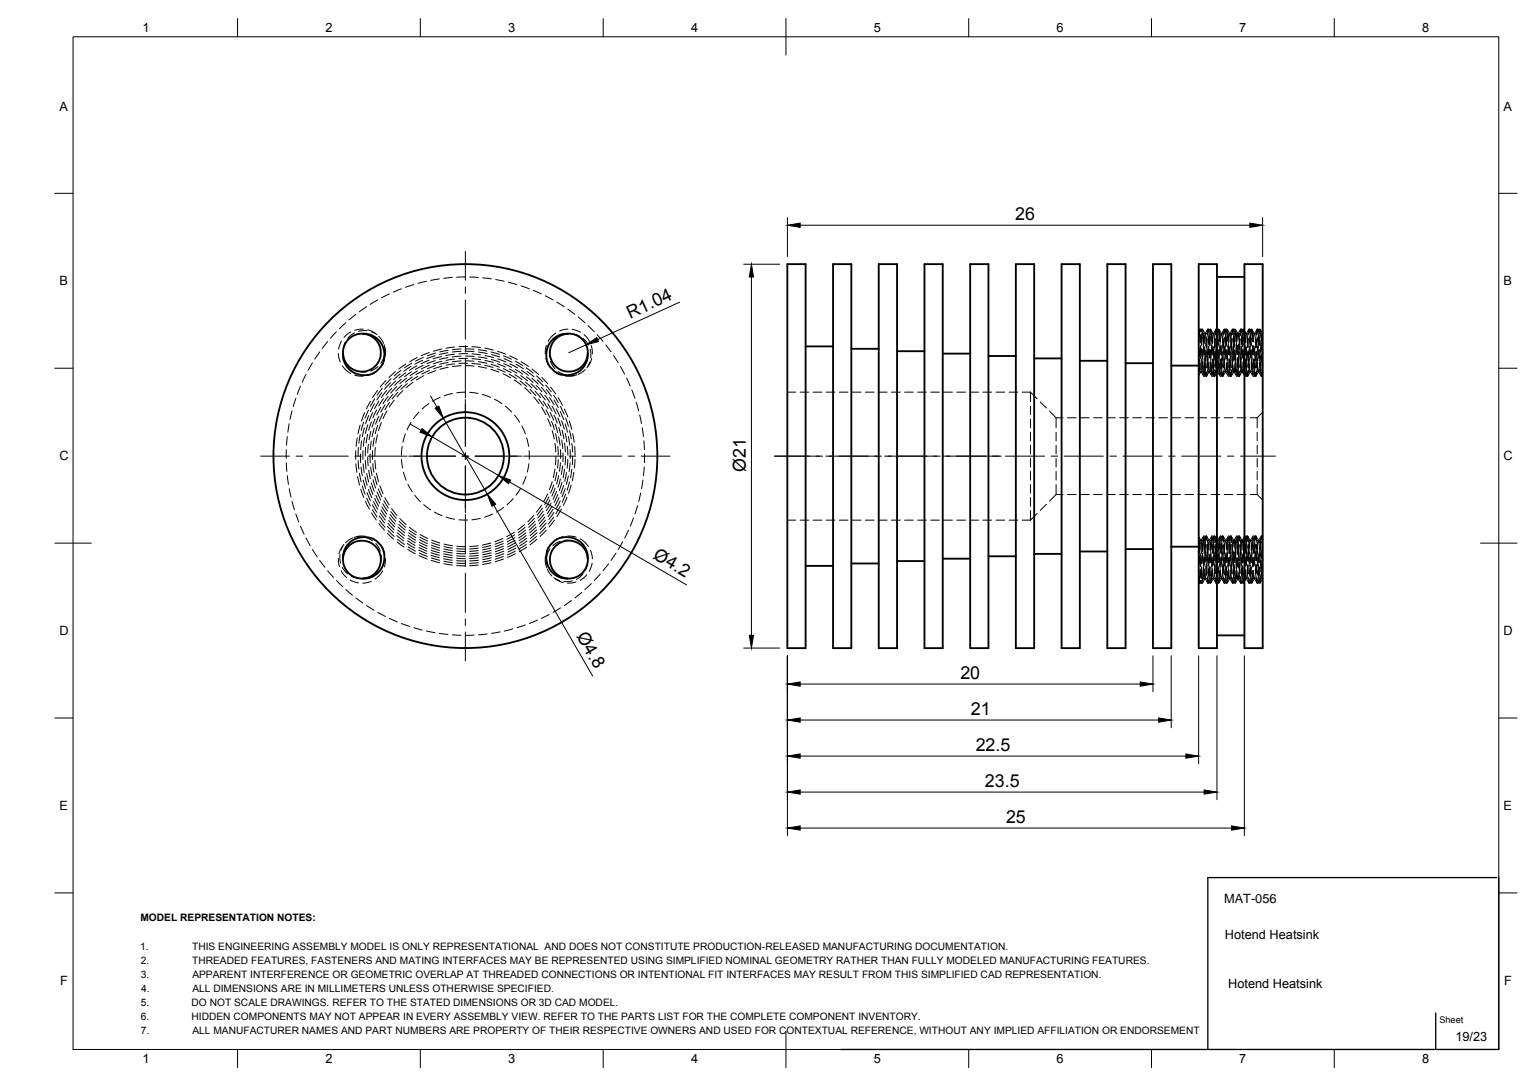
ISO-10303-21;
HEADER;
/* Generated by software containing ST-Developer
 * from STEP Tools, Inc. (www.steptools.com) 
 */

FILE_DESCRIPTION(
/* description */ (''),
/* implementation_level */ '2;1');

FILE_NAME(
/* name */ 'Hotend Heatsink.step',
/* time_stamp */ '2026-10-28T16:47:13+01:00',
/* author */ (''),
/* organization */ (''),
/* preprocessor_version */ 'ST-DEVELOPER v20.2',
/* originating_system */ 'Autodesk Translation Framework v15.17.0.0',
/* authorisation */ '');

FILE_SCHEMA (('AUTOMOTIVE_DESIGN { 1 0 10303 214 3 1 1 }'));
ENDSEC;

DATA;
#10=MECHANICAL_DESIGN_GEOMETRIC_PRESENTATION_REPRESENTATION('',(#4609),#459242);
#4421=SHAPE_REPRESENTATION_RELATIONSHIP('SRR','None',#459348,#4442);
#4442=ADVANCED_BREP_SHAPE_REPRESENTATION('',(#4489),#459237);
#4489=MANIFOLD_SOLID_BREP('E3D V6 heathink',#94667);
#4609=STYLED_ITEM('',(#459519),#4489);
#5105=CONICAL_SURFACE('',#105260,2.25,0.785398163397451);
#5106=CONICAL_SURFACE('',#105276,1.99999999999997,0.785398163397454);
#5230=FACE_BOUND('',#17895,.T.);
#5231=FACE_BOUND('',#17896,.T.);
#5232=FACE_BOUND('',#17897,.T.);
#5233=FACE_BOUND('',#17898,.T.);
#5234=FACE_BOUND('',#17899,.T.);
#5235=FACE_BOUND('',#17904,.T.);
#5236=FACE_BOUND('',#17905,.T.);
#5237=FACE_BOUND('',#17906,.T.);
#5238=FACE_BOUND('',#17907,.T.);
#5239=FACE_BOUND('',#17908,.T.);
#5240=FACE_BOUND('',#17934,.T.);
#5241=FACE_BOUND('',#17936,.T.);
#5242=FACE_BOUND('',#17938,.T.);
#5243=FACE_BOUND('',#17940,.T.);
#5244=FACE_BOUND('',#17942,.T.);
#5245=FACE_BOUND('',#17944,.T.);
#5246=FACE_BOUND('',#17946,.T.);
#5247=FACE_BOUND('',#17948,.T.);
#5248=FACE_BOUND('',#17950,.T.);
#5249=FACE_BOUND('',#17952,.T.);
#5250=FACE_BOUND('',#17954,.T.);
#5251=FACE_BOUND('',#17956,.T.);
#5252=FACE_BOUND('',#17958,.T.);
#5253=FACE_BOUND('',#17960,.T.);
#5254=FACE_BOUND('',#17962,.T.);
#5255=FACE_BOUND('',#17964,.T.);
#5256=FACE_BOUND('',#17966,.T.);
#5257=FACE_BOUND('',#17968,.T.);
#5258=FACE_BOUND('',#17970,.T.);
#5259=FACE_BOUND('',#17972,.T.);
#6106=PLANE('',#105266);
#6107=PLANE('',#105269);
#6108=PLANE('',#105337);
#6109=PLANE('',#105338);
#6110=PLANE('',#105339);
#6111=PLANE('',#105340);
#6112=PLANE('',#105341);
#6113=PLANE('',#105342);
#6114=PLANE('',#105343);
#6115=PLANE('',#105344);
#6116=PLANE('',#105345);
#6117=PLANE('',#105346);
#6118=PLANE('',#105347);
#6119=PLANE('',#105348);
#6120=PLANE('',#105349);
#6121=PLANE('',#105350);
#6122=PLANE('',#105351);
#6123=PLANE('',#105352);
#6124=PLANE('',#105353);
#6125=PLANE('',#105354);
#6126=PLANE('',#105355);
#6127=PLANE('',#105356);
#6337=B_SPLINE_SURFACE_WITH_KNOTS('',3,3,((#452194,#452195,#452196,#452197,
#452198,#452199,#452200,#452201,#452202,#452203,#452204,#452205,#452206,
#452207,#452208,#452209,#452210,#452211,#452212,#452213,#452214,#452215,
#452216,#452217,#452218,#452219,#452220,#452221,#452222,#452223,#452224,
#452225,#452226,#452227,#452228,#452229,#452230,#452231,#452232,#452233,
#452234,#452235,#452236,#452237,#452238,#452239,#452240,#452241,#452242,
#452243,#452244,#452245,#452246,#452247),(#452248,#452249,#452250,#452251,
#452252,#452253,#452254,#452255,#452256,#452257,#452258,#452259,#452260,
#452261,#452262,#452263,#452264,#452265,#452266,#452267,#452268,#452269,
#452270,#452271,#452272,#452273,#452274,#452275,#452276,#452277,#452278,
#452279,#452280,#452281,#452282,#452283,#452284,#452285,#452286,#452287,
#452288,#452289,#452290,#452291,#452292,#452293,#452294,#452295,#452296,
#452297,#452298,#452299,#452300,#452301),(#452302,#452303,#452304,#452305,
#452306,#452307,#452308,#452309,#452310,#452311,#452312,#452313,#452314,
#452315,#452316,#452317,#452318,#452319,#452320,#452321,#452322,#452323,
#452324,#452325,#452326,#452327,#452328,#452329,#452330,#452331,#452332,
#452333,#452334,#452335,#452336,#452337,#452338,#452339,#452340,#452341,
#452342,#452343,#452344,#452345,#452346,#452347,#452348,#452349,#452350,
#452351,#452352,#452353,#452354,#452355),(#452356,#452357,#452358,#452359,
#452360,#452361,#452362,#452363,#452364,#452365,#452366,#452367,#452368,
#452369,#452370,#452371,#452372,#452373,#452374,#452375,#452376,#452377,
#452378,#452379,#452380,#452381,#452382,#452383,#452384,#452385,#452386,
#452387,#452388,#452389,#452390,#452391,#452392,#452393,#452394,#452395,
#452396,#452397,#452398,#452399,#452400,#452401,#452402,#452403,#452404,
#452405,#452406,#452407,#452408,#452409)),.UNSPECIFIED.,.F.,.F.,.F.,(4,
4),(4,1,1,1,1,1,1,1,1,1,1,1,1,1,1,1,1,1,1,1,1,1,1,1,1,1,1,1,1,1,1,1,1,1,
1,1,1,1,1,1,1,1,1,1,1,1,1,1,1,1,1,4),(0.,0.0291273210806165),(11.8408508686654,
12.8389428231049,13.8370347775443,14.8351267319837,15.8332186864231,16.8313106408625,
17.829402595302,18.8274945497414,19.8255865041808,20.8236784586202,21.8217704130596,
22.8198623674991,23.8179543219385,24.8160462763779,25.8141382308173,26.8122301852567,
27.8103221396962,28.8084140941356,29.806506048575,30.8045980030144,31.8026899574538,
32.8007819118933,33.7988738663327,34.7969658207721,35.7950577752115,36.7931497296509,
37.7912416840904,38.7893336385298,39.7874255929692,40.7855175474086,41.783609501848,
42.7817014562875,43.7797934107269,44.7778853651663,45.7759773196057,46.7740692740451,
47.7721612284846,48.770253182924,49.7683451373634,50.7664370918028,51.7645290462422,
52.7626210006817,53.7607129551211,54.7588049095605,55.7568968639999,56.7549888184393,
57.7530807728788,58.7511727273182,59.7492646817576,60.747356636197,61.7454485906364,
62.7435405450759),.UNSPECIFIED.);
#6338=B_SPLINE_SURFACE_WITH_KNOTS('',3,3,((#452514,#452515,#452516,#452517,
#452518,#452519,#452520,#452521,#452522,#452523,#452524,#452525,#452526,
#452527,#452528,#452529,#452530,#452531,#452532,#452533,#452534,#452535,
#452536,#452537,#452538,#452539,#452540,#452541,#452542,#452543,#452544,
#452545,#452546,#452547,#452548,#452549,#452550,#452551,#452552,#452553,
#452554,#452555,#452556,#452557,#452558,#452559,#452560,#452561,#452562,
#452563,#452564,#452565,#452566,#452567),(#452568,#452569,#452570,#452571,
#452572,#452573,#452574,#452575,#452576,#452577,#452578,#452579,#452580,
#452581,#452582,#452583,#452584,#452585,#452586,#452587,#452588,#452589,
#452590,#452591,#452592,#452593,#452594,#452595,#452596,#452597,#452598,
#452599,#452600,#452601,#452602,#452603,#452604,#452605,#452606,#452607,
#452608,#452609,#452610,#452611,#452612,#452613,#452614,#452615,#452616,
#452617,#452618,#452619,#452620,#452621),(#452622,#452623,#452624,#452625,
#452626,#452627,#452628,#452629,#452630,#452631,#452632,#452633,#452634,
#452635,#452636,#452637,#452638,#452639,#452640,#452641,#452642,#452643,
#452644,#452645,#452646,#452647,#452648,#452649,#452650,#452651,#452652,
#452653,#452654,#452655,#452656,#452657,#452658,#452659,#452660,#452661,
#452662,#452663,#452664,#452665,#452666,#452667,#452668,#452669,#452670,
#452671,#452672,#452673,#452674,#452675),(#452676,#452677,#452678,#452679,
#452680,#452681,#452682,#452683,#452684,#452685,#452686,#452687,#452688,
#452689,#452690,#452691,#452692,#452693,#452694,#452695,#452696,#452697,
#452698,#452699,#452700,#452701,#452702,#452703,#452704,#452705,#452706,
#452707,#452708,#452709,#452710,#452711,#452712,#452713,#452714,#452715,
#452716,#452717,#452718,#452719,#452720,#452721,#452722,#452723,#452724,
#452725,#452726,#452727,#452728,#452729)),.UNSPECIFIED.,.F.,.F.,.F.,(4,
4),(4,1,1,1,1,1,1,1,1,1,1,1,1,1,1,1,1,1,1,1,1,1,1,1,1,1,1,1,1,1,1,1,1,1,
1,1,1,1,1,1,1,1,1,1,1,1,1,1,1,1,1,4),(0.,0.0291273210806165),(14.4000123930734,
15.3981043475128,16.3961963019522,17.3942882563917,18.3923802108311,19.3904721652705,
20.3885641197099,21.3866560741493,22.3847480285887,23.3828399830282,24.3809319374676,
25.379023891907,26.3771158463464,27.3752078007858,28.3732997552253,29.3713917096647,
30.3694836641041,31.3675756185435,32.3656675729829,33.3637595274224,34.3618514818618,
35.3599434363012,36.3580353907406,37.35612734518,38.3542192996195,39.3523112540589,
40.3504032084983,41.3484951629377,42.3465871173771,43.3446790718166,44.342771026256,
45.3408629806954,46.3389549351348,47.3370468895742,48.3351388440137,49.3332307984531,
50.3313227528925,51.3294147073319,52.3275066617713,53.3255986162108,54.3236905706502,
55.3217825250896,56.319874479529,57.3179664339684,58.3160583884079,59.3141503428473,
60.3122422972867,61.3103342517261,62.3084262061655,63.306518160605,64.3046101150444,
65.3027020694838),.UNSPECIFIED.);
#6339=B_SPLINE_SURFACE_WITH_KNOTS('',3,3,((#453481,#453482,#453483,#453484,
#453485,#453486,#453487,#453488,#453489,#453490,#453491,#453492,#453493,
#453494,#453495,#453496,#453497,#453498,#453499,#453500,#453501,#453502,
#453503,#453504,#453505,#453506,#453507,#453508,#453509,#453510,#453511,
#453512,#453513,#453514,#453515,#453516,#453517,#453518,#453519,#453520,
#453521,#453522,#453523,#453524,#453525,#453526,#453527,#453528,#453529,
#453530,#453531,#453532,#453533,#453534),(#453535,#453536,#453537,#453538,
#453539,#453540,#453541,#453542,#453543,#453544,#453545,#453546,#453547,
#453548,#453549,#453550,#453551,#453552,#453553,#453554,#453555,#453556,
#453557,#453558,#453559,#453560,#453561,#453562,#453563,#453564,#453565,
#453566,#453567,#453568,#453569,#453570,#453571,#453572,#453573,#453574,
#453575,#453576,#453577,#453578,#453579,#453580,#453581,#453582,#453583,
#453584,#453585,#453586,#453587,#453588),(#453589,#453590,#453591,#453592,
#453593,#453594,#453595,#453596,#453597,#453598,#453599,#453600,#453601,
#453602,#453603,#453604,#453605,#453606,#453607,#453608,#453609,#453610,
#453611,#453612,#453613,#453614,#453615,#453616,#453617,#453618,#453619,
#453620,#453621,#453622,#453623,#453624,#453625,#453626,#453627,#453628,
#453629,#453630,#453631,#453632,#453633,#453634,#453635,#453636,#453637,
#453638,#453639,#453640,#453641,#453642),(#453643,#453644,#453645,#453646,
#453647,#453648,#453649,#453650,#453651,#453652,#453653,#453654,#453655,
#453656,#453657,#453658,#453659,#453660,#453661,#453662,#453663,#453664,
#453665,#453666,#453667,#453668,#453669,#453670,#453671,#453672,#453673,
#453674,#453675,#453676,#453677,#453678,#453679,#453680,#453681,#453682,
#453683,#453684,#453685,#453686,#453687,#453688,#453689,#453690,#453691,
#453692,#453693,#453694,#453695,#453696)),.UNSPECIFIED.,.F.,.F.,.F.,(4,
4),(4,1,1,1,1,1,1,1,1,1,1,1,1,1,1,1,1,1,1,1,1,1,1,1,1,1,1,1,1,1,1,1,1,1,
1,1,1,1,1,1,1,1,1,1,1,1,1,1,1,1,1,4),(0.,0.0291273210806165),(11.8408508686654,
12.8389428231049,13.8370347775443,14.8351267319837,15.8332186864231,16.8313106408625,
17.829402595302,18.8274945497414,19.8255865041808,20.8236784586202,21.8217704130596,
22.8198623674991,23.8179543219385,24.8160462763779,25.8141382308173,26.8122301852567,
27.8103221396962,28.8084140941356,29.806506048575,30.8045980030144,31.8026899574538,
32.8007819118933,33.7988738663327,34.7969658207721,35.7950577752115,36.7931497296509,
37.7912416840904,38.7893336385298,39.7874255929692,40.7855175474086,41.783609501848,
42.7817014562875,43.7797934107269,44.7778853651663,45.7759773196057,46.7740692740451,
47.7721612284846,48.770253182924,49.7683451373634,50.7664370918028,51.7645290462422,
52.7626210006817,53.7607129551211,54.7588049095605,55.7568968639999,56.7549888184393,
57.7530807728788,58.7511727273182,59.7492646817576,60.747356636197,61.7454485906364,
62.7435405450759),.UNSPECIFIED.);
#6340=B_SPLINE_SURFACE_WITH_KNOTS('',3,3,((#453722,#453723,#453724,#453725,
#453726,#453727,#453728,#453729,#453730,#453731,#453732,#453733,#453734,
#453735,#453736,#453737,#453738,#453739,#453740,#453741,#453742,#453743,
#453744,#453745,#453746,#453747,#453748,#453749,#453750,#453751,#453752,
#453753,#453754,#453755,#453756,#453757,#453758,#453759,#453760,#453761,
#453762,#453763,#453764,#453765,#453766,#453767,#453768,#453769,#453770,
#453771,#453772,#453773,#453774,#453775),(#453776,#453777,#453778,#453779,
#453780,#453781,#453782,#453783,#453784,#453785,#453786,#453787,#453788,
#453789,#453790,#453791,#453792,#453793,#453794,#453795,#453796,#453797,
#453798,#453799,#453800,#453801,#453802,#453803,#453804,#453805,#453806,
#453807,#453808,#453809,#453810,#453811,#453812,#453813,#453814,#453815,
#453816,#453817,#453818,#453819,#453820,#453821,#453822,#453823,#453824,
#453825,#453826,#453827,#453828,#453829),(#453830,#453831,#453832,#453833,
#453834,#453835,#453836,#453837,#453838,#453839,#453840,#453841,#453842,
#453843,#453844,#453845,#453846,#453847,#453848,#453849,#453850,#453851,
#453852,#453853,#453854,#453855,#453856,#453857,#453858,#453859,#453860,
#453861,#453862,#453863,#453864,#453865,#453866,#453867,#453868,#453869,
#453870,#453871,#453872,#453873,#453874,#453875,#453876,#453877,#453878,
#453879,#453880,#453881,#453882,#453883),(#453884,#453885,#453886,#453887,
#453888,#453889,#453890,#453891,#453892,#453893,#453894,#453895,#453896,
#453897,#453898,#453899,#453900,#453901,#453902,#453903,#453904,#453905,
#453906,#453907,#453908,#453909,#453910,#453911,#453912,#453913,#453914,
#453915,#453916,#453917,#453918,#453919,#453920,#453921,#453922,#453923,
#453924,#453925,#453926,#453927,#453928,#453929,#453930,#453931,#453932,
#453933,#453934,#453935,#453936,#453937)),.UNSPECIFIED.,.F.,.F.,.F.,(4,
4),(4,1,1,1,1,1,1,1,1,1,1,1,1,1,1,1,1,1,1,1,1,1,1,1,1,1,1,1,1,1,1,1,1,1,
1,1,1,1,1,1,1,1,1,1,1,1,1,1,1,1,1,4),(0.,0.0291273210806165),(14.4000123930734,
15.3981043475128,16.3961963019522,17.3942882563917,18.3923802108311,19.3904721652705,
20.3885641197099,21.3866560741493,22.3847480285887,23.3828399830282,24.3809319374676,
25.379023891907,26.3771158463464,27.3752078007858,28.3732997552253,29.3713917096647,
30.3694836641041,31.3675756185435,32.3656675729829,33.3637595274224,34.3618514818618,
35.3599434363012,36.3580353907406,37.35612734518,38.3542192996195,39.3523112540589,
40.3504032084983,41.3484951629377,42.3465871173771,43.3446790718166,44.342771026256,
45.3408629806954,46.3389549351348,47.3370468895742,48.3351388440137,49.3332307984531,
50.3313227528925,51.3294147073319,52.3275066617713,53.3255986162108,54.3236905706502,
55.3217825250896,56.319874479529,57.3179664339684,58.3160583884079,59.3141503428473,
60.3122422972867,61.3103342517261,62.3084262061655,63.306518160605,64.3046101150444,
65.3027020694838),.UNSPECIFIED.);
#6341=B_SPLINE_SURFACE_WITH_KNOTS('',3,3,((#453983,#453984,#453985,#453986,
#453987,#453988,#453989,#453990,#453991,#453992,#453993,#453994,#453995,
#453996,#453997,#453998,#453999,#454000,#454001,#454002,#454003,#454004,
#454005,#454006,#454007,#454008,#454009,#454010,#454011,#454012,#454013,
#454014,#454015,#454016,#454017,#454018,#454019,#454020,#454021,#454022,
#454023,#454024,#454025,#454026,#454027,#454028,#454029,#454030,#454031,
#454032,#454033,#454034,#454035,#454036),(#454037,#454038,#454039,#454040,
#454041,#454042,#454043,#454044,#454045,#454046,#454047,#454048,#454049,
#454050,#454051,#454052,#454053,#454054,#454055,#454056,#454057,#454058,
#454059,#454060,#454061,#454062,#454063,#454064,#454065,#454066,#454067,
#454068,#454069,#454070,#454071,#454072,#454073,#454074,#454075,#454076,
#454077,#454078,#454079,#454080,#454081,#454082,#454083,#454084,#454085,
#454086,#454087,#454088,#454089,#454090),(#454091,#454092,#454093,#454094,
#454095,#454096,#454097,#454098,#454099,#454100,#454101,#454102,#454103,
#454104,#454105,#454106,#454107,#454108,#454109,#454110,#454111,#454112,
#454113,#454114,#454115,#454116,#454117,#454118,#454119,#454120,#454121,
#454122,#454123,#454124,#454125,#454126,#454127,#454128,#454129,#454130,
#454131,#454132,#454133,#454134,#454135,#454136,#454137,#454138,#454139,
#454140,#454141,#454142,#454143,#454144),(#454145,#454146,#454147,#454148,
#454149,#454150,#454151,#454152,#454153,#454154,#454155,#454156,#454157,
#454158,#454159,#454160,#454161,#454162,#454163,#454164,#454165,#454166,
#454167,#454168,#454169,#454170,#454171,#454172,#454173,#454174,#454175,
#454176,#454177,#454178,#454179,#454180,#454181,#454182,#454183,#454184,
#454185,#454186,#454187,#454188,#454189,#454190,#454191,#454192,#454193,
#454194,#454195,#454196,#454197,#454198)),.UNSPECIFIED.,.F.,.F.,.F.,(4,
4),(4,1,1,1,1,1,1,1,1,1,1,1,1,1,1,1,1,1,1,1,1,1,1,1,1,1,1,1,1,1,1,1,1,1,
1,1,1,1,1,1,1,1,1,1,1,1,1,1,1,1,1,4),(0.,0.0291273210806165),(11.8408508686654,
12.8389428231049,13.8370347775443,14.8351267319837,15.8332186864231,16.8313106408625,
17.829402595302,18.8274945497414,19.8255865041808,20.8236784586202,21.8217704130596,
22.8198623674991,23.8179543219385,24.8160462763779,25.8141382308173,26.8122301852567,
27.8103221396962,28.8084140941356,29.806506048575,30.8045980030144,31.8026899574538,
32.8007819118933,33.7988738663327,34.7969658207721,35.7950577752115,36.7931497296509,
37.7912416840904,38.7893336385298,39.7874255929692,40.7855175474086,41.783609501848,
42.7817014562875,43.7797934107269,44.7778853651663,45.7759773196057,46.7740692740451,
47.7721612284846,48.770253182924,49.7683451373634,50.7664370918028,51.7645290462422,
52.7626210006817,53.7607129551211,54.7588049095605,55.7568968639999,56.7549888184393,
57.7530807728788,58.7511727273182,59.7492646817576,60.747356636197,61.7454485906364,
62.7435405450759),.UNSPECIFIED.);
#6342=B_SPLINE_SURFACE_WITH_KNOTS('',3,3,((#454224,#454225,#454226,#454227,
#454228,#454229,#454230,#454231,#454232,#454233,#454234,#454235,#454236,
#454237,#454238,#454239,#454240,#454241,#454242,#454243,#454244,#454245,
#454246,#454247,#454248,#454249,#454250,#454251,#454252,#454253,#454254,
#454255,#454256,#454257,#454258,#454259,#454260,#454261,#454262,#454263,
#454264,#454265,#454266,#454267,#454268,#454269,#454270,#454271,#454272,
#454273,#454274,#454275,#454276,#454277),(#454278,#454279,#454280,#454281,
#454282,#454283,#454284,#454285,#454286,#454287,#454288,#454289,#454290,
#454291,#454292,#454293,#454294,#454295,#454296,#454297,#454298,#454299,
#454300,#454301,#454302,#454303,#454304,#454305,#454306,#454307,#454308,
#454309,#454310,#454311,#454312,#454313,#454314,#454315,#454316,#454317,
#454318,#454319,#454320,#454321,#454322,#454323,#454324,#454325,#454326,
#454327,#454328,#454329,#454330,#454331),(#454332,#454333,#454334,#454335,
#454336,#454337,#454338,#454339,#454340,#454341,#454342,#454343,#454344,
#454345,#454346,#454347,#454348,#454349,#454350,#454351,#454352,#454353,
#454354,#454355,#454356,#454357,#454358,#454359,#454360,#454361,#454362,
#454363,#454364,#454365,#454366,#454367,#454368,#454369,#454370,#454371,
#454372,#454373,#454374,#454375,#454376,#454377,#454378,#454379,#454380,
#454381,#454382,#454383,#454384,#454385),(#454386,#454387,#454388,#454389,
#454390,#454391,#454392,#454393,#454394,#454395,#454396,#454397,#454398,
#454399,#454400,#454401,#454402,#454403,#454404,#454405,#454406,#454407,
#454408,#454409,#454410,#454411,#454412,#454413,#454414,#454415,#454416,
#454417,#454418,#454419,#454420,#454421,#454422,#454423,#454424,#454425,
#454426,#454427,#454428,#454429,#454430,#454431,#454432,#454433,#454434,
#454435,#454436,#454437,#454438,#454439)),.UNSPECIFIED.,.F.,.F.,.F.,(4,
4),(4,1,1,1,1,1,1,1,1,1,1,1,1,1,1,1,1,1,1,1,1,1,1,1,1,1,1,1,1,1,1,1,1,1,
1,1,1,1,1,1,1,1,1,1,1,1,1,1,1,1,1,4),(0.,0.0291273210806165),(14.4000123930734,
15.3981043475128,16.3961963019522,17.3942882563917,18.3923802108311,19.3904721652705,
20.3885641197099,21.3866560741493,22.3847480285887,23.3828399830282,24.3809319374676,
25.379023891907,26.3771158463464,27.3752078007858,28.3732997552253,29.3713917096647,
30.3694836641041,31.3675756185435,32.3656675729829,33.3637595274224,34.3618514818618,
35.3599434363012,36.3580353907406,37.35612734518,38.3542192996195,39.3523112540589,
40.3504032084983,41.3484951629377,42.3465871173771,43.3446790718166,44.342771026256,
45.3408629806954,46.3389549351348,47.3370468895742,48.3351388440137,49.3332307984531,
50.3313227528925,51.3294147073319,52.3275066617713,53.3255986162108,54.3236905706502,
55.3217825250896,56.319874479529,57.3179664339684,58.3160583884079,59.3141503428473,
60.3122422972867,61.3103342517261,62.3084262061655,63.306518160605,64.3046101150444,
65.3027020694838),.UNSPECIFIED.);
#6343=B_SPLINE_SURFACE_WITH_KNOTS('',3,3,((#454485,#454486,#454487,#454488,
#454489,#454490,#454491,#454492,#454493,#454494,#454495,#454496,#454497,
#454498,#454499,#454500,#454501,#454502,#454503,#454504,#454505,#454506,
#454507,#454508,#454509,#454510,#454511,#454512,#454513,#454514,#454515,
#454516,#454517,#454518,#454519,#454520,#454521,#454522,#454523,#454524,
#454525,#454526,#454527,#454528,#454529,#454530,#454531,#454532,#454533,
#454534,#454535,#454536,#454537,#454538),(#454539,#454540,#454541,#454542,
#454543,#454544,#454545,#454546,#454547,#454548,#454549,#454550,#454551,
#454552,#454553,#454554,#454555,#454556,#454557,#454558,#454559,#454560,
#454561,#454562,#454563,#454564,#454565,#454566,#454567,#454568,#454569,
#454570,#454571,#454572,#454573,#454574,#454575,#454576,#454577,#454578,
#454579,#454580,#454581,#454582,#454583,#454584,#454585,#454586,#454587,
#454588,#454589,#454590,#454591,#454592),(#454593,#454594,#454595,#454596,
#454597,#454598,#454599,#454600,#454601,#454602,#454603,#454604,#454605,
#454606,#454607,#454608,#454609,#454610,#454611,#454612,#454613,#454614,
#454615,#454616,#454617,#454618,#454619,#454620,#454621,#454622,#454623,
#454624,#454625,#454626,#454627,#454628,#454629,#454630,#454631,#454632,
#454633,#454634,#454635,#454636,#454637,#454638,#454639,#454640,#454641,
#454642,#454643,#454644,#454645,#454646),(#454647,#454648,#454649,#454650,
#454651,#454652,#454653,#454654,#454655,#454656,#454657,#454658,#454659,
#454660,#454661,#454662,#454663,#454664,#454665,#454666,#454667,#454668,
#454669,#454670,#454671,#454672,#454673,#454674,#454675,#454676,#454677,
#454678,#454679,#454680,#454681,#454682,#454683,#454684,#454685,#454686,
#454687,#454688,#454689,#454690,#454691,#454692,#454693,#454694,#454695,
#454696,#454697,#454698,#454699,#454700)),.UNSPECIFIED.,.F.,.F.,.F.,(4,
4),(4,1,1,1,1,1,1,1,1,1,1,1,1,1,1,1,1,1,1,1,1,1,1,1,1,1,1,1,1,1,1,1,1,1,
1,1,1,1,1,1,1,1,1,1,1,1,1,1,1,1,1,4),(0.,0.0291273210806165),(11.8408508686654,
12.8389428231049,13.8370347775443,14.8351267319837,15.8332186864231,16.8313106408625,
17.829402595302,18.8274945497414,19.8255865041808,20.8236784586202,21.8217704130596,
22.8198623674991,23.8179543219385,24.8160462763779,25.8141382308173,26.8122301852567,
27.8103221396962,28.8084140941356,29.806506048575,30.8045980030144,31.8026899574538,
32.8007819118933,33.7988738663327,34.7969658207721,35.7950577752115,36.7931497296509,
37.7912416840904,38.7893336385298,39.7874255929692,40.7855175474086,41.783609501848,
42.7817014562875,43.7797934107269,44.7778853651663,45.7759773196057,46.7740692740451,
47.7721612284846,48.770253182924,49.7683451373634,50.7664370918028,51.7645290462422,
52.7626210006817,53.7607129551211,54.7588049095605,55.7568968639999,56.7549888184393,
57.7530807728788,58.7511727273182,59.7492646817576,60.747356636197,61.7454485906364,
62.7435405450759),.UNSPECIFIED.);
#6344=B_SPLINE_SURFACE_WITH_KNOTS('',3,3,((#454726,#454727,#454728,#454729,
#454730,#454731,#454732,#454733,#454734,#454735,#454736,#454737,#454738,
#454739,#454740,#454741,#454742,#454743,#454744,#454745,#454746,#454747,
#454748,#454749,#454750,#454751,#454752,#454753,#454754,#454755,#454756,
#454757,#454758,#454759,#454760,#454761,#454762,#454763,#454764,#454765,
#454766,#454767,#454768,#454769,#454770,#454771,#454772,#454773,#454774,
#454775,#454776,#454777,#454778,#454779),(#454780,#454781,#454782,#454783,
#454784,#454785,#454786,#454787,#454788,#454789,#454790,#454791,#454792,
#454793,#454794,#454795,#454796,#454797,#454798,#454799,#454800,#454801,
#454802,#454803,#454804,#454805,#454806,#454807,#454808,#454809,#454810,
#454811,#454812,#454813,#454814,#454815,#454816,#454817,#454818,#454819,
#454820,#454821,#454822,#454823,#454824,#454825,#454826,#454827,#454828,
#454829,#454830,#454831,#454832,#454833),(#454834,#454835,#454836,#454837,
#454838,#454839,#454840,#454841,#454842,#454843,#454844,#454845,#454846,
#454847,#454848,#454849,#454850,#454851,#454852,#454853,#454854,#454855,
#454856,#454857,#454858,#454859,#454860,#454861,#454862,#454863,#454864,
#454865,#454866,#454867,#454868,#454869,#454870,#454871,#454872,#454873,
#454874,#454875,#454876,#454877,#454878,#454879,#454880,#454881,#454882,
#454883,#454884,#454885,#454886,#454887),(#454888,#454889,#454890,#454891,
#454892,#454893,#454894,#454895,#454896,#454897,#454898,#454899,#454900,
#454901,#454902,#454903,#454904,#454905,#454906,#454907,#454908,#454909,
#454910,#454911,#454912,#454913,#454914,#454915,#454916,#454917,#454918,
#454919,#454920,#454921,#454922,#454923,#454924,#454925,#454926,#454927,
#454928,#454929,#454930,#454931,#454932,#454933,#454934,#454935,#454936,
#454937,#454938,#454939,#454940,#454941)),.UNSPECIFIED.,.F.,.F.,.F.,(4,
4),(4,1,1,1,1,1,1,1,1,1,1,1,1,1,1,1,1,1,1,1,1,1,1,1,1,1,1,1,1,1,1,1,1,1,
1,1,1,1,1,1,1,1,1,1,1,1,1,1,1,1,1,4),(0.,0.0291273210806165),(14.4000123930734,
15.3981043475128,16.3961963019522,17.3942882563917,18.3923802108311,19.3904721652705,
20.3885641197099,21.3866560741493,22.3847480285887,23.3828399830282,24.3809319374676,
25.379023891907,26.3771158463464,27.3752078007858,28.3732997552253,29.3713917096647,
30.3694836641041,31.3675756185435,32.3656675729829,33.3637595274224,34.3618514818618,
35.3599434363012,36.3580353907406,37.35612734518,38.3542192996195,39.3523112540589,
40.3504032084983,41.3484951629377,42.3465871173771,43.3446790718166,44.342771026256,
45.3408629806954,46.3389549351348,47.3370468895742,48.3351388440137,49.3332307984531,
50.3313227528925,51.3294147073319,52.3275066617713,53.3255986162108,54.3236905706502,
55.3217825250896,56.319874479529,57.3179664339684,58.3160583884079,59.3141503428473,
60.3122422972867,61.3103342517261,62.3084262061655,63.306518160605,64.3046101150444,
65.3027020694838),.UNSPECIFIED.);
#11903=FACE_OUTER_BOUND('',#17828,.T.);
#11904=FACE_OUTER_BOUND('',#17829,.T.);
#11905=FACE_OUTER_BOUND('',#17830,.T.);
#11906=FACE_OUTER_BOUND('',#17831,.T.);
#11907=FACE_OUTER_BOUND('',#17832,.T.);
#11908=FACE_OUTER_BOUND('',#17833,.T.);
#11909=FACE_OUTER_BOUND('',#17834,.T.);
#11910=FACE_OUTER_BOUND('',#17835,.T.);
#11911=FACE_OUTER_BOUND('',#17836,.T.);
#11912=FACE_OUTER_BOUND('',#17837,.T.);
#11913=FACE_OUTER_BOUND('',#17838,.T.);
#11914=FACE_OUTER_BOUND('',#17839,.T.);
#11915=FACE_OUTER_BOUND('',#17840,.T.);
#11916=FACE_OUTER_BOUND('',#17841,.T.);
#11917=FACE_OUTER_BOUND('',#17842,.T.);
#11918=FACE_OUTER_BOUND('',#17843,.T.);
#11919=FACE_OUTER_BOUND('',#17844,.T.);
#11920=FACE_OUTER_BOUND('',#17845,.T.);
#11921=FACE_OUTER_BOUND('',#17846,.T.);
#11922=FACE_OUTER_BOUND('',#17847,.T.);
#11923=FACE_OUTER_BOUND('',#17848,.T.);
#11924=FACE_OUTER_BOUND('',#17849,.T.);
#11925=FACE_OUTER_BOUND('',#17850,.T.);
#11926=FACE_OUTER_BOUND('',#17851,.T.);
#11927=FACE_OUTER_BOUND('',#17852,.T.);
#11928=FACE_OUTER_BOUND('',#17853,.T.);
#11929=FACE_OUTER_BOUND('',#17854,.T.);
#11930=FACE_OUTER_BOUND('',#17855,.T.);
#11931=FACE_OUTER_BOUND('',#17856,.T.);
#11932=FACE_OUTER_BOUND('',#17857,.T.);
#11933=FACE_OUTER_BOUND('',#17858,.T.);
#11934=FACE_OUTER_BOUND('',#17859,.T.);
#11935=FACE_OUTER_BOUND('',#17860,.T.);
#11936=FACE_OUTER_BOUND('',#17861,.T.);
#11937=FACE_OUTER_BOUND('',#17862,.T.);
#11938=FACE_OUTER_BOUND('',#17863,.T.);
#11939=FACE_OUTER_BOUND('',#17864,.T.);
#11940=FACE_OUTER_BOUND('',#17865,.T.);
#11941=FACE_OUTER_BOUND('',#17866,.T.);
#11942=FACE_OUTER_BOUND('',#17867,.T.);
#11943=FACE_OUTER_BOUND('',#17868,.T.);
#11944=FACE_OUTER_BOUND('',#17869,.T.);
#11945=FACE_OUTER_BOUND('',#17870,.T.);
#11946=FACE_OUTER_BOUND('',#17871,.T.);
#11947=FACE_OUTER_BOUND('',#17872,.T.);
#11948=FACE_OUTER_BOUND('',#17873,.T.);
#11949=FACE_OUTER_BOUND('',#17874,.T.);
#11950=FACE_OUTER_BOUND('',#17875,.T.);
#11951=FACE_OUTER_BOUND('',#17876,.T.);
#11952=FACE_OUTER_BOUND('',#17877,.T.);
#11953=FACE_OUTER_BOUND('',#17878,.T.);
#11954=FACE_OUTER_BOUND('',#17879,.T.);
#11955=FACE_OUTER_BOUND('',#17880,.T.);
#11956=FACE_OUTER_BOUND('',#17881,.T.);
#11957=FACE_OUTER_BOUND('',#17882,.T.);
#11958=FACE_OUTER_BOUND('',#17883,.T.);
#11959=FACE_OUTER_BOUND('',#17884,.T.);
#11960=FACE_OUTER_BOUND('',#17885,.T.);
#11961=FACE_OUTER_BOUND('',#17886,.T.);
#11962=FACE_OUTER_BOUND('',#17887,.T.);
#11963=FACE_OUTER_BOUND('',#17888,.T.);
#11964=FACE_OUTER_BOUND('',#17889,.T.);
#11965=FACE_OUTER_BOUND('',#17890,.T.);
#11966=FACE_OUTER_BOUND('',#17891,.T.);
#11967=FACE_OUTER_BOUND('',#17892,.T.);
#11968=FACE_OUTER_BOUND('',#17893,.T.);
#11969=FACE_OUTER_BOUND('',#17894,.T.);
#11970=FACE_OUTER_BOUND('',#17900,.T.);
#11971=FACE_OUTER_BOUND('',#17901,.T.);
#11972=FACE_OUTER_BOUND('',#17902,.T.);
#11973=FACE_OUTER_BOUND('',#17903,.T.);
#11974=FACE_OUTER_BOUND('',#17909,.T.);
#11975=FACE_OUTER_BOUND('',#17910,.T.);
#11976=FACE_OUTER_BOUND('',#17911,.T.);
#11977=FACE_OUTER_BOUND('',#17912,.T.);
#11978=FACE_OUTER_BOUND('',#17913,.T.);
#11979=FACE_OUTER_BOUND('',#17914,.T.);
#11980=FACE_OUTER_BOUND('',#17915,.T.);
#11981=FACE_OUTER_BOUND('',#17916,.T.);
#11982=FACE_OUTER_BOUND('',#17917,.T.);
#11983=FACE_OUTER_BOUND('',#17918,.T.);
#11984=FACE_OUTER_BOUND('',#17919,.T.);
#11985=FACE_OUTER_BOUND('',#17920,.T.);
#11986=FACE_OUTER_BOUND('',#17921,.T.);
#11987=FACE_OUTER_BOUND('',#17922,.T.);
#11988=FACE_OUTER_BOUND('',#17923,.T.);
#11989=FACE_OUTER_BOUND('',#17924,.T.);
#11990=FACE_OUTER_BOUND('',#17925,.T.);
#11991=FACE_OUTER_BOUND('',#17926,.T.);
#11992=FACE_OUTER_BOUND('',#17927,.T.);
#11993=FACE_OUTER_BOUND('',#17928,.T.);
#11994=FACE_OUTER_BOUND('',#17929,.T.);
#11995=FACE_OUTER_BOUND('',#17930,.T.);
#11996=FACE_OUTER_BOUND('',#17931,.T.);
#11997=FACE_OUTER_BOUND('',#17932,.T.);
#11998=FACE_OUTER_BOUND('',#17933,.T.);
#11999=FACE_OUTER_BOUND('',#17935,.T.);
#12000=FACE_OUTER_BOUND('',#17937,.T.);
#12001=FACE_OUTER_BOUND('',#17939,.T.);
#12002=FACE_OUTER_BOUND('',#17941,.T.);
#12003=FACE_OUTER_BOUND('',#17943,.T.);
#12004=FACE_OUTER_BOUND('',#17945,.T.);
#12005=FACE_OUTER_BOUND('',#17947,.T.);
#12006=FACE_OUTER_BOUND('',#17949,.T.);
#12007=FACE_OUTER_BOUND('',#17951,.T.);
#12008=FACE_OUTER_BOUND('',#17953,.T.);
#12009=FACE_OUTER_BOUND('',#17955,.T.);
#12010=FACE_OUTER_BOUND('',#17957,.T.);
#12011=FACE_OUTER_BOUND('',#17959,.T.);
#12012=FACE_OUTER_BOUND('',#17961,.T.);
#12013=FACE_OUTER_BOUND('',#17963,.T.);
#12014=FACE_OUTER_BOUND('',#17965,.T.);
#12015=FACE_OUTER_BOUND('',#17967,.T.);
#12016=FACE_OUTER_BOUND('',#17969,.T.);
#12017=FACE_OUTER_BOUND('',#17971,.T.);
#12018=FACE_OUTER_BOUND('',#17973,.T.);
#12019=FACE_OUTER_BOUND('',#17974,.T.);
#12020=FACE_OUTER_BOUND('',#17975,.T.);
#12021=FACE_OUTER_BOUND('',#17976,.T.);
#12022=FACE_OUTER_BOUND('',#17977,.T.);
#12023=FACE_OUTER_BOUND('',#17978,.T.);
#12024=FACE_OUTER_BOUND('',#17979,.T.);
#12025=FACE_OUTER_BOUND('',#17980,.T.);
#12026=FACE_OUTER_BOUND('',#17981,.T.);
#12027=FACE_OUTER_BOUND('',#17982,.T.);
#12028=FACE_OUTER_BOUND('',#17983,.T.);
#12029=FACE_OUTER_BOUND('',#17984,.T.);
#17828=EDGE_LOOP('',(#85802,#85803,#85804));
#17829=EDGE_LOOP('',(#85805,#85806,#85807,#85808,#85809));
#17830=EDGE_LOOP('',(#85810,#85811,#85812,#85813));
#17831=EDGE_LOOP('',(#85814,#85815,#85816,#85817));
#17832=EDGE_LOOP('',(#85818,#85819,#85820,#85821));
#17833=EDGE_LOOP('',(#85822,#85823,#85824,#85825));
#17834=EDGE_LOOP('',(#85826,#85827,#85828,#85829));
#17835=EDGE_LOOP('',(#85830,#85831,#85832,#85833));
#17836=EDGE_LOOP('',(#85834,#85835,#85836,#85837));
#17837=EDGE_LOOP('',(#85838,#85839,#85840,#85841));
#17838=EDGE_LOOP('',(#85842,#85843,#85844,#85845));
#17839=EDGE_LOOP('',(#85846,#85847,#85848,#85849));
#17840=EDGE_LOOP('',(#85850,#85851,#85852,#85853));
#17841=EDGE_LOOP('',(#85854,#85855,#85856,#85857));
#17842=EDGE_LOOP('',(#85858,#85859,#85860,#85861));
#17843=EDGE_LOOP('',(#85862,#85863,#85864,#85865));
#17844=EDGE_LOOP('',(#85866,#85867,#85868));
#17845=EDGE_LOOP('',(#85869,#85870,#85871,#85872,#85873));
#17846=EDGE_LOOP('',(#85874,#85875,#85876,#85877));
#17847=EDGE_LOOP('',(#85878,#85879,#85880,#85881));
#17848=EDGE_LOOP('',(#85882,#85883,#85884,#85885));
#17849=EDGE_LOOP('',(#85886,#85887,#85888,#85889));
#17850=EDGE_LOOP('',(#85890,#85891,#85892,#85893));
#17851=EDGE_LOOP('',(#85894,#85895,#85896,#85897));
#17852=EDGE_LOOP('',(#85898,#85899,#85900,#85901));
#17853=EDGE_LOOP('',(#85902,#85903,#85904,#85905));
#17854=EDGE_LOOP('',(#85906,#85907,#85908,#85909));
#17855=EDGE_LOOP('',(#85910,#85911,#85912,#85913));
#17856=EDGE_LOOP('',(#85914,#85915,#85916,#85917));
#17857=EDGE_LOOP('',(#85918,#85919,#85920,#85921));
#17858=EDGE_LOOP('',(#85922,#85923,#85924,#85925));
#17859=EDGE_LOOP('',(#85926,#85927,#85928,#85929));
#17860=EDGE_LOOP('',(#85930,#85931,#85932));
#17861=EDGE_LOOP('',(#85933,#85934,#85935,#85936,#85937));
#17862=EDGE_LOOP('',(#85938,#85939,#85940,#85941));
#17863=EDGE_LOOP('',(#85942,#85943,#85944,#85945));
#17864=EDGE_LOOP('',(#85946,#85947,#85948,#85949));
#17865=EDGE_LOOP('',(#85950,#85951,#85952,#85953));
#17866=EDGE_LOOP('',(#85954,#85955,#85956,#85957));
#17867=EDGE_LOOP('',(#85958,#85959,#85960,#85961));
#17868=EDGE_LOOP('',(#85962,#85963,#85964,#85965));
#17869=EDGE_LOOP('',(#85966,#85967,#85968,#85969));
#17870=EDGE_LOOP('',(#85970,#85971,#85972,#85973));
#17871=EDGE_LOOP('',(#85974,#85975,#85976,#85977));
#17872=EDGE_LOOP('',(#85978,#85979,#85980,#85981));
#17873=EDGE_LOOP('',(#85982,#85983,#85984,#85985));
#17874=EDGE_LOOP('',(#85986,#85987,#85988,#85989));
#17875=EDGE_LOOP('',(#85990,#85991,#85992,#85993));
#17876=EDGE_LOOP('',(#85994,#85995,#85996));
#17877=EDGE_LOOP('',(#85997,#85998,#85999,#86000,#86001));
#17878=EDGE_LOOP('',(#86002,#86003,#86004,#86005));
#17879=EDGE_LOOP('',(#86006,#86007,#86008,#86009));
#17880=EDGE_LOOP('',(#86010,#86011,#86012,#86013));
#17881=EDGE_LOOP('',(#86014,#86015,#86016,#86017));
#17882=EDGE_LOOP('',(#86018,#86019,#86020,#86021));
#17883=EDGE_LOOP('',(#86022,#86023,#86024,#86025));
#17884=EDGE_LOOP('',(#86026,#86027,#86028,#86029));
#17885=EDGE_LOOP('',(#86030,#86031,#86032,#86033));
#17886=EDGE_LOOP('',(#86034,#86035,#86036,#86037));
#17887=EDGE_LOOP('',(#86038,#86039,#86040,#86041));
#17888=EDGE_LOOP('',(#86042,#86043,#86044,#86045));
#17889=EDGE_LOOP('',(#86046,#86047,#86048,#86049));
#17890=EDGE_LOOP('',(#86050,#86051,#86052,#86053));
#17891=EDGE_LOOP('',(#86054,#86055,#86056,#86057));
#17892=EDGE_LOOP('',(#86058,#86059,#86060,#86061));
#17893=EDGE_LOOP('',(#86062,#86063,#86064,#86065,#86066));
#17894=EDGE_LOOP('',(#86067));
#17895=EDGE_LOOP('',(#86068,#86069,#86070,#86071));
#17896=EDGE_LOOP('',(#86072,#86073,#86074,#86075));
#17897=EDGE_LOOP('',(#86076,#86077,#86078,#86079));
#17898=EDGE_LOOP('',(#86080,#86081,#86082,#86083));
#17899=EDGE_LOOP('',(#86084));
#17900=EDGE_LOOP('',(#86085,#86086,#86087,#86088));
#17901=EDGE_LOOP('',(#86089,#86090,#86091,#86092,#86093,#86094,#86095,#86096,
#86097,#86098,#86099,#86100,#86101,#86102,#86103,#86104,#86105,#86106,#86107,
#86108));
#17902=EDGE_LOOP('',(#86109,#86110,#86111,#86112,#86113,#86114,#86115,#86116,
#86117,#86118,#86119,#86120,#86121,#86122,#86123,#86124,#86125,#86126,#86127));
#17903=EDGE_LOOP('',(#86128));
#17904=EDGE_LOOP('',(#86129,#86130,#86131,#86132,#86133));
#17905=EDGE_LOOP('',(#86134,#86135,#86136,#86137,#86138));
#17906=EDGE_LOOP('',(#86139,#86140,#86141,#86142,#86143));
#17907=EDGE_LOOP('',(#86144));
#17908=EDGE_LOOP('',(#86145,#86146,#86147,#86148,#86149));
#17909=EDGE_LOOP('',(#86150,#86151,#86152,#86153));
#17910=EDGE_LOOP('',(#86154,#86155,#86156,#86157));
#17911=EDGE_LOOP('',(#86158,#86159,#86160,#86161,#86162));
#17912=EDGE_LOOP('',(#86163,#86164,#86165,#86166));
#17913=EDGE_LOOP('',(#86167,#86168,#86169,#86170));
#17914=EDGE_LOOP('',(#86171,#86172,#86173,#86174));
#17915=EDGE_LOOP('',(#86175,#86176,#86177,#86178));
#17916=EDGE_LOOP('',(#86179,#86180,#86181,#86182));
#17917=EDGE_LOOP('',(#86183,#86184,#86185,#86186));
#17918=EDGE_LOOP('',(#86187,#86188,#86189,#86190));
#17919=EDGE_LOOP('',(#86191,#86192,#86193,#86194));
#17920=EDGE_LOOP('',(#86195,#86196,#86197,#86198));
#17921=EDGE_LOOP('',(#86199,#86200,#86201,#86202));
#17922=EDGE_LOOP('',(#86203,#86204,#86205,#86206));
#17923=EDGE_LOOP('',(#86207,#86208,#86209,#86210));
#17924=EDGE_LOOP('',(#86211,#86212,#86213,#86214));
#17925=EDGE_LOOP('',(#86215,#86216,#86217,#86218));
#17926=EDGE_LOOP('',(#86219,#86220,#86221,#86222));
#17927=EDGE_LOOP('',(#86223,#86224,#86225,#86226));
#17928=EDGE_LOOP('',(#86227,#86228,#86229,#86230));
#17929=EDGE_LOOP('',(#86231,#86232,#86233,#86234));
#17930=EDGE_LOOP('',(#86235,#86236,#86237,#86238));
#17931=EDGE_LOOP('',(#86239,#86240,#86241,#86242));
#17932=EDGE_LOOP('',(#86243,#86244,#86245,#86246));
#17933=EDGE_LOOP('',(#86247));
#17934=EDGE_LOOP('',(#86248));
#17935=EDGE_LOOP('',(#86249));
#17936=EDGE_LOOP('',(#86250));
#17937=EDGE_LOOP('',(#86251));
#17938=EDGE_LOOP('',(#86252));
#17939=EDGE_LOOP('',(#86253));
#17940=EDGE_LOOP('',(#86254));
#17941=EDGE_LOOP('',(#86255));
#17942=EDGE_LOOP('',(#86256));
#17943=EDGE_LOOP('',(#86257));
#17944=EDGE_LOOP('',(#86258));
#17945=EDGE_LOOP('',(#86259));
#17946=EDGE_LOOP('',(#86260));
#17947=EDGE_LOOP('',(#86261));
#17948=EDGE_LOOP('',(#86262));
#17949=EDGE_LOOP('',(#86263));
#17950=EDGE_LOOP('',(#86264));
#17951=EDGE_LOOP('',(#86265));
#17952=EDGE_LOOP('',(#86266));
#17953=EDGE_LOOP('',(#86267));
#17954=EDGE_LOOP('',(#86268));
#17955=EDGE_LOOP('',(#86269));
#17956=EDGE_LOOP('',(#86270));
#17957=EDGE_LOOP('',(#86271));
#17958=EDGE_LOOP('',(#86272));
#17959=EDGE_LOOP('',(#86273));
#17960=EDGE_LOOP('',(#86274));
#17961=EDGE_LOOP('',(#86275));
#17962=EDGE_LOOP('',(#86276));
#17963=EDGE_LOOP('',(#86277));
#17964=EDGE_LOOP('',(#86278));
#17965=EDGE_LOOP('',(#86279));
#17966=EDGE_LOOP('',(#86280));
#17967=EDGE_LOOP('',(#86281));
#17968=EDGE_LOOP('',(#86282));
#17969=EDGE_LOOP('',(#86283));
#17970=EDGE_LOOP('',(#86284));
#17971=EDGE_LOOP('',(#86285));
#17972=EDGE_LOOP('',(#86286));
#17973=EDGE_LOOP('',(#86287,#86288,#86289,#86290));
#17974=EDGE_LOOP('',(#86291,#86292,#86293,#86294,#86295,#86296,#86297,#86298,
#86299,#86300,#86301,#86302,#86303,#86304,#86305,#86306,#86307,#86308,#86309,
#86310));
#17975=EDGE_LOOP('',(#86311,#86312,#86313,#86314,#86315,#86316,#86317,#86318,
#86319,#86320,#86321,#86322,#86323,#86324,#86325,#86326,#86327,#86328,#86329));
#17976=EDGE_LOOP('',(#86330,#86331,#86332,#86333));
#17977=EDGE_LOOP('',(#86334,#86335,#86336,#86337));
#17978=EDGE_LOOP('',(#86338,#86339,#86340,#86341,#86342,#86343,#86344,#86345,
#86346,#86347,#86348,#86349,#86350,#86351,#86352,#86353,#86354,#86355,#86356,
#86357));
#17979=EDGE_LOOP('',(#86358,#86359,#86360,#86361,#86362,#86363,#86364,#86365,
#86366,#86367,#86368,#86369,#86370,#86371,#86372,#86373,#86374,#86375,#86376));
#17980=EDGE_LOOP('',(#86377,#86378,#86379,#86380));
#17981=EDGE_LOOP('',(#86381,#86382,#86383,#86384));
#17982=EDGE_LOOP('',(#86385,#86386,#86387,#86388,#86389,#86390,#86391,#86392,
#86393,#86394,#86395,#86396,#86397,#86398,#86399,#86400,#86401,#86402,#86403,
#86404));
#17983=EDGE_LOOP('',(#86405,#86406,#86407,#86408,#86409,#86410,#86411,#86412,
#86413,#86414,#86415,#86416,#86417,#86418,#86419,#86420,#86421,#86422,#86423));
#17984=EDGE_LOOP('',(#86424,#86425,#86426,#86427));
#23374=CIRCLE('',#105177,1.03775);
#23375=CIRCLE('',#105179,1.03775);
#23376=CIRCLE('',#105186,1.03775);
#23377=CIRCLE('',#105188,1.29);
#23378=CIRCLE('',#105196,1.29);
#23379=CIRCLE('',#105198,1.03775);
#23380=CIRCLE('',#105200,1.03775);
#23381=CIRCLE('',#105207,1.03775);
#23382=CIRCLE('',#105209,1.29);
#23383=CIRCLE('',#105217,1.29);
#23384=CIRCLE('',#105219,1.03775);
#23385=CIRCLE('',#105221,1.03775);
#23386=CIRCLE('',#105228,1.03775);
#23387=CIRCLE('',#105230,1.29);
#23388=CIRCLE('',#105238,1.29);
#23389=CIRCLE('',#105240,1.03775);
#23390=CIRCLE('',#105242,1.03775);
#23391=CIRCLE('',#105249,1.03775);
#23392=CIRCLE('',#105251,1.29);
#23393=CIRCLE('',#105259,1.29);
#23394=CIRCLE('',#105261,2.4);
#23395=CIRCLE('',#105262,2.1);
#23396=CIRCLE('',#105264,2.1);
#23397=CIRCLE('',#105265,2.1);
#23398=CIRCLE('',#105267,10.5);
#23399=CIRCLE('',#105270,10.5);
#23400=CIRCLE('',#105271,4.95184441433916);
#23401=CIRCLE('',#105274,9.8);
#23402=CIRCLE('',#105275,9.8);
#23403=CIRCLE('',#105277,3.5);
#23404=CIRCLE('',#105279,3.5);
#23405=CIRCLE('',#105281,10.5);
#23406=CIRCLE('',#105283,10.5);
#23407=CIRCLE('',#105285,4.95184441433916);
#23408=CIRCLE('',#105287,10.5);
#23409=CIRCLE('',#105288,10.5);
#23410=CIRCLE('',#105290,5.08286386254677);
#23411=CIRCLE('',#105291,5.08286386254677);
#23412=CIRCLE('',#105293,10.5);
#23413=CIRCLE('',#105294,10.5);
#23414=CIRCLE('',#105296,5.21388331075437);
#23415=CIRCLE('',#105297,5.21388331075437);
#23416=CIRCLE('',#105299,10.5);
#23417=CIRCLE('',#105300,10.5);
#23418=CIRCLE('',#105302,5.34490275896198);
#23419=CIRCLE('',#105303,5.34490275896198);
#23420=CIRCLE('',#105305,10.5);
#23421=CIRCLE('',#105306,10.5);
#23422=CIRCLE('',#105308,5.47592220716958);
#23423=CIRCLE('',#105309,5.47592220716958);
#23424=CIRCLE('',#105311,10.5);
#23425=CIRCLE('',#105312,10.5);
#23426=CIRCLE('',#105314,5.60694165537719);
#23427=CIRCLE('',#105315,5.60694165537719);
#23428=CIRCLE('',#105317,10.5);
#23429=CIRCLE('',#105318,10.5);
#23430=CIRCLE('',#105320,5.73796110358479);
#23431=CIRCLE('',#105321,5.73796110358479);
#23432=CIRCLE('',#105323,10.5);
#23433=CIRCLE('',#105324,10.5);
#23434=CIRCLE('',#105326,5.8689805517924);
#23435=CIRCLE('',#105327,5.8689805517924);
#23436=CIRCLE('',#105329,10.5);
#23437=CIRCLE('',#105330,10.5);
#23438=CIRCLE('',#105332,6.);
#23439=CIRCLE('',#105333,6.);
#23440=CIRCLE('',#105335,10.5);
#23441=CIRCLE('',#105336,10.5);
#26780=B_SPLINE_CURVE_WITH_KNOTS('',3,(#449399,#449400,#449401,#449402,
#449403,#449404,#449405),.UNSPECIFIED.,.F.,.F.,(4,3,4),(-48.8692190558412,
-47.9084138130922,-47.8494095495406),.UNSPECIFIED.);
#26781=B_SPLINE_CURVE_WITH_KNOTS('',3,(#449411,#449412,#449413,#449414,
#449415,#449416,#449417,#449418,#449419,#449420,#449421,#449422,#449423,
#449424,#449425,#449426,#449427,#449428,#449429),.UNSPECIFIED.,.F.,.F.,
(4,3,3,3,3,3,4),(45.2902480251326,45.9122299042133,46.9103218586527,47.9084138130921,
48.9065057675316,49.904597721971,50.9026896764104),.UNSPECIFIED.);
#26782=B_SPLINE_CURVE_WITH_KNOTS('',3,(#449431,#449432,#449433,#449434,
#449435,#449436,#449437,#449438,#449439,#449440,#449441,#449442,#449443,
#449444,#449445,#449446,#449447,#449448,#449449,#449450,#449451,#449452),
 .UNSPECIFIED.,.F.,.F.,(4,3,3,3,3,3,3,4),(-47.8494095495406,-46.9103218586527,
-45.9122299042133,-44.9141379497739,-43.9160459953345,-42.9179540408951,
-41.9198620864556,-41.5662242423611),.UNSPECIFIED.);
#26783=B_SPLINE_CURVE_WITH_KNOTS('',3,(#449457,#449458,#449459,#449460,
#449461,#449462,#449463,#449464,#449465,#449466,#449467,#449468,#449469,
#449470,#449471,#449472,#449473,#449474,#449475,#449476,#449477,#449478),
 .UNSPECIFIED.,.F.,.F.,(4,3,3,3,3,3,3,4),(39.007062717953,39.9236781775768,
40.9217701320162,41.9198620864556,42.917954040895,43.9160459953345,44.9141379497739,
45.2902480251326),.UNSPECIFIED.);
#26784=B_SPLINE_CURVE_WITH_KNOTS('',3,(#449479,#449480,#449481,#449482,
#449483,#449484,#449485,#449486,#449487,#449488,#449489,#449490,#449491,
#449492,#449493,#449494,#449495,#449496,#449497,#449498,#449499,#449500),
 .UNSPECIFIED.,.F.,.F.,(4,3,3,3,3,3,3,4),(-41.5662242423611,-40.9217701320162,
-39.9236781775768,-38.9255862231374,-37.927494268698,-36.9294023142585,
-35.9313103598191,-35.2830389351814),.UNSPECIFIED.);
#26785=B_SPLINE_CURVE_WITH_KNOTS('',3,(#449505,#449506,#449507,#449508,
#449509,#449510,#449511,#449512,#449513,#449514,#449515,#449516,#449517,
#449518,#449519,#449520,#449521,#449522,#449523,#449524,#449525,#449526,
#449527,#449528,#449529),.UNSPECIFIED.,.F.,.F.,(4,3,3,3,3,3,3,3,4),(32.7238774107735,
32.9370344965008,33.9351264509403,34.9332184053797,35.9313103598191,36.9294023142585,
37.9274942686979,38.9255862231374,39.007062717953),.UNSPECIFIED.);
#26786=B_SPLINE_CURVE_WITH_KNOTS('',3,(#449530,#449531,#449532,#449533,
#449534,#449535,#449536,#449537,#449538,#449539,#449540,#449541,#449542,
#449543,#449544,#449545,#449546,#449547,#449548,#449549,#449550,#449551),
 .UNSPECIFIED.,.F.,.F.,(4,3,3,3,3,3,3,4),(-35.2830389351814,-34.9332184053797,
-33.9351264509403,-32.9370344965009,-31.9389425420614,-30.940850587622,
-29.9427586331826,-28.9998536280018),.UNSPECIFIED.);
#26787=B_SPLINE_CURVE_WITH_KNOTS('',3,(#449556,#449557,#449558,#449559,
#449560,#449561,#449562,#449563,#449564,#449565,#449566,#449567,#449568,
#449569,#449570,#449571,#449572,#449573,#449574,#449575,#449576,#449577),
 .UNSPECIFIED.,.F.,.F.,(4,3,3,3,3,3,3,4),(26.4406921035939,26.9484827698643,
27.9465747243037,28.9446666787432,29.9427586331826,30.940850587622,31.9389425420614,
32.7238774107735),.UNSPECIFIED.);
#26788=B_SPLINE_CURVE_WITH_KNOTS('',3,(#449578,#449579,#449580,#449581,
#449582,#449583,#449584,#449585,#449586,#449587,#449588,#449589,#449590,
#449591,#449592,#449593,#449594,#449595,#449596,#449597,#449598,#449599,
#449600,#449601,#449602),.UNSPECIFIED.,.F.,.F.,(4,3,3,3,3,3,3,3,4),(-28.9998536280018,
-28.9446666787432,-27.9465747243038,-26.9484827698643,-25.9503908154249,
-24.9522988609855,-23.9542069065461,-22.9561149521067,-22.7166683208223),
 .UNSPECIFIED.);
#26789=B_SPLINE_CURVE_WITH_KNOTS('',3,(#449607,#449608,#449609,#449610,
#449611,#449612,#449613,#449614,#449615,#449616,#449617,#449618,#449619,
#449620,#449621,#449622,#449623,#449624,#449625,#449626,#449627,#449628),
 .UNSPECIFIED.,.F.,.F.,(4,3,3,3,3,3,3,4),(20.1575067964143,20.9599310432278,
21.9580229976672,22.9561149521067,23.9542069065461,24.9522988609855,25.9503908154249,
26.4406921035939),.UNSPECIFIED.);
#26790=B_SPLINE_CURVE_WITH_KNOTS('',3,(#449629,#449630,#449631,#449632,
#449633,#449634,#449635,#449636,#449637,#449638,#449639,#449640,#449641,
#449642,#449643,#449644,#449645,#449646,#449647,#449648,#449649,#449650),
 .UNSPECIFIED.,.F.,.F.,(4,3,3,3,3,3,3,4),(-22.7166683208223,-21.9580229976672,
-20.9599310432278,-19.9618390887884,-18.963747134349,-17.9656551799096,
-16.9675632254701,-16.4334830136427),.UNSPECIFIED.);
#26791=B_SPLINE_CURVE_WITH_KNOTS('',3,(#449655,#449656,#449657,#449658,
#449659,#449660,#449661,#449662,#449663,#449664,#449665,#449666,#449667,
#449668,#449669,#449670,#449671,#449672,#449673,#449674,#449675,#449676,
#449677,#449678,#449679),.UNSPECIFIED.,.F.,.F.,(4,3,3,3,3,3,3,3,4),(13.8743214892347,
13.9732873621519,14.9713793165913,15.9694712710307,16.9675632254701,17.9656551799096,
18.963747134349,19.9618390887884,20.1575067964143),.UNSPECIFIED.);
#26792=B_SPLINE_CURVE_WITH_KNOTS('',3,(#449680,#449681,#449682,#449683,
#449684,#449685,#449686,#449687,#449688,#449689,#449690,#449691,#449692,
#449693,#449694,#449695,#449696,#449697,#449698,#449699,#449700,#449701),
 .UNSPECIFIED.,.F.,.F.,(4,3,3,3,3,3,3,4),(-16.4334830136427,-15.9694712710307,
-14.9713793165913,-13.9732873621519,-12.9751954077125,-11.977103453273,
-10.9790114988336,-10.1502977064631),.UNSPECIFIED.);
#26793=B_SPLINE_CURVE_WITH_KNOTS('',3,(#449707,#449708,#449709,#449710,
#449711,#449712,#449713,#449714,#449715,#449716,#449717,#449718,#449719),
 .UNSPECIFIED.,.F.,.F.,(4,3,3,3,4),(-3.86711239928348,-2.99427586331826,
-1.99618390887884,-0.998091954439421,0.),.UNSPECIFIED.);
#26794=B_SPLINE_CURVE_WITH_KNOTS('',3,(#449722,#449723,#449724,#449725,
#449726,#449727,#449728,#449729,#449730,#449731,#449732,#449733,#449734,
#449735,#449736,#449737,#449738,#449739,#449740),.UNSPECIFIED.,.F.,.F.,
(4,3,3,3,3,3,4),(2.03347062056922,2.99427586331826,3.99236781775768,4.9904597721971,
5.98855172663652,6.98664368107594,7.59113618205511),.UNSPECIFIED.);
#26795=B_SPLINE_CURVE_WITH_KNOTS('',3,(#449746,#449747,#449748,#449749,
#449750,#449751,#449752),.UNSPECIFIED.,.F.,.F.,(4,1,1,1,4),(59.6902604182061,
59.7492646817576,60.747356636197,61.7454485906364,62.7435405450759),
 .UNSPECIFIED.);
#26796=B_SPLINE_CURVE_WITH_KNOTS('',3,(#449755,#449756,#449757,#449758,
#449759,#449760,#449761),.UNSPECIFIED.,.F.,.F.,(4,1,1,1,4),(59.6902604182061,
60.3122422972867,61.3103342517261,62.3084262061655,63.2692314489146),
 .UNSPECIFIED.);
#26797=B_SPLINE_CURVE_WITH_KNOTS('',3,(#449766,#449767,#449768,#449769,
#449770,#449771,#449772,#449773,#449774,#449775),.UNSPECIFIED.,.F.,.F.,
(4,1,1,1,1,1,1,4),(53.4070751110265,53.7607129551211,54.7588049095605,55.7568968639999,
56.7549888184393,57.7530807728788,58.7511727273182,59.6902604182061),
 .UNSPECIFIED.);
#26798=B_SPLINE_CURVE_WITH_KNOTS('',3,(#449776,#449777,#449778,#449779,
#449780,#449781,#449782,#449783,#449784,#449785),.UNSPECIFIED.,.F.,.F.,
(4,1,1,1,1,1,1,4),(53.4070751110265,54.3236905706502,55.3217825250896,56.319874479529,
57.3179664339684,58.3160583884079,59.3141503428473,59.6902604182061),
 .UNSPECIFIED.);
#26799=B_SPLINE_CURVE_WITH_KNOTS('',3,(#449790,#449791,#449792,#449793,
#449794,#449795,#449796,#449797,#449798,#449799),.UNSPECIFIED.,.F.,.F.,
(4,1,1,1,1,1,1,4),(47.1238898038469,47.7721612284846,48.770253182924,49.7683451373634,
50.7664370918028,51.7645290462422,52.7626210006817,53.4070751110265),
 .UNSPECIFIED.);
#26800=B_SPLINE_CURVE_WITH_KNOTS('',3,(#449800,#449801,#449802,#449803,
#449804,#449805,#449806,#449807,#449808,#449809,#449810),.UNSPECIFIED.,
 .F.,.F.,(4,1,1,1,1,1,1,1,4),(47.1238898038469,47.3370468895742,48.3351388440137,
49.3332307984531,50.3313227528925,51.3294147073319,52.3275066617713,53.3255986162108,
53.4070751110265),.UNSPECIFIED.);
#26801=B_SPLINE_CURVE_WITH_KNOTS('',3,(#449815,#449816,#449817,#449818,
#449819,#449820,#449821,#449822,#449823,#449824),.UNSPECIFIED.,.F.,.F.,
(4,1,1,1,1,1,1,4),(40.8407044966673,41.783609501848,42.7817014562875,43.7797934107269,
44.7778853651663,45.7759773196057,46.7740692740451,47.1238898038469),
 .UNSPECIFIED.);
#26802=B_SPLINE_CURVE_WITH_KNOTS('',3,(#449825,#449826,#449827,#449828,
#449829,#449830,#449831,#449832,#449833,#449834),.UNSPECIFIED.,.F.,.F.,
(4,1,1,1,1,1,1,4),(40.8407044966673,41.3484951629377,42.3465871173771,43.3446790718166,
44.342771026256,45.3408629806954,46.3389549351348,47.1238898038469),
 .UNSPECIFIED.);
#26803=B_SPLINE_CURVE_WITH_KNOTS('',3,(#449839,#449840,#449841,#449842,
#449843,#449844,#449845,#449846,#449847,#449848,#449849),.UNSPECIFIED.,
 .F.,.F.,(4,1,1,1,1,1,1,1,4),(34.5575191894877,34.7969658207721,35.7950577752115,
36.7931497296509,37.7912416840904,38.7893336385298,39.7874255929692,40.7855175474086,
40.8407044966673),.UNSPECIFIED.);
#26804=B_SPLINE_CURVE_WITH_KNOTS('',3,(#449850,#449851,#449852,#449853,
#449854,#449855,#449856,#449857,#449858,#449859),.UNSPECIFIED.,.F.,.F.,
(4,1,1,1,1,1,1,4),(34.5575191894877,35.3599434363012,36.3580353907406,37.35612734518,
38.3542192996195,39.3523112540589,40.3504032084983,40.8407044966673),
 .UNSPECIFIED.);
#26805=B_SPLINE_CURVE_WITH_KNOTS('',3,(#449864,#449865,#449866,#449867,
#449868,#449869,#449870,#449871,#449872,#449873),.UNSPECIFIED.,.F.,.F.,
(4,1,1,1,1,1,1,4),(28.2743338823081,28.8084140941356,29.806506048575,30.8045980030144,
31.8026899574538,32.8007819118933,33.7988738663327,34.5575191894877),
 .UNSPECIFIED.);
#26806=B_SPLINE_CURVE_WITH_KNOTS('',3,(#449874,#449875,#449876,#449877,
#449878,#449879,#449880,#449881,#449882,#449883,#449884),.UNSPECIFIED.,
 .F.,.F.,(4,1,1,1,1,1,1,1,4),(28.2743338823081,28.3732997552253,29.3713917096647,
30.3694836641041,31.3675756185435,32.3656675729829,33.3637595274224,34.3618514818618,
34.5575191894877),.UNSPECIFIED.);
#26807=B_SPLINE_CURVE_WITH_KNOTS('',3,(#449889,#449890,#449891,#449892,
#449893,#449894,#449895,#449896,#449897,#449898),.UNSPECIFIED.,.F.,.F.,
(4,1,1,1,1,1,1,4),(21.9911485751285,22.8198623674991,23.8179543219385,24.8160462763779,
25.8141382308173,26.8122301852567,27.8103221396962,28.2743338823081),
 .UNSPECIFIED.);
#26808=B_SPLINE_CURVE_WITH_KNOTS('',3,(#449899,#449900,#449901,#449902,
#449903,#449904,#449905,#449906,#449907,#449908),.UNSPECIFIED.,.F.,.F.,
(4,1,1,1,1,1,1,4),(21.9911485751285,22.3847480285887,23.3828399830282,24.3809319374676,
25.379023891907,26.3771158463464,27.3752078007858,28.2743338823081),
 .UNSPECIFIED.);
#26809=B_SPLINE_CURVE_WITH_KNOTS('',3,(#449914,#449915,#449916,#449917,
#449918),.UNSPECIFIED.,.F.,.F.,(4,1,4),(14.4000123930734,15.3981043475128,
15.7079632679489),.UNSPECIFIED.);
#26810=B_SPLINE_CURVE_WITH_KNOTS('',3,(#449921,#449922,#449923,#449924,
#449925),.UNSPECIFIED.,.F.,.F.,(4,1,4),(13.8743214892347,14.8351267319837,
15.7079632679489),.UNSPECIFIED.);
#26811=B_SPLINE_CURVE_WITH_KNOTS('',3,(#449932,#449933,#449934,#449935,
#449936,#449937,#449938),.UNSPECIFIED.,.F.,.F.,(4,3,4),(-48.8692190558412,
-47.9084138130922,-47.8494095495406),.UNSPECIFIED.);
#26812=B_SPLINE_CURVE_WITH_KNOTS('',3,(#449944,#449945,#449946,#449947,
#449948,#449949,#449950,#449951,#449952,#449953,#449954,#449955,#449956,
#449957,#449958,#449959,#449960,#449961,#449962),.UNSPECIFIED.,.F.,.F.,
(4,3,3,3,3,3,4),(45.2902480251326,45.9122299042133,46.9103218586527,47.9084138130921,
48.9065057675316,49.904597721971,50.9026896764104),.UNSPECIFIED.);
#26813=B_SPLINE_CURVE_WITH_KNOTS('',3,(#449964,#449965,#449966,#449967,
#449968,#449969,#449970,#449971,#449972,#449973,#449974,#449975,#449976,
#449977,#449978,#449979,#449980,#449981,#449982,#449983,#449984,#449985),
 .UNSPECIFIED.,.F.,.F.,(4,3,3,3,3,3,3,4),(-47.8494095495406,-46.9103218586527,
-45.9122299042133,-44.9141379497739,-43.9160459953345,-42.9179540408951,
-41.9198620864556,-41.5662242423611),.UNSPECIFIED.);
#26814=B_SPLINE_CURVE_WITH_KNOTS('',3,(#449990,#449991,#449992,#449993,
#449994,#449995,#449996,#449997,#449998,#449999,#450000,#450001,#450002,
#450003,#450004,#450005,#450006,#450007,#450008,#450009,#450010,#450011),
 .UNSPECIFIED.,.F.,.F.,(4,3,3,3,3,3,3,4),(39.007062717953,39.9236781775768,
40.9217701320162,41.9198620864556,42.917954040895,43.9160459953345,44.9141379497739,
45.2902480251326),.UNSPECIFIED.);
#26815=B_SPLINE_CURVE_WITH_KNOTS('',3,(#450012,#450013,#450014,#450015,
#450016,#450017,#450018,#450019,#450020,#450021,#450022,#450023,#450024,
#450025,#450026,#450027,#450028,#450029,#450030,#450031,#450032,#450033),
 .UNSPECIFIED.,.F.,.F.,(4,3,3,3,3,3,3,4),(-41.5662242423611,-40.9217701320162,
-39.9236781775768,-38.9255862231374,-37.927494268698,-36.9294023142585,
-35.9313103598191,-35.2830389351814),.UNSPECIFIED.);
#26816=B_SPLINE_CURVE_WITH_KNOTS('',3,(#450038,#450039,#450040,#450041,
#450042,#450043,#450044,#450045,#450046,#450047,#450048,#450049,#450050,
#450051,#450052,#450053,#450054,#450055,#450056,#450057,#450058,#450059,
#450060,#450061,#450062),.UNSPECIFIED.,.F.,.F.,(4,3,3,3,3,3,3,3,4),(32.7238774107735,
32.9370344965008,33.9351264509403,34.9332184053797,35.9313103598191,36.9294023142585,
37.9274942686979,38.9255862231374,39.007062717953),.UNSPECIFIED.);
#26817=B_SPLINE_CURVE_WITH_KNOTS('',3,(#450063,#450064,#450065,#450066,
#450067,#450068,#450069,#450070,#450071,#450072,#450073,#450074,#450075,
#450076,#450077,#450078,#450079,#450080,#450081,#450082,#450083,#450084),
 .UNSPECIFIED.,.F.,.F.,(4,3,3,3,3,3,3,4),(-35.2830389351814,-34.9332184053797,
-33.9351264509403,-32.9370344965009,-31.9389425420614,-30.940850587622,
-29.9427586331826,-28.9998536280018),.UNSPECIFIED.);
#26818=B_SPLINE_CURVE_WITH_KNOTS('',3,(#450089,#450090,#450091,#450092,
#450093,#450094,#450095,#450096,#450097,#450098,#450099,#450100,#450101,
#450102,#450103,#450104,#450105,#450106,#450107,#450108,#450109,#450110),
 .UNSPECIFIED.,.F.,.F.,(4,3,3,3,3,3,3,4),(26.4406921035939,26.9484827698643,
27.9465747243037,28.9446666787432,29.9427586331826,30.940850587622,31.9389425420614,
32.7238774107735),.UNSPECIFIED.);
#26819=B_SPLINE_CURVE_WITH_KNOTS('',3,(#450111,#450112,#450113,#450114,
#450115,#450116,#450117,#450118,#450119,#450120,#450121,#450122,#450123,
#450124,#450125,#450126,#450127,#450128,#450129,#450130,#450131,#450132,
#450133,#450134,#450135),.UNSPECIFIED.,.F.,.F.,(4,3,3,3,3,3,3,3,4),(-28.9998536280018,
-28.9446666787432,-27.9465747243038,-26.9484827698643,-25.9503908154249,
-24.9522988609855,-23.9542069065461,-22.9561149521067,-22.7166683208223),
 .UNSPECIFIED.);
#26820=B_SPLINE_CURVE_WITH_KNOTS('',3,(#450140,#450141,#450142,#450143,
#450144,#450145,#450146,#450147,#450148,#450149,#450150,#450151,#450152,
#450153,#450154,#450155,#450156,#450157,#450158,#450159,#450160,#450161),
 .UNSPECIFIED.,.F.,.F.,(4,3,3,3,3,3,3,4),(20.1575067964143,20.9599310432278,
21.9580229976672,22.9561149521067,23.9542069065461,24.9522988609855,25.9503908154249,
26.4406921035939),.UNSPECIFIED.);
#26821=B_SPLINE_CURVE_WITH_KNOTS('',3,(#450162,#450163,#450164,#450165,
#450166,#450167,#450168,#450169,#450170,#450171,#450172,#450173,#450174,
#450175,#450176,#450177,#450178,#450179,#450180,#450181,#450182,#450183),
 .UNSPECIFIED.,.F.,.F.,(4,3,3,3,3,3,3,4),(-22.7166683208223,-21.9580229976672,
-20.9599310432278,-19.9618390887884,-18.963747134349,-17.9656551799096,
-16.9675632254701,-16.4334830136427),.UNSPECIFIED.);
#26822=B_SPLINE_CURVE_WITH_KNOTS('',3,(#450188,#450189,#450190,#450191,
#450192,#450193,#450194,#450195,#450196,#450197,#450198,#450199,#450200,
#450201,#450202,#450203,#450204,#450205,#450206,#450207,#450208,#450209,
#450210,#450211,#450212),.UNSPECIFIED.,.F.,.F.,(4,3,3,3,3,3,3,3,4),(13.8743214892347,
13.9732873621519,14.9713793165913,15.9694712710307,16.9675632254701,17.9656551799096,
18.963747134349,19.9618390887884,20.1575067964143),.UNSPECIFIED.);
#26823=B_SPLINE_CURVE_WITH_KNOTS('',3,(#450213,#450214,#450215,#450216,
#450217,#450218,#450219,#450220,#450221,#450222,#450223,#450224,#450225,
#450226,#450227,#450228,#450229,#450230,#450231,#450232,#450233,#450234),
 .UNSPECIFIED.,.F.,.F.,(4,3,3,3,3,3,3,4),(-16.4334830136427,-15.9694712710307,
-14.9713793165913,-13.9732873621519,-12.9751954077125,-11.977103453273,
-10.9790114988336,-10.1502977064631),.UNSPECIFIED.);
#26824=B_SPLINE_CURVE_WITH_KNOTS('',3,(#450240,#450241,#450242,#450243,
#450244,#450245,#450246,#450247,#450248,#450249,#450250,#450251,#450252),
 .UNSPECIFIED.,.F.,.F.,(4,3,3,3,4),(-3.86711239928348,-2.99427586331826,
-1.99618390887884,-0.998091954439421,0.),.UNSPECIFIED.);
#26825=B_SPLINE_CURVE_WITH_KNOTS('',3,(#450255,#450256,#450257,#450258,
#450259,#450260,#450261,#450262,#450263,#450264,#450265,#450266,#450267,
#450268,#450269,#450270,#450271,#450272,#450273),.UNSPECIFIED.,.F.,.F.,
(4,3,3,3,3,3,4),(2.03347062056922,2.99427586331826,3.99236781775768,4.9904597721971,
5.98855172663652,6.98664368107594,7.59113618205511),.UNSPECIFIED.);
#26826=B_SPLINE_CURVE_WITH_KNOTS('',3,(#450279,#450280,#450281,#450282,
#450283,#450284,#450285),.UNSPECIFIED.,.F.,.F.,(4,1,1,1,4),(59.6902604182061,
59.7492646817576,60.747356636197,61.7454485906364,62.7435405450759),
 .UNSPECIFIED.);
#26827=B_SPLINE_CURVE_WITH_KNOTS('',3,(#450288,#450289,#450290,#450291,
#450292,#450293,#450294),.UNSPECIFIED.,.F.,.F.,(4,1,1,1,4),(59.6902604182061,
60.3122422972867,61.3103342517261,62.3084262061655,63.2692314489146),
 .UNSPECIFIED.);
#26828=B_SPLINE_CURVE_WITH_KNOTS('',3,(#450299,#450300,#450301,#450302,
#450303,#450304,#450305,#450306,#450307,#450308),.UNSPECIFIED.,.F.,.F.,
(4,1,1,1,1,1,1,4),(53.4070751110265,53.7607129551211,54.7588049095605,55.7568968639999,
56.7549888184393,57.7530807728788,58.7511727273182,59.6902604182061),
 .UNSPECIFIED.);
#26829=B_SPLINE_CURVE_WITH_KNOTS('',3,(#450309,#450310,#450311,#450312,
#450313,#450314,#450315,#450316,#450317,#450318),.UNSPECIFIED.,.F.,.F.,
(4,1,1,1,1,1,1,4),(53.4070751110265,54.3236905706502,55.3217825250896,56.319874479529,
57.3179664339684,58.3160583884079,59.3141503428473,59.6902604182061),
 .UNSPECIFIED.);
#26830=B_SPLINE_CURVE_WITH_KNOTS('',3,(#450323,#450324,#450325,#450326,
#450327,#450328,#450329,#450330,#450331,#450332),.UNSPECIFIED.,.F.,.F.,
(4,1,1,1,1,1,1,4),(47.1238898038469,47.7721612284846,48.770253182924,49.7683451373634,
50.7664370918028,51.7645290462422,52.7626210006817,53.4070751110265),
 .UNSPECIFIED.);
#26831=B_SPLINE_CURVE_WITH_KNOTS('',3,(#450333,#450334,#450335,#450336,
#450337,#450338,#450339,#450340,#450341,#450342,#450343),.UNSPECIFIED.,
 .F.,.F.,(4,1,1,1,1,1,1,1,4),(47.1238898038469,47.3370468895742,48.3351388440137,
49.3332307984531,50.3313227528925,51.3294147073319,52.3275066617713,53.3255986162108,
53.4070751110265),.UNSPECIFIED.);
#26832=B_SPLINE_CURVE_WITH_KNOTS('',3,(#450348,#450349,#450350,#450351,
#450352,#450353,#450354,#450355,#450356,#450357),.UNSPECIFIED.,.F.,.F.,
(4,1,1,1,1,1,1,4),(40.8407044966673,41.783609501848,42.7817014562875,43.7797934107269,
44.7778853651663,45.7759773196057,46.7740692740451,47.1238898038469),
 .UNSPECIFIED.);
#26833=B_SPLINE_CURVE_WITH_KNOTS('',3,(#450358,#450359,#450360,#450361,
#450362,#450363,#450364,#450365,#450366,#450367),.UNSPECIFIED.,.F.,.F.,
(4,1,1,1,1,1,1,4),(40.8407044966673,41.3484951629377,42.3465871173771,43.3446790718166,
44.342771026256,45.3408629806954,46.3389549351348,47.1238898038469),
 .UNSPECIFIED.);
#26834=B_SPLINE_CURVE_WITH_KNOTS('',3,(#450372,#450373,#450374,#450375,
#450376,#450377,#450378,#450379,#450380,#450381,#450382),.UNSPECIFIED.,
 .F.,.F.,(4,1,1,1,1,1,1,1,4),(34.5575191894877,34.7969658207721,35.7950577752115,
36.7931497296509,37.7912416840904,38.7893336385298,39.7874255929692,40.7855175474086,
40.8407044966673),.UNSPECIFIED.);
#26835=B_SPLINE_CURVE_WITH_KNOTS('',3,(#450383,#450384,#450385,#450386,
#450387,#450388,#450389,#450390,#450391,#450392),.UNSPECIFIED.,.F.,.F.,
(4,1,1,1,1,1,1,4),(34.5575191894877,35.3599434363012,36.3580353907406,37.35612734518,
38.3542192996195,39.3523112540589,40.3504032084983,40.8407044966673),
 .UNSPECIFIED.);
#26836=B_SPLINE_CURVE_WITH_KNOTS('',3,(#450397,#450398,#450399,#450400,
#450401,#450402,#450403,#450404,#450405,#450406),.UNSPECIFIED.,.F.,.F.,
(4,1,1,1,1,1,1,4),(28.2743338823081,28.8084140941356,29.806506048575,30.8045980030144,
31.8026899574538,32.8007819118933,33.7988738663327,34.5575191894877),
 .UNSPECIFIED.);
#26837=B_SPLINE_CURVE_WITH_KNOTS('',3,(#450407,#450408,#450409,#450410,
#450411,#450412,#450413,#450414,#450415,#450416,#450417),.UNSPECIFIED.,
 .F.,.F.,(4,1,1,1,1,1,1,1,4),(28.2743338823081,28.3732997552253,29.3713917096647,
30.3694836641041,31.3675756185435,32.3656675729829,33.3637595274224,34.3618514818618,
34.5575191894877),.UNSPECIFIED.);
#26838=B_SPLINE_CURVE_WITH_KNOTS('',3,(#450422,#450423,#450424,#450425,
#450426,#450427,#450428,#450429,#450430,#450431),.UNSPECIFIED.,.F.,.F.,
(4,1,1,1,1,1,1,4),(21.9911485751285,22.8198623674991,23.8179543219385,24.8160462763779,
25.8141382308173,26.8122301852567,27.8103221396962,28.2743338823081),
 .UNSPECIFIED.);
#26839=B_SPLINE_CURVE_WITH_KNOTS('',3,(#450432,#450433,#450434,#450435,
#450436,#450437,#450438,#450439,#450440,#450441),.UNSPECIFIED.,.F.,.F.,
(4,1,1,1,1,1,1,4),(21.9911485751285,22.3847480285887,23.3828399830282,24.3809319374676,
25.379023891907,26.3771158463464,27.3752078007858,28.2743338823081),
 .UNSPECIFIED.);
#26840=B_SPLINE_CURVE_WITH_KNOTS('',3,(#450447,#450448,#450449,#450450,
#450451),.UNSPECIFIED.,.F.,.F.,(4,1,4),(14.4000123930734,15.3981043475128,
15.7079632679489),.UNSPECIFIED.);
#26841=B_SPLINE_CURVE_WITH_KNOTS('',3,(#450454,#450455,#450456,#450457,
#450458),.UNSPECIFIED.,.F.,.F.,(4,1,4),(13.8743214892347,14.8351267319837,
15.7079632679489),.UNSPECIFIED.);
#26842=B_SPLINE_CURVE_WITH_KNOTS('',3,(#450465,#450466,#450467,#450468,
#450469,#450470,#450471),.UNSPECIFIED.,.F.,.F.,(4,3,4),(-48.8692190558412,
-47.9084138130922,-47.8494095495406),.UNSPECIFIED.);
#26843=B_SPLINE_CURVE_WITH_KNOTS('',3,(#450477,#450478,#450479,#450480,
#450481,#450482,#450483,#450484,#450485,#450486,#450487,#450488,#450489,
#450490,#450491,#450492,#450493,#450494,#450495),.UNSPECIFIED.,.F.,.F.,
(4,3,3,3,3,3,4),(45.2902480251326,45.9122299042133,46.9103218586527,47.9084138130921,
48.9065057675316,49.904597721971,50.9026896764104),.UNSPECIFIED.);
#26844=B_SPLINE_CURVE_WITH_KNOTS('',3,(#450497,#450498,#450499,#450500,
#450501,#450502,#450503,#450504,#450505,#450506,#450507,#450508,#450509,
#450510,#450511,#450512,#450513,#450514,#450515,#450516,#450517,#450518),
 .UNSPECIFIED.,.F.,.F.,(4,3,3,3,3,3,3,4),(-47.8494095495406,-46.9103218586527,
-45.9122299042133,-44.9141379497739,-43.9160459953345,-42.9179540408951,
-41.9198620864556,-41.5662242423611),.UNSPECIFIED.);
#26845=B_SPLINE_CURVE_WITH_KNOTS('',3,(#450523,#450524,#450525,#450526,
#450527,#450528,#450529,#450530,#450531,#450532,#450533,#450534,#450535,
#450536,#450537,#450538,#450539,#450540,#450541,#450542,#450543,#450544),
 .UNSPECIFIED.,.F.,.F.,(4,3,3,3,3,3,3,4),(39.007062717953,39.9236781775768,
40.9217701320162,41.9198620864556,42.917954040895,43.9160459953345,44.9141379497739,
45.2902480251326),.UNSPECIFIED.);
#26846=B_SPLINE_CURVE_WITH_KNOTS('',3,(#450545,#450546,#450547,#450548,
#450549,#450550,#450551,#450552,#450553,#450554,#450555,#450556,#450557,
#450558,#450559,#450560,#450561,#450562,#450563,#450564,#450565,#450566),
 .UNSPECIFIED.,.F.,.F.,(4,3,3,3,3,3,3,4),(-41.5662242423611,-40.9217701320162,
-39.9236781775768,-38.9255862231374,-37.927494268698,-36.9294023142585,
-35.9313103598191,-35.2830389351814),.UNSPECIFIED.);
#26847=B_SPLINE_CURVE_WITH_KNOTS('',3,(#450571,#450572,#450573,#450574,
#450575,#450576,#450577,#450578,#450579,#450580,#450581,#450582,#450583,
#450584,#450585,#450586,#450587,#450588,#450589,#450590,#450591,#450592,
#450593,#450594,#450595),.UNSPECIFIED.,.F.,.F.,(4,3,3,3,3,3,3,3,4),(32.7238774107735,
32.9370344965008,33.9351264509403,34.9332184053797,35.9313103598191,36.9294023142585,
37.9274942686979,38.9255862231374,39.007062717953),.UNSPECIFIED.);
#26848=B_SPLINE_CURVE_WITH_KNOTS('',3,(#450596,#450597,#450598,#450599,
#450600,#450601,#450602,#450603,#450604,#450605,#450606,#450607,#450608,
#450609,#450610,#450611,#450612,#450613,#450614,#450615,#450616,#450617),
 .UNSPECIFIED.,.F.,.F.,(4,3,3,3,3,3,3,4),(-35.2830389351814,-34.9332184053797,
-33.9351264509403,-32.9370344965009,-31.9389425420614,-30.940850587622,
-29.9427586331826,-28.9998536280018),.UNSPECIFIED.);
#26849=B_SPLINE_CURVE_WITH_KNOTS('',3,(#450622,#450623,#450624,#450625,
#450626,#450627,#450628,#450629,#450630,#450631,#450632,#450633,#450634,
#450635,#450636,#450637,#450638,#450639,#450640,#450641,#450642,#450643),
 .UNSPECIFIED.,.F.,.F.,(4,3,3,3,3,3,3,4),(26.4406921035939,26.9484827698643,
27.9465747243037,28.9446666787432,29.9427586331826,30.940850587622,31.9389425420614,
32.7238774107735),.UNSPECIFIED.);
#26850=B_SPLINE_CURVE_WITH_KNOTS('',3,(#450644,#450645,#450646,#450647,
#450648,#450649,#450650,#450651,#450652,#450653,#450654,#450655,#450656,
#450657,#450658,#450659,#450660,#450661,#450662,#450663,#450664,#450665,
#450666,#450667,#450668),.UNSPECIFIED.,.F.,.F.,(4,3,3,3,3,3,3,3,4),(-28.9998536280018,
-28.9446666787432,-27.9465747243038,-26.9484827698643,-25.9503908154249,
-24.9522988609855,-23.9542069065461,-22.9561149521067,-22.7166683208223),
 .UNSPECIFIED.);
#26851=B_SPLINE_CURVE_WITH_KNOTS('',3,(#450673,#450674,#450675,#450676,
#450677,#450678,#450679,#450680,#450681,#450682,#450683,#450684,#450685,
#450686,#450687,#450688,#450689,#450690,#450691,#450692,#450693,#450694),
 .UNSPECIFIED.,.F.,.F.,(4,3,3,3,3,3,3,4),(20.1575067964143,20.9599310432278,
21.9580229976672,22.9561149521067,23.9542069065461,24.9522988609855,25.9503908154249,
26.4406921035939),.UNSPECIFIED.);
#26852=B_SPLINE_CURVE_WITH_KNOTS('',3,(#450695,#450696,#450697,#450698,
#450699,#450700,#450701,#450702,#450703,#450704,#450705,#450706,#450707,
#450708,#450709,#450710,#450711,#450712,#450713,#450714,#450715,#450716),
 .UNSPECIFIED.,.F.,.F.,(4,3,3,3,3,3,3,4),(-22.7166683208223,-21.9580229976672,
-20.9599310432278,-19.9618390887884,-18.963747134349,-17.9656551799096,
-16.9675632254701,-16.4334830136427),.UNSPECIFIED.);
#26853=B_SPLINE_CURVE_WITH_KNOTS('',3,(#450721,#450722,#450723,#450724,
#450725,#450726,#450727,#450728,#450729,#450730,#450731,#450732,#450733,
#450734,#450735,#450736,#450737,#450738,#450739,#450740,#450741,#450742,
#450743,#450744,#450745),.UNSPECIFIED.,.F.,.F.,(4,3,3,3,3,3,3,3,4),(13.8743214892347,
13.9732873621519,14.9713793165913,15.9694712710307,16.9675632254701,17.9656551799096,
18.963747134349,19.9618390887884,20.1575067964143),.UNSPECIFIED.);
#26854=B_SPLINE_CURVE_WITH_KNOTS('',3,(#450746,#450747,#450748,#450749,
#450750,#450751,#450752,#450753,#450754,#450755,#450756,#450757,#450758,
#450759,#450760,#450761,#450762,#450763,#450764,#450765,#450766,#450767),
 .UNSPECIFIED.,.F.,.F.,(4,3,3,3,3,3,3,4),(-16.4334830136427,-15.9694712710307,
-14.9713793165913,-13.9732873621519,-12.9751954077125,-11.977103453273,
-10.9790114988336,-10.1502977064631),.UNSPECIFIED.);
#26855=B_SPLINE_CURVE_WITH_KNOTS('',3,(#450773,#450774,#450775,#450776,
#450777,#450778,#450779,#450780,#450781,#450782,#450783,#450784,#450785),
 .UNSPECIFIED.,.F.,.F.,(4,3,3,3,4),(-3.86711239928348,-2.99427586331826,
-1.99618390887884,-0.998091954439421,0.),.UNSPECIFIED.);
#26856=B_SPLINE_CURVE_WITH_KNOTS('',3,(#450788,#450789,#450790,#450791,
#450792,#450793,#450794,#450795,#450796,#450797,#450798,#450799,#450800,
#450801,#450802,#450803,#450804,#450805,#450806),.UNSPECIFIED.,.F.,.F.,
(4,3,3,3,3,3,4),(2.03347062056922,2.99427586331826,3.99236781775768,4.9904597721971,
5.98855172663652,6.98664368107594,7.59113618205511),.UNSPECIFIED.);
#26857=B_SPLINE_CURVE_WITH_KNOTS('',3,(#450812,#450813,#450814,#450815,
#450816,#450817,#450818),.UNSPECIFIED.,.F.,.F.,(4,1,1,1,4),(59.6902604182061,
59.7492646817576,60.747356636197,61.7454485906364,62.7435405450759),
 .UNSPECIFIED.);
#26858=B_SPLINE_CURVE_WITH_KNOTS('',3,(#450821,#450822,#450823,#450824,
#450825,#450826,#450827),.UNSPECIFIED.,.F.,.F.,(4,1,1,1,4),(59.6902604182061,
60.3122422972867,61.3103342517261,62.3084262061655,63.2692314489146),
 .UNSPECIFIED.);
#26859=B_SPLINE_CURVE_WITH_KNOTS('',3,(#450832,#450833,#450834,#450835,
#450836,#450837,#450838,#450839,#450840,#450841),.UNSPECIFIED.,.F.,.F.,
(4,1,1,1,1,1,1,4),(53.4070751110265,53.7607129551211,54.7588049095605,55.7568968639999,
56.7549888184393,57.7530807728788,58.7511727273182,59.6902604182061),
 .UNSPECIFIED.);
#26860=B_SPLINE_CURVE_WITH_KNOTS('',3,(#450842,#450843,#450844,#450845,
#450846,#450847,#450848,#450849,#450850,#450851),.UNSPECIFIED.,.F.,.F.,
(4,1,1,1,1,1,1,4),(53.4070751110265,54.3236905706502,55.3217825250896,56.319874479529,
57.3179664339684,58.3160583884079,59.3141503428473,59.6902604182061),
 .UNSPECIFIED.);
#26861=B_SPLINE_CURVE_WITH_KNOTS('',3,(#450856,#450857,#450858,#450859,
#450860,#450861,#450862,#450863,#450864,#450865),.UNSPECIFIED.,.F.,.F.,
(4,1,1,1,1,1,1,4),(47.1238898038469,47.7721612284846,48.770253182924,49.7683451373634,
50.7664370918028,51.7645290462422,52.7626210006817,53.4070751110265),
 .UNSPECIFIED.);
#26862=B_SPLINE_CURVE_WITH_KNOTS('',3,(#450866,#450867,#450868,#450869,
#450870,#450871,#450872,#450873,#450874,#450875,#450876),.UNSPECIFIED.,
 .F.,.F.,(4,1,1,1,1,1,1,1,4),(47.1238898038469,47.3370468895742,48.3351388440137,
49.3332307984531,50.3313227528925,51.3294147073319,52.3275066617713,53.3255986162108,
53.4070751110265),.UNSPECIFIED.);
#26863=B_SPLINE_CURVE_WITH_KNOTS('',3,(#450881,#450882,#450883,#450884,
#450885,#450886,#450887,#450888,#450889,#450890),.UNSPECIFIED.,.F.,.F.,
(4,1,1,1,1,1,1,4),(40.8407044966673,41.783609501848,42.7817014562875,43.7797934107269,
44.7778853651663,45.7759773196057,46.7740692740451,47.1238898038469),
 .UNSPECIFIED.);
#26864=B_SPLINE_CURVE_WITH_KNOTS('',3,(#450891,#450892,#450893,#450894,
#450895,#450896,#450897,#450898,#450899,#450900),.UNSPECIFIED.,.F.,.F.,
(4,1,1,1,1,1,1,4),(40.8407044966673,41.3484951629377,42.3465871173771,43.3446790718166,
44.342771026256,45.3408629806954,46.3389549351348,47.1238898038469),
 .UNSPECIFIED.);
#26865=B_SPLINE_CURVE_WITH_KNOTS('',3,(#450905,#450906,#450907,#450908,
#450909,#450910,#450911,#450912,#450913,#450914,#450915),.UNSPECIFIED.,
 .F.,.F.,(4,1,1,1,1,1,1,1,4),(34.5575191894877,34.7969658207721,35.7950577752115,
36.7931497296509,37.7912416840904,38.7893336385298,39.7874255929692,40.7855175474086,
40.8407044966673),.UNSPECIFIED.);
#26866=B_SPLINE_CURVE_WITH_KNOTS('',3,(#450916,#450917,#450918,#450919,
#450920,#450921,#450922,#450923,#450924,#450925),.UNSPECIFIED.,.F.,.F.,
(4,1,1,1,1,1,1,4),(34.5575191894877,35.3599434363012,36.3580353907406,37.35612734518,
38.3542192996195,39.3523112540589,40.3504032084983,40.8407044966673),
 .UNSPECIFIED.);
#26867=B_SPLINE_CURVE_WITH_KNOTS('',3,(#450930,#450931,#450932,#450933,
#450934,#450935,#450936,#450937,#450938,#450939),.UNSPECIFIED.,.F.,.F.,
(4,1,1,1,1,1,1,4),(28.2743338823081,28.8084140941356,29.806506048575,30.8045980030144,
31.8026899574538,32.8007819118933,33.7988738663327,34.5575191894877),
 .UNSPECIFIED.);
#26868=B_SPLINE_CURVE_WITH_KNOTS('',3,(#450940,#450941,#450942,#450943,
#450944,#450945,#450946,#450947,#450948,#450949,#450950),.UNSPECIFIED.,
 .F.,.F.,(4,1,1,1,1,1,1,1,4),(28.2743338823081,28.3732997552253,29.3713917096647,
30.3694836641041,31.3675756185435,32.3656675729829,33.3637595274224,34.3618514818618,
34.5575191894877),.UNSPECIFIED.);
#26869=B_SPLINE_CURVE_WITH_KNOTS('',3,(#450955,#450956,#450957,#450958,
#450959,#450960,#450961,#450962,#450963,#450964),.UNSPECIFIED.,.F.,.F.,
(4,1,1,1,1,1,1,4),(21.9911485751285,22.8198623674991,23.8179543219385,24.8160462763779,
25.8141382308173,26.8122301852567,27.8103221396962,28.2743338823081),
 .UNSPECIFIED.);
#26870=B_SPLINE_CURVE_WITH_KNOTS('',3,(#450965,#450966,#450967,#450968,
#450969,#450970,#450971,#450972,#450973,#450974),.UNSPECIFIED.,.F.,.F.,
(4,1,1,1,1,1,1,4),(21.9911485751285,22.3847480285887,23.3828399830282,24.3809319374676,
25.379023891907,26.3771158463464,27.3752078007858,28.2743338823081),
 .UNSPECIFIED.);
#26871=B_SPLINE_CURVE_WITH_KNOTS('',3,(#450980,#450981,#450982,#450983,
#450984),.UNSPECIFIED.,.F.,.F.,(4,1,4),(14.4000123930734,15.3981043475128,
15.7079632679489),.UNSPECIFIED.);
#26872=B_SPLINE_CURVE_WITH_KNOTS('',3,(#450987,#450988,#450989,#450990,
#450991),.UNSPECIFIED.,.F.,.F.,(4,1,4),(13.8743214892347,14.8351267319837,
15.7079632679489),.UNSPECIFIED.);
#26873=B_SPLINE_CURVE_WITH_KNOTS('',3,(#450998,#450999,#451000,#451001,
#451002,#451003,#451004),.UNSPECIFIED.,.F.,.F.,(4,3,4),(-48.8692190558412,
-47.9084138130922,-47.8494095495406),.UNSPECIFIED.);
#26874=B_SPLINE_CURVE_WITH_KNOTS('',3,(#451010,#451011,#451012,#451013,
#451014,#451015,#451016,#451017,#451018,#451019,#451020,#451021,#451022,
#451023,#451024,#451025,#451026,#451027,#451028),.UNSPECIFIED.,.F.,.F.,
(4,3,3,3,3,3,4),(45.2902480251326,45.9122299042133,46.9103218586527,47.9084138130921,
48.9065057675316,49.904597721971,50.9026896764104),.UNSPECIFIED.);
#26875=B_SPLINE_CURVE_WITH_KNOTS('',3,(#451030,#451031,#451032,#451033,
#451034,#451035,#451036,#451037,#451038,#451039,#451040,#451041,#451042,
#451043,#451044,#451045,#451046,#451047,#451048,#451049,#451050,#451051),
 .UNSPECIFIED.,.F.,.F.,(4,3,3,3,3,3,3,4),(-47.8494095495406,-46.9103218586527,
-45.9122299042133,-44.9141379497739,-43.9160459953345,-42.9179540408951,
-41.9198620864556,-41.5662242423611),.UNSPECIFIED.);
#26876=B_SPLINE_CURVE_WITH_KNOTS('',3,(#451056,#451057,#451058,#451059,
#451060,#451061,#451062,#451063,#451064,#451065,#451066,#451067,#451068,
#451069,#451070,#451071,#451072,#451073,#451074,#451075,#451076,#451077),
 .UNSPECIFIED.,.F.,.F.,(4,3,3,3,3,3,3,4),(39.007062717953,39.9236781775768,
40.9217701320162,41.9198620864556,42.917954040895,43.9160459953345,44.9141379497739,
45.2902480251326),.UNSPECIFIED.);
#26877=B_SPLINE_CURVE_WITH_KNOTS('',3,(#451078,#451079,#451080,#451081,
#451082,#451083,#451084,#451085,#451086,#451087,#451088,#451089,#451090,
#451091,#451092,#451093,#451094,#451095,#451096,#451097,#451098,#451099),
 .UNSPECIFIED.,.F.,.F.,(4,3,3,3,3,3,3,4),(-41.5662242423611,-40.9217701320162,
-39.9236781775768,-38.9255862231374,-37.927494268698,-36.9294023142585,
-35.9313103598191,-35.2830389351814),.UNSPECIFIED.);
#26878=B_SPLINE_CURVE_WITH_KNOTS('',3,(#451104,#451105,#451106,#451107,
#451108,#451109,#451110,#451111,#451112,#451113,#451114,#451115,#451116,
#451117,#451118,#451119,#451120,#451121,#451122,#451123,#451124,#451125,
#451126,#451127,#451128),.UNSPECIFIED.,.F.,.F.,(4,3,3,3,3,3,3,3,4),(32.7238774107735,
32.9370344965008,33.9351264509403,34.9332184053797,35.9313103598191,36.9294023142585,
37.9274942686979,38.9255862231374,39.007062717953),.UNSPECIFIED.);
#26879=B_SPLINE_CURVE_WITH_KNOTS('',3,(#451129,#451130,#451131,#451132,
#451133,#451134,#451135,#451136,#451137,#451138,#451139,#451140,#451141,
#451142,#451143,#451144,#451145,#451146,#451147,#451148,#451149,#451150),
 .UNSPECIFIED.,.F.,.F.,(4,3,3,3,3,3,3,4),(-35.2830389351814,-34.9332184053797,
-33.9351264509403,-32.9370344965009,-31.9389425420614,-30.940850587622,
-29.9427586331826,-28.9998536280018),.UNSPECIFIED.);
#26880=B_SPLINE_CURVE_WITH_KNOTS('',3,(#451155,#451156,#451157,#451158,
#451159,#451160,#451161,#451162,#451163,#451164,#451165,#451166,#451167,
#451168,#451169,#451170,#451171,#451172,#451173,#451174,#451175,#451176),
 .UNSPECIFIED.,.F.,.F.,(4,3,3,3,3,3,3,4),(26.4406921035939,26.9484827698643,
27.9465747243037,28.9446666787432,29.9427586331826,30.940850587622,31.9389425420614,
32.7238774107735),.UNSPECIFIED.);
#26881=B_SPLINE_CURVE_WITH_KNOTS('',3,(#451177,#451178,#451179,#451180,
#451181,#451182,#451183,#451184,#451185,#451186,#451187,#451188,#451189,
#451190,#451191,#451192,#451193,#451194,#451195,#451196,#451197,#451198,
#451199,#451200,#451201),.UNSPECIFIED.,.F.,.F.,(4,3,3,3,3,3,3,3,4),(-28.9998536280018,
-28.9446666787432,-27.9465747243038,-26.9484827698643,-25.9503908154249,
-24.9522988609855,-23.9542069065461,-22.9561149521067,-22.7166683208223),
 .UNSPECIFIED.);
#26882=B_SPLINE_CURVE_WITH_KNOTS('',3,(#451206,#451207,#451208,#451209,
#451210,#451211,#451212,#451213,#451214,#451215,#451216,#451217,#451218,
#451219,#451220,#451221,#451222,#451223,#451224,#451225,#451226,#451227),
 .UNSPECIFIED.,.F.,.F.,(4,3,3,3,3,3,3,4),(20.1575067964143,20.9599310432278,
21.9580229976672,22.9561149521067,23.9542069065461,24.9522988609855,25.9503908154249,
26.4406921035939),.UNSPECIFIED.);
#26883=B_SPLINE_CURVE_WITH_KNOTS('',3,(#451228,#451229,#451230,#451231,
#451232,#451233,#451234,#451235,#451236,#451237,#451238,#451239,#451240,
#451241,#451242,#451243,#451244,#451245,#451246,#451247,#451248,#451249),
 .UNSPECIFIED.,.F.,.F.,(4,3,3,3,3,3,3,4),(-22.7166683208223,-21.9580229976672,
-20.9599310432278,-19.9618390887884,-18.963747134349,-17.9656551799096,
-16.9675632254701,-16.4334830136427),.UNSPECIFIED.);
#26884=B_SPLINE_CURVE_WITH_KNOTS('',3,(#451254,#451255,#451256,#451257,
#451258,#451259,#451260,#451261,#451262,#451263,#451264,#451265,#451266,
#451267,#451268,#451269,#451270,#451271,#451272,#451273,#451274,#451275,
#451276,#451277,#451278),.UNSPECIFIED.,.F.,.F.,(4,3,3,3,3,3,3,3,4),(13.8743214892347,
13.9732873621519,14.9713793165913,15.9694712710307,16.9675632254701,17.9656551799096,
18.963747134349,19.9618390887884,20.1575067964143),.UNSPECIFIED.);
#26885=B_SPLINE_CURVE_WITH_KNOTS('',3,(#451279,#451280,#451281,#451282,
#451283,#451284,#451285,#451286,#451287,#451288,#451289,#451290,#451291,
#451292,#451293,#451294,#451295,#451296,#451297,#451298,#451299,#451300),
 .UNSPECIFIED.,.F.,.F.,(4,3,3,3,3,3,3,4),(-16.4334830136427,-15.9694712710307,
-14.9713793165913,-13.9732873621519,-12.9751954077125,-11.977103453273,
-10.9790114988336,-10.1502977064631),.UNSPECIFIED.);
#26886=B_SPLINE_CURVE_WITH_KNOTS('',3,(#451306,#451307,#451308,#451309,
#451310,#451311,#451312,#451313,#451314,#451315,#451316,#451317,#451318),
 .UNSPECIFIED.,.F.,.F.,(4,3,3,3,4),(-3.86711239928348,-2.99427586331826,
-1.99618390887884,-0.998091954439421,0.),.UNSPECIFIED.);
#26887=B_SPLINE_CURVE_WITH_KNOTS('',3,(#451321,#451322,#451323,#451324,
#451325,#451326,#451327,#451328,#451329,#451330,#451331,#451332,#451333,
#451334,#451335,#451336,#451337,#451338,#451339),.UNSPECIFIED.,.F.,.F.,
(4,3,3,3,3,3,4),(2.03347062056922,2.99427586331826,3.99236781775768,4.9904597721971,
5.98855172663652,6.98664368107594,7.59113618205511),.UNSPECIFIED.);
#26888=B_SPLINE_CURVE_WITH_KNOTS('',3,(#451345,#451346,#451347,#451348,
#451349,#451350,#451351),.UNSPECIFIED.,.F.,.F.,(4,1,1,1,4),(59.6902604182061,
59.7492646817576,60.747356636197,61.7454485906364,62.7435405450759),
 .UNSPECIFIED.);
#26889=B_SPLINE_CURVE_WITH_KNOTS('',3,(#451354,#451355,#451356,#451357,
#451358,#451359,#451360),.UNSPECIFIED.,.F.,.F.,(4,1,1,1,4),(59.6902604182061,
60.3122422972867,61.3103342517261,62.3084262061655,63.2692314489146),
 .UNSPECIFIED.);
#26890=B_SPLINE_CURVE_WITH_KNOTS('',3,(#451365,#451366,#451367,#451368,
#451369,#451370,#451371,#451372,#451373,#451374),.UNSPECIFIED.,.F.,.F.,
(4,1,1,1,1,1,1,4),(53.4070751110265,53.7607129551211,54.7588049095605,55.7568968639999,
56.7549888184393,57.7530807728788,58.7511727273182,59.6902604182061),
 .UNSPECIFIED.);
#26891=B_SPLINE_CURVE_WITH_KNOTS('',3,(#451375,#451376,#451377,#451378,
#451379,#451380,#451381,#451382,#451383,#451384),.UNSPECIFIED.,.F.,.F.,
(4,1,1,1,1,1,1,4),(53.4070751110265,54.3236905706502,55.3217825250896,56.319874479529,
57.3179664339684,58.3160583884079,59.3141503428473,59.6902604182061),
 .UNSPECIFIED.);
#26892=B_SPLINE_CURVE_WITH_KNOTS('',3,(#451389,#451390,#451391,#451392,
#451393,#451394,#451395,#451396,#451397,#451398),.UNSPECIFIED.,.F.,.F.,
(4,1,1,1,1,1,1,4),(47.1238898038469,47.7721612284846,48.770253182924,49.7683451373634,
50.7664370918028,51.7645290462422,52.7626210006817,53.4070751110265),
 .UNSPECIFIED.);
#26893=B_SPLINE_CURVE_WITH_KNOTS('',3,(#451399,#451400,#451401,#451402,
#451403,#451404,#451405,#451406,#451407,#451408,#451409),.UNSPECIFIED.,
 .F.,.F.,(4,1,1,1,1,1,1,1,4),(47.1238898038469,47.3370468895742,48.3351388440137,
49.3332307984531,50.3313227528925,51.3294147073319,52.3275066617713,53.3255986162108,
53.4070751110265),.UNSPECIFIED.);
#26894=B_SPLINE_CURVE_WITH_KNOTS('',3,(#451414,#451415,#451416,#451417,
#451418,#451419,#451420,#451421,#451422,#451423),.UNSPECIFIED.,.F.,.F.,
(4,1,1,1,1,1,1,4),(40.8407044966673,41.783609501848,42.7817014562875,43.7797934107269,
44.7778853651663,45.7759773196057,46.7740692740451,47.1238898038469),
 .UNSPECIFIED.);
#26895=B_SPLINE_CURVE_WITH_KNOTS('',3,(#451424,#451425,#451426,#451427,
#451428,#451429,#451430,#451431,#451432,#451433),.UNSPECIFIED.,.F.,.F.,
(4,1,1,1,1,1,1,4),(40.8407044966673,41.3484951629377,42.3465871173771,43.3446790718166,
44.342771026256,45.3408629806954,46.3389549351348,47.1238898038469),
 .UNSPECIFIED.);
#26896=B_SPLINE_CURVE_WITH_KNOTS('',3,(#451438,#451439,#451440,#451441,
#451442,#451443,#451444,#451445,#451446,#451447,#451448),.UNSPECIFIED.,
 .F.,.F.,(4,1,1,1,1,1,1,1,4),(34.5575191894877,34.7969658207721,35.7950577752115,
36.7931497296509,37.7912416840904,38.7893336385298,39.7874255929692,40.7855175474086,
40.8407044966673),.UNSPECIFIED.);
#26897=B_SPLINE_CURVE_WITH_KNOTS('',3,(#451449,#451450,#451451,#451452,
#451453,#451454,#451455,#451456,#451457,#451458),.UNSPECIFIED.,.F.,.F.,
(4,1,1,1,1,1,1,4),(34.5575191894877,35.3599434363012,36.3580353907406,37.35612734518,
38.3542192996195,39.3523112540589,40.3504032084983,40.8407044966673),
 .UNSPECIFIED.);
#26898=B_SPLINE_CURVE_WITH_KNOTS('',3,(#451463,#451464,#451465,#451466,
#451467,#451468,#451469,#451470,#451471,#451472),.UNSPECIFIED.,.F.,.F.,
(4,1,1,1,1,1,1,4),(28.2743338823081,28.8084140941356,29.806506048575,30.8045980030144,
31.8026899574538,32.8007819118933,33.7988738663327,34.5575191894877),
 .UNSPECIFIED.);
#26899=B_SPLINE_CURVE_WITH_KNOTS('',3,(#451473,#451474,#451475,#451476,
#451477,#451478,#451479,#451480,#451481,#451482,#451483),.UNSPECIFIED.,
 .F.,.F.,(4,1,1,1,1,1,1,1,4),(28.2743338823081,28.3732997552253,29.3713917096647,
30.3694836641041,31.3675756185435,32.3656675729829,33.3637595274224,34.3618514818618,
34.5575191894877),.UNSPECIFIED.);
#26900=B_SPLINE_CURVE_WITH_KNOTS('',3,(#451488,#451489,#451490,#451491,
#451492,#451493,#451494,#451495,#451496,#451497),.UNSPECIFIED.,.F.,.F.,
(4,1,1,1,1,1,1,4),(21.9911485751285,22.8198623674991,23.8179543219385,24.8160462763779,
25.8141382308173,26.8122301852567,27.8103221396962,28.2743338823081),
 .UNSPECIFIED.);
#26901=B_SPLINE_CURVE_WITH_KNOTS('',3,(#451498,#451499,#451500,#451501,
#451502,#451503,#451504,#451505,#451506,#451507),.UNSPECIFIED.,.F.,.F.,
(4,1,1,1,1,1,1,4),(21.9911485751285,22.3847480285887,23.3828399830282,24.3809319374676,
25.379023891907,26.3771158463464,27.3752078007858,28.2743338823081),
 .UNSPECIFIED.);
#26902=B_SPLINE_CURVE_WITH_KNOTS('',3,(#451513,#451514,#451515,#451516,
#451517),.UNSPECIFIED.,.F.,.F.,(4,1,4),(14.4000123930734,15.3981043475128,
15.7079632679489),.UNSPECIFIED.);
#26903=B_SPLINE_CURVE_WITH_KNOTS('',3,(#451520,#451521,#451522,#451523,
#451524),.UNSPECIFIED.,.F.,.F.,(4,1,4),(13.8743214892347,14.8351267319837,
15.7079632679489),.UNSPECIFIED.);
#26904=B_SPLINE_CURVE_WITH_KNOTS('',3,(#451540,#451541,#451542,#451543,
#451544,#451545,#451546,#451547,#451548,#451549,#451550,#451551,#451552,
#451553,#451554,#451555,#451556,#451557,#451558,#451559,#451560,#451561,
#451562,#451563,#451564,#451565,#451566,#451567,#451568,#451569,#451570,
#451571,#451572,#451573,#451574,#451575,#451576,#451577,#451578,#451579,
#451580,#451581,#451582,#451583,#451584,#451585,#451586,#451587,#451588,
#451589,#451590,#451591,#451592,#451593,#451594,#451595,#451596,#451597,
#451598,#451599,#451600,#451601,#451602,#451603,#451604,#451605,#451606,
#451607,#451608,#451609,#451610,#451611,#451612,#451613,#451614,#451615,
#451616,#451617,#451618),.UNSPECIFIED.,.F.,.F.,(4,3,3,3,3,3,3,3,3,3,3,3,
3,3,3,3,3,3,3,3,3,3,3,3,3,3,4),(0.,0.0157320924267747,0.0316472886091288,
0.043157780198946,0.0480880250790969,0.0511356327252552,0.0665923147581226,
0.0816964235607721,0.0922051230024958,0.0959158625638971,0.0986562987241478,
0.113270482254995,0.123731221327667,0.137671787499722,0.141347701639905,
0.14411982558934,0.15865675060424,0.173153963373766,0.180916686790059,0.184948756264495,
0.18803730480951,0.201934721427929,0.211309428016589,0.21535636816053,0.228670816766457,
0.235255750704108,0.23917877492942),.UNSPECIFIED.);
#26905=B_SPLINE_CURVE_WITH_KNOTS('',3,(#451619,#451620,#451621,#451622,
#451623,#451624,#451625,#451626,#451627,#451628,#451629,#451630,#451631,
#451632,#451633,#451634,#451635,#451636,#451637,#451638,#451639,#451640,
#451641,#451642,#451643,#451644,#451645,#451646,#451647,#451648,#451649,
#451650,#451651,#451652,#451653,#451654,#451655,#451656,#451657,#451658,
#451659,#451660,#451661,#451662,#451663,#451664,#451665,#451666,#451667,
#451668,#451669,#451670,#451671,#451672,#451673,#451674,#451675,#451676,
#451677,#451678,#451679,#451680,#451681,#451682,#451683,#451684,#451685,
#451686,#451687,#451688,#451689,#451690,#451691,#451692,#451693,#451694,
#451695,#451696,#451697),.UNSPECIFIED.,.F.,.F.,(4,3,3,3,3,3,3,3,3,3,3,3,
3,3,3,3,3,3,3,3,3,3,3,3,3,3,4),(0.,0.0130352311543815,0.0266669283949033,
0.0371674278206855,0.0406547610952736,0.0430558088931652,0.057131904576132,
0.0714875682820563,0.0812834071618324,0.0840733481352456,0.0867292191258407,
0.101529760808593,0.110670923801161,0.125085624608173,0.128310240996154,
0.131025696331468,0.145800277836723,0.160944486485529,0.169985276581641,
0.174963947365941,0.177680096517495,0.193348287176511,0.204022641009529,
0.208963013854378,0.224845444526331,0.233270807254426,0.238077416065722),
 .UNSPECIFIED.);
#26906=B_SPLINE_CURVE_WITH_KNOTS('',3,(#451698,#451699,#451700,#451701,
#451702,#451703,#451704,#451705,#451706,#451707,#451708,#451709,#451710,
#451711,#451712,#451713,#451714,#451715,#451716,#451717,#451718,#451719,
#451720,#451721,#451722,#451723,#451724,#451725,#451726,#451727,#451728,
#451729,#451730,#451731,#451732,#451733,#451734,#451735,#451736,#451737,
#451738,#451739,#451740,#451741,#451742,#451743,#451744,#451745,#451746,
#451747,#451748,#451749,#451750,#451751,#451752,#451753,#451754,#451755,
#451756,#451757,#451758,#451759,#451760,#451761,#451762,#451763,#451764,
#451765,#451766,#451767,#451768,#451769,#451770,#451771,#451772,#451773,
#451774,#451775,#451776),.UNSPECIFIED.,.F.,.F.,(4,3,3,3,3,3,3,3,3,3,3,3,
3,3,3,3,3,3,3,3,3,3,3,3,3,3,4),(0.,0.0157320924267752,0.0316472886090957,
0.0431577801989171,0.0480880250790769,0.0511356327253695,0.0665923147581514,
0.0816964235608268,0.0922051230025368,0.0959158625640407,0.0986562987234703,
0.113270482254332,0.123731221327667,0.137671787499722,0.141347701639849,
0.144119825587372,0.158656750602193,0.173153963371847,0.180916686788379,
0.184948756260439,0.188037304808125,0.201934721426646,0.211309428014682,
0.215356368159481,0.228670816765373,0.235255750704108,0.23917877492942),
 .UNSPECIFIED.);
#26907=B_SPLINE_CURVE_WITH_KNOTS('',3,(#451777,#451778,#451779,#451780,
#451781,#451782,#451783,#451784,#451785,#451786,#451787,#451788,#451789,
#451790,#451791,#451792,#451793,#451794,#451795,#451796,#451797,#451798,
#451799,#451800,#451801,#451802,#451803,#451804,#451805,#451806,#451807,
#451808,#451809,#451810,#451811,#451812,#451813,#451814,#451815,#451816,
#451817,#451818,#451819,#451820,#451821,#451822,#451823,#451824,#451825,
#451826,#451827,#451828,#451829,#451830,#451831,#451832,#451833,#451834,
#451835,#451836,#451837,#451838,#451839,#451840,#451841,#451842,#451843,
#451844,#451845,#451846,#451847,#451848,#451849,#451850,#451851,#451852,
#451853,#451854,#451855),.UNSPECIFIED.,.F.,.F.,(4,3,3,3,3,3,3,3,3,3,3,3,
3,3,3,3,3,3,3,3,3,3,3,3,3,3,4),(0.,0.0130352311543815,0.0266669283949033,
0.0371674278206855,0.0406547610952736,0.0430558088931652,0.057131904576132,
0.0714875682820563,0.0812834071618324,0.0840733481352456,0.0867292191258407,
0.101529760808593,0.110670923801161,0.125085624608173,0.128310240996154,
0.131025696331468,0.145800277836723,0.160944486485529,0.169985276581641,
0.174963947365941,0.177680096517495,0.193348287176511,0.204022641009529,
0.208963013854378,0.224845444526331,0.233270807254426,0.238077416065722),
 .UNSPECIFIED.);
#26908=B_SPLINE_CURVE_WITH_KNOTS('',3,(#451856,#451857,#451858,#451859,
#451860,#451861,#451862,#451863,#451864,#451865,#451866,#451867,#451868,
#451869,#451870,#451871,#451872,#451873,#451874,#451875,#451876,#451877,
#451878,#451879,#451880,#451881,#451882,#451883,#451884,#451885,#451886,
#451887,#451888,#451889,#451890,#451891,#451892,#451893,#451894,#451895,
#451896,#451897,#451898,#451899,#451900,#451901,#451902,#451903,#451904,
#451905,#451906,#451907,#451908,#451909,#451910,#451911,#451912,#451913,
#451914,#451915,#451916,#451917,#451918,#451919,#451920,#451921,#451922,
#451923,#451924,#451925,#451926,#451927,#451928,#451929,#451930,#451931,
#451932,#451933,#451934),.UNSPECIFIED.,.F.,.F.,(4,3,3,3,3,3,3,3,3,3,3,3,
3,3,3,3,3,3,3,3,3,3,3,3,3,3,4),(0.,0.0157320924267737,0.0316472886090531,
0.0431577801988798,0.0480880250789605,0.0511356327296043,0.0665923147621861,
0.081696423564749,0.0922051230054785,0.0959158625863417,0.098656298737445,
0.113270482268115,0.123731221327667,0.137671787499722,0.141347701639876,
0.144119825589662,0.1586567506045,0.173153963374121,0.18091668679037,0.184948756264717,
0.188037304802666,0.201934721421039,0.211309428006616,0.215356368156104,
0.228670816762204,0.235255750704108,0.23917877492942),.UNSPECIFIED.);
#26909=B_SPLINE_CURVE_WITH_KNOTS('',3,(#451935,#451936,#451937,#451938,
#451939,#451940,#451941,#451942,#451943,#451944,#451945,#451946,#451947,
#451948,#451949,#451950,#451951,#451952,#451953,#451954,#451955,#451956,
#451957,#451958,#451959,#451960,#451961,#451962,#451963,#451964,#451965,
#451966,#451967,#451968,#451969,#451970,#451971,#451972,#451973,#451974,
#451975,#451976,#451977,#451978,#451979,#451980,#451981,#451982,#451983,
#451984,#451985,#451986,#451987,#451988,#451989,#451990,#451991,#451992,
#451993,#451994,#451995,#451996,#451997,#451998,#451999,#452000,#452001,
#452002,#452003,#452004,#452005,#452006,#452007,#452008,#452009,#452010,
#452011,#452012,#452013),.UNSPECIFIED.,.F.,.F.,(4,3,3,3,3,3,3,3,3,3,3,3,
3,3,3,3,3,3,3,3,3,3,3,3,3,3,4),(0.,0.0130352311543805,0.026666928394927,
0.0371674278207062,0.0406547610703887,0.0430558088506834,0.0571319045324971,
0.0714875682385721,0.0812834071292192,0.0840733479829169,0.0867292190991322,
0.101529760781986,0.110670923801161,0.125085624608173,0.128310241000168,
0.131025696331686,0.145800277836979,0.160944486485698,0.169985276581789,
0.1749639473661,0.177680096519024,0.193348287178018,0.20402264101174,0.208963013855492,
0.224845444527478,0.233270807254426,0.238077416065722),.UNSPECIFIED.);
#26910=B_SPLINE_CURVE_WITH_KNOTS('',3,(#452014,#452015,#452016,#452017,
#452018,#452019,#452020,#452021,#452022,#452023,#452024,#452025,#452026,
#452027,#452028,#452029,#452030,#452031,#452032,#452033,#452034,#452035,
#452036,#452037,#452038,#452039,#452040,#452041,#452042,#452043,#452044,
#452045,#452046,#452047,#452048,#452049,#452050,#452051,#452052,#452053,
#452054,#452055,#452056,#452057,#452058,#452059,#452060,#452061,#452062,
#452063,#452064,#452065,#452066,#452067,#452068,#452069,#452070,#452071,
#452072,#452073,#452074,#452075,#452076,#452077,#452078,#452079,#452080,
#452081,#452082,#452083,#452084,#452085,#452086,#452087,#452088,#452089,
#452090,#452091,#452092),.UNSPECIFIED.,.F.,.F.,(4,3,3,3,3,3,3,3,3,3,3,3,
3,3,3,3,3,3,3,3,3,3,3,3,3,3,4),(0.,0.0157320924267737,0.0316472886090531,
0.0431577801988798,0.0480880250789605,0.0511356327296043,0.0665923147621861,
0.081696423564749,0.0922051230054785,0.0959158625863417,0.098656298737445,
0.113270482268115,0.123731221327667,0.137671787499722,0.141347701639876,
0.144119825589662,0.1586567506045,0.173153963374121,0.18091668679037,0.184948756264717,
0.188037304802666,0.201934721421039,0.211309428006616,0.215356368156104,
0.228670816762204,0.235255750704108,0.23917877492942),.UNSPECIFIED.);
#26911=B_SPLINE_CURVE_WITH_KNOTS('',3,(#452093,#452094,#452095,#452096,
#452097,#452098,#452099,#452100,#452101,#452102,#452103,#452104,#452105,
#452106,#452107,#452108,#452109,#452110,#452111,#452112,#452113,#452114,
#452115,#452116,#452117,#452118,#452119,#452120,#452121,#452122,#452123,
#452124,#452125,#452126,#452127,#452128,#452129,#452130,#452131,#452132,
#452133,#452134,#452135,#452136,#452137,#452138,#452139,#452140,#452141,
#452142,#452143,#452144,#452145,#452146,#452147,#452148,#452149,#452150,
#452151,#452152,#452153,#452154,#452155,#452156,#452157,#452158,#452159,
#452160,#452161,#452162,#452163,#452164,#452165,#452166,#452167,#452168,
#452169,#452170,#452171),.UNSPECIFIED.,.F.,.F.,(4,3,3,3,3,3,3,3,3,3,3,3,
3,3,3,3,3,3,3,3,3,3,3,3,3,3,4),(0.,0.0130352311543801,0.026666928394903,
0.0371674278206852,0.0406547610767215,0.0430558088631254,0.057131904545114,
0.0714875682511512,0.0812834071386536,0.0840733480328551,0.0867292191078698,
0.101529760790684,0.110670923801161,0.125085624608172,0.128310241001407,
0.131025696334341,0.145800277839661,0.160944486488484,0.169985276584227,
0.174963947370384,0.177680096527197,0.193348287186297,0.204022641023147,
0.208963013858931,0.224845444530877,0.233270807254426,0.238077416065722),
 .UNSPECIFIED.);
#26912=B_SPLINE_CURVE_WITH_KNOTS('',3,(#452173,#452174,#452175,#452176,
#452177,#452178,#452179,#452180,#452181,#452182,#452183),.UNSPECIFIED.,
 .F.,.F.,(4,1,1,1,1,1,1,1,4),(15.7079632679489,15.8332186864231,16.8313106408625,
17.829402595302,18.8274945497414,19.8255865041808,20.8236784586202,21.8217704130596,
21.9911485751285),.UNSPECIFIED.);
#26913=B_SPLINE_CURVE_WITH_KNOTS('',3,(#452184,#452185,#452186,#452187,
#452188,#452189,#452190,#452191,#452192,#452193),.UNSPECIFIED.,.F.,.F.,
(4,1,1,1,1,1,1,4),(15.7079632679489,16.3961963019522,17.3942882563917,18.3923802108311,
19.3904721652705,20.3885641197099,21.3866560741493,21.9911485751285),
 .UNSPECIFIED.);
#26914=B_SPLINE_CURVE_WITH_KNOTS('',3,(#452410,#452411,#452412,#452413,
#452414,#452415,#452416,#452417,#452418,#452419,#452420,#452421,#452422,
#452423,#452424,#452425,#452426,#452427,#452428,#452429,#452430,#452431,
#452432,#452433,#452434,#452435,#452436,#452437,#452438,#452439,#452440,
#452441,#452442,#452443,#452444,#452445,#452446,#452447,#452448,#452449,
#452450,#452451,#452452,#452453,#452454,#452455,#452456,#452457,#452458,
#452459,#452460,#452461,#452462,#452463,#452464,#452465,#452466,#452467,
#452468,#452469,#452470,#452471,#452472,#452473,#452474,#452475,#452476,
#452477,#452478,#452479,#452480,#452481,#452482,#452483,#452484,#452485,
#452486,#452487,#452488),.UNSPECIFIED.,.F.,.F.,(4,3,3,3,3,3,3,3,3,3,3,3,
3,3,3,3,3,3,3,3,3,3,3,3,3,3,4),(0.,0.0157320931414714,0.0316472893339854,
0.0431577808331959,0.0480880269721251,0.0511356325173917,0.0665923145021214,
0.081696422951762,0.0922051225457388,0.0959158592594865,0.0986562961493802,
0.113270479382768,0.123731221327669,0.137671787499727,0.141347701391183,
0.144119825431661,0.158656750491721,0.173153963159623,0.180916686602687,
0.184948755241336,0.188037304397269,0.201934720592235,0.211309426632634,
0.215356367558587,0.228670815451418,0.235255750704128,0.239178774929437),
 .UNSPECIFIED.);
#26915=B_SPLINE_CURVE_WITH_KNOTS('',3,(#452489,#452490,#452491,#452492,
#452493,#452494,#452495,#452496,#452497,#452498,#452499,#452500,#452501,
#452502,#452503,#452504,#452505,#452506,#452507,#452508,#452509,#452510,
#452511,#452512,#452513),.UNSPECIFIED.,.F.,.F.,(4,3,3,3,3,3,3,3,4),(-10.1502977064631,
-9.9809195443942,-8.98282758995478,-7.98473563551536,-6.98664368107594,
-5.98855172663652,-4.9904597721971,-3.99236781775768,-3.86711239928348),
 .UNSPECIFIED.);
#26916=B_SPLINE_CURVE_WITH_KNOTS('',3,(#452730,#452731,#452732,#452733,
#452734,#452735,#452736,#452737,#452738,#452739,#452740,#452741,#452742,
#452743,#452744,#452745,#452746,#452747,#452748,#452749,#452750,#452751,
#452752,#452753,#452754,#452755,#452756,#452757,#452758,#452759,#452760,
#452761,#452762,#452763,#452764,#452765,#452766,#452767,#452768,#452769,
#452770,#452771,#452772,#452773,#452774,#452775,#452776,#452777,#452778,
#452779,#452780,#452781,#452782,#452783,#452784,#452785,#452786,#452787,
#452788,#452789,#452790,#452791,#452792,#452793,#452794,#452795,#452796,
#452797,#452798,#452799,#452800,#452801,#452802,#452803,#452804,#452805,
#452806,#452807,#452808),.UNSPECIFIED.,.F.,.F.,(4,3,3,3,3,3,3,3,3,3,3,3,
3,3,3,3,3,3,3,3,3,3,3,3,3,3,4),(0.,0.0130352298242541,0.0266669261176872,
0.0371674258281218,0.0406547814925501,0.0430558447319413,0.0571319404399593,
0.0714876040892006,0.0812834340171916,0.0840734593866279,0.0867292385757745,
0.101529780369819,0.110670923801164,0.125085625301101,0.128310245101767,
0.131025701128335,0.145800283575492,0.160944492677408,0.169985281999537,
0.174963957321762,0.177680109845532,0.193348300597375,0.204022660000448,
0.208963012593868,0.224845443267828,0.233270807254441,0.238077416065717),
 .UNSPECIFIED.);
#26917=B_SPLINE_CURVE_WITH_KNOTS('',3,(#452809,#452810,#452811,#452812,
#452813,#452814,#452815,#452816,#452817,#452818,#452819,#452820,#452821,
#452822,#452823,#452824,#452825,#452826,#452827,#452828,#452829,#452830),
 .UNSPECIFIED.,.F.,.F.,(4,3,3,3,3,3,3,4),(7.59113618205511,7.98473563551536,
8.98282758995478,9.9809195443942,10.9790114988336,11.977103453273,12.9751954077125,
13.8743214892347),.UNSPECIFIED.);
#26918=B_SPLINE_CURVE_WITH_KNOTS('',3,(#452834,#452835,#452836,#452837,
#452838,#452839,#452840,#452841,#452842,#452843,#452844,#452845,#452846,
#452847,#452848,#452849,#452850,#452851,#452852,#452853,#452854,#452855,
#452856,#452857,#452858,#452859,#452860,#452861,#452862,#452863,#452864,
#452865,#452866,#452867,#452868,#452869,#452870,#452871,#452872,#452873,
#452874,#452875,#452876,#452877,#452878,#452879,#452880,#452881,#452882,
#452883,#452884,#452885,#452886,#452887,#452888,#452889,#452890,#452891,
#452892,#452893,#452894,#452895,#452896,#452897,#452898,#452899,#452900,
#452901,#452902,#452903,#452904,#452905,#452906,#452907,#452908,#452909,
#452910,#452911,#452912),.UNSPECIFIED.,.F.,.F.,(4,3,3,3,3,3,3,3,3,3,3,3,
3,3,3,3,3,3,3,3,3,3,3,3,3,3,4),(0.,0.0157320931414709,0.0316472893341372,
0.0431577808333288,0.0480880269725141,0.0511356325307602,0.0665923145154681,
0.081696422964954,0.0922051225556328,0.0959158593335102,0.0986562962157222,
0.113270479448293,0.123731221327669,0.137671787499727,0.141347701390983,
0.144119825446287,0.158656750506384,0.173153963174152,0.180916686615399,
0.184948755270777,0.18803730441128,0.201934720606637,0.211309426653049,
0.215356367562411,0.228670815455102,0.235255750704128,0.239178774929437),
 .UNSPECIFIED.);
#26919=B_SPLINE_CURVE_WITH_KNOTS('',3,(#452913,#452914,#452915,#452916,
#452917,#452918,#452919,#452920,#452921,#452922,#452923,#452924,#452925,
#452926,#452927,#452928,#452929,#452930,#452931,#452932,#452933,#452934,
#452935,#452936,#452937,#452938,#452939,#452940,#452941,#452942,#452943,
#452944,#452945,#452946,#452947,#452948,#452949,#452950,#452951,#452952,
#452953,#452954,#452955,#452956,#452957,#452958,#452959,#452960,#452961,
#452962,#452963,#452964,#452965,#452966,#452967,#452968,#452969,#452970,
#452971,#452972,#452973,#452974,#452975,#452976,#452977,#452978,#452979,
#452980,#452981,#452982,#452983,#452984,#452985,#452986,#452987,#452988,
#452989,#452990,#452991),.UNSPECIFIED.,.F.,.F.,(4,3,3,3,3,3,3,3,3,3,3,3,
3,3,3,3,3,3,3,3,3,3,3,3,3,3,4),(0.,0.0130352298242513,0.0266669261174319,
0.0371674258278985,0.0406547813928594,0.0430558445655346,0.057131940264528,
0.0714876039142613,0.0812834338859871,0.0840734588472805,0.0867292384812191,
0.101529780275389,0.110670923801164,0.125085625301103,0.12831024509547,
0.131025701136019,0.145800283582927,0.160944492684684,0.169985282005903,
0.174963957332129,0.17768010985427,0.193348300606252,0.20402266001364,0.208963012602614,
0.224845443276616,0.233270807254441,0.238077416065717),.UNSPECIFIED.);
#26920=B_SPLINE_CURVE_WITH_KNOTS('',3,(#452992,#452993,#452994,#452995,
#452996,#452997,#452998,#452999,#453000,#453001,#453002,#453003,#453004,
#453005,#453006,#453007,#453008,#453009,#453010,#453011,#453012,#453013,
#453014,#453015,#453016,#453017,#453018,#453019,#453020,#453021,#453022,
#453023,#453024,#453025,#453026,#453027,#453028,#453029,#453030,#453031,
#453032,#453033,#453034,#453035,#453036,#453037,#453038,#453039,#453040,
#453041,#453042,#453043,#453044,#453045,#453046,#453047,#453048,#453049,
#453050,#453051,#453052,#453053,#453054,#453055,#453056,#453057,#453058,
#453059,#453060,#453061,#453062,#453063,#453064,#453065,#453066,#453067,
#453068,#453069,#453070),.UNSPECIFIED.,.F.,.F.,(4,3,3,3,3,3,3,3,3,3,3,3,
3,3,3,3,3,3,3,3,3,3,3,3,3,3,4),(0.,0.015732093141471,0.0316472893339033,
0.0431577808331241,0.0480880269716089,0.0511356325101152,0.066592314495774,
0.0816964229456337,0.0922051225411426,0.0959158592248474,0.0986562961367495,
0.113270479370498,0.123731221327669,0.137671787499727,0.141347701390887,
0.144119825427528,0.158656750487409,0.173153963155311,0.180916686598913,
0.184948755232054,0.18803730438579,0.201934720581443,0.211309426616656,
0.215356367553738,0.228670815447029,0.235255750704128,0.239178774929437),
 .UNSPECIFIED.);
#26921=B_SPLINE_CURVE_WITH_KNOTS('',3,(#453071,#453072,#453073,#453074,
#453075,#453076,#453077,#453078,#453079,#453080,#453081,#453082,#453083,
#453084,#453085,#453086,#453087,#453088,#453089,#453090,#453091,#453092,
#453093,#453094,#453095,#453096,#453097,#453098,#453099,#453100,#453101,
#453102,#453103,#453104,#453105,#453106,#453107,#453108,#453109,#453110,
#453111,#453112,#453113,#453114,#453115,#453116,#453117,#453118,#453119,
#453120,#453121,#453122,#453123,#453124,#453125,#453126,#453127,#453128,
#453129,#453130,#453131,#453132,#453133,#453134,#453135,#453136,#453137,
#453138,#453139,#453140,#453141,#453142,#453143,#453144,#453145,#453146,
#453147,#453148,#453149),.UNSPECIFIED.,.F.,.F.,(4,3,3,3,3,3,3,3,3,3,3,3,
3,3,3,3,3,3,3,3,3,3,3,3,3,3,4),(0.,0.0130352298242513,0.0266669261174319,
0.0371674258278985,0.0406547813928594,0.0430558445655346,0.057131940264528,
0.0714876039142613,0.0812834338859871,0.0840734588472805,0.0867292384812191,
0.101529780275389,0.110670923801164,0.125085625301103,0.12831024509547,
0.131025701136019,0.145800283582927,0.160944492684684,0.169985282005903,
0.174963957332129,0.17768010985427,0.193348300606252,0.20402266001364,0.208963012602614,
0.224845443276616,0.233270807254441,0.238077416065717),.UNSPECIFIED.);
#26922=B_SPLINE_CURVE_WITH_KNOTS('',3,(#453150,#453151,#453152,#453153,
#453154,#453155,#453156,#453157,#453158,#453159,#453160,#453161,#453162,
#453163,#453164,#453165,#453166,#453167,#453168,#453169,#453170,#453171,
#453172,#453173,#453174,#453175,#453176,#453177,#453178,#453179,#453180,
#453181,#453182,#453183,#453184,#453185,#453186,#453187,#453188,#453189,
#453190,#453191,#453192,#453193,#453194,#453195,#453196,#453197,#453198,
#453199,#453200,#453201,#453202,#453203,#453204,#453205,#453206,#453207,
#453208,#453209,#453210,#453211,#453212,#453213,#453214,#453215,#453216,
#453217,#453218,#453219,#453220,#453221,#453222,#453223,#453224,#453225,
#453226,#453227,#453228),.UNSPECIFIED.,.F.,.F.,(4,3,3,3,3,3,3,3,3,3,3,3,
3,3,3,3,3,3,3,3,3,3,3,3,3,3,4),(0.,0.0157320931414714,0.0316472893339854,
0.0431577808331959,0.0480880269721251,0.0511356325173917,0.0665923145021214,
0.081696422951762,0.0922051225457388,0.0959158592594865,0.0986562961493802,
0.113270479382768,0.123731221327669,0.137671787499727,0.141347701391183,
0.144119825431661,0.158656750491721,0.173153963159623,0.180916686602687,
0.184948755241336,0.188037304397269,0.201934720592235,0.211309426632634,
0.215356367558587,0.228670815451418,0.235255750704128,0.239178774929437),
 .UNSPECIFIED.);
#26923=B_SPLINE_CURVE_WITH_KNOTS('',3,(#453229,#453230,#453231,#453232,
#453233,#453234,#453235,#453236,#453237,#453238,#453239,#453240,#453241,
#453242,#453243,#453244,#453245,#453246,#453247,#453248,#453249,#453250,
#453251,#453252,#453253,#453254,#453255,#453256,#453257,#453258,#453259,
#453260,#453261,#453262,#453263,#453264,#453265,#453266,#453267,#453268,
#453269,#453270,#453271,#453272,#453273,#453274,#453275,#453276,#453277,
#453278,#453279,#453280,#453281,#453282,#453283,#453284,#453285,#453286,
#453287,#453288,#453289,#453290,#453291,#453292,#453293,#453294,#453295,
#453296,#453297,#453298,#453299,#453300,#453301,#453302,#453303,#453304,
#453305,#453306,#453307),.UNSPECIFIED.,.F.,.F.,(4,3,3,3,3,3,3,3,3,3,3,3,
3,3,3,3,3,3,3,3,3,3,3,3,3,3,4),(0.,0.0130352298242544,0.0266669261174456,
0.0371674258279105,0.0406547815148651,0.0430558447696239,0.0571319404770745,
0.0714876041258789,0.0812834340447003,0.0840734595031264,0.0867292385960914,
0.101529780390005,0.110670923801164,0.125085625301101,0.128310245110238,
0.131025701127911,0.14580028357443,0.160944492676094,0.169985281998388,
0.17496395731976,0.177680109834163,0.193348300586186,0.204022659984646,
0.208963012605258,0.224845443279121,0.233270807254441,0.238077416065717),
 .UNSPECIFIED.);
#26924=B_SPLINE_CURVE_WITH_KNOTS('',3,(#453460,#453461,#453462,#453463,
#453464,#453465,#453466,#453467,#453468,#453469,#453470),.UNSPECIFIED.,
 .F.,.F.,(4,1,1,1,1,1,1,1,4),(15.7079632679489,15.8332186864231,16.8313106408625,
17.829402595302,18.8274945497414,19.8255865041808,20.8236784586202,21.8217704130596,
21.9911485751285),.UNSPECIFIED.);
#26925=B_SPLINE_CURVE_WITH_KNOTS('',3,(#453471,#453472,#453473,#453474,
#453475,#453476,#453477,#453478,#453479,#453480),.UNSPECIFIED.,.F.,.F.,
(4,1,1,1,1,1,1,4),(15.7079632679489,16.3961963019522,17.3942882563917,18.3923802108311,
19.3904721652705,20.3885641197099,21.3866560741493,21.9911485751285),
 .UNSPECIFIED.);
#26926=B_SPLINE_CURVE_WITH_KNOTS('',3,(#453697,#453698,#453699,#453700,
#453701,#453702,#453703,#453704,#453705,#453706,#453707,#453708,#453709,
#453710,#453711,#453712,#453713,#453714,#453715,#453716,#453717,#453718,
#453719,#453720,#453721),.UNSPECIFIED.,.F.,.F.,(4,3,3,3,3,3,3,3,4),(-10.1502977064631,
-9.9809195443942,-8.98282758995478,-7.98473563551536,-6.98664368107594,
-5.98855172663652,-4.9904597721971,-3.99236781775768,-3.86711239928348),
 .UNSPECIFIED.);
#26927=B_SPLINE_CURVE_WITH_KNOTS('',3,(#453938,#453939,#453940,#453941,
#453942,#453943,#453944,#453945,#453946,#453947,#453948,#453949,#453950,
#453951,#453952,#453953,#453954,#453955,#453956,#453957,#453958,#453959),
 .UNSPECIFIED.,.F.,.F.,(4,3,3,3,3,3,3,4),(7.59113618205511,7.98473563551536,
8.98282758995478,9.9809195443942,10.9790114988336,11.977103453273,12.9751954077125,
13.8743214892347),.UNSPECIFIED.);
#26928=B_SPLINE_CURVE_WITH_KNOTS('',3,(#453962,#453963,#453964,#453965,
#453966,#453967,#453968,#453969,#453970,#453971,#453972),.UNSPECIFIED.,
 .F.,.F.,(4,1,1,1,1,1,1,1,4),(15.7079632679489,15.8332186864231,16.8313106408625,
17.829402595302,18.8274945497414,19.8255865041808,20.8236784586202,21.8217704130596,
21.9911485751285),.UNSPECIFIED.);
#26929=B_SPLINE_CURVE_WITH_KNOTS('',3,(#453973,#453974,#453975,#453976,
#453977,#453978,#453979,#453980,#453981,#453982),.UNSPECIFIED.,.F.,.F.,
(4,1,1,1,1,1,1,4),(15.7079632679489,16.3961963019522,17.3942882563917,18.3923802108311,
19.3904721652705,20.3885641197099,21.3866560741493,21.9911485751285),
 .UNSPECIFIED.);
#26930=B_SPLINE_CURVE_WITH_KNOTS('',3,(#454199,#454200,#454201,#454202,
#454203,#454204,#454205,#454206,#454207,#454208,#454209,#454210,#454211,
#454212,#454213,#454214,#454215,#454216,#454217,#454218,#454219,#454220,
#454221,#454222,#454223),.UNSPECIFIED.,.F.,.F.,(4,3,3,3,3,3,3,3,4),(-10.1502977064631,
-9.9809195443942,-8.98282758995478,-7.98473563551536,-6.98664368107594,
-5.98855172663652,-4.9904597721971,-3.99236781775768,-3.86711239928348),
 .UNSPECIFIED.);
#26931=B_SPLINE_CURVE_WITH_KNOTS('',3,(#454440,#454441,#454442,#454443,
#454444,#454445,#454446,#454447,#454448,#454449,#454450,#454451,#454452,
#454453,#454454,#454455,#454456,#454457,#454458,#454459,#454460,#454461),
 .UNSPECIFIED.,.F.,.F.,(4,3,3,3,3,3,3,4),(7.59113618205511,7.98473563551536,
8.98282758995478,9.9809195443942,10.9790114988336,11.977103453273,12.9751954077125,
13.8743214892347),.UNSPECIFIED.);
#26932=B_SPLINE_CURVE_WITH_KNOTS('',3,(#454464,#454465,#454466,#454467,
#454468,#454469,#454470,#454471,#454472,#454473,#454474),.UNSPECIFIED.,
 .F.,.F.,(4,1,1,1,1,1,1,1,4),(15.7079632679489,15.8332186864231,16.8313106408625,
17.829402595302,18.8274945497414,19.8255865041808,20.8236784586202,21.8217704130596,
21.9911485751285),.UNSPECIFIED.);
#26933=B_SPLINE_CURVE_WITH_KNOTS('',3,(#454475,#454476,#454477,#454478,
#454479,#454480,#454481,#454482,#454483,#454484),.UNSPECIFIED.,.F.,.F.,
(4,1,1,1,1,1,1,4),(15.7079632679489,16.3961963019522,17.3942882563917,18.3923802108311,
19.3904721652705,20.3885641197099,21.3866560741493,21.9911485751285),
 .UNSPECIFIED.);
#26934=B_SPLINE_CURVE_WITH_KNOTS('',3,(#454701,#454702,#454703,#454704,
#454705,#454706,#454707,#454708,#454709,#454710,#454711,#454712,#454713,
#454714,#454715,#454716,#454717,#454718,#454719,#454720,#454721,#454722,
#454723,#454724,#454725),.UNSPECIFIED.,.F.,.F.,(4,3,3,3,3,3,3,3,4),(-10.1502977064631,
-9.9809195443942,-8.98282758995478,-7.98473563551536,-6.98664368107594,
-5.98855172663652,-4.9904597721971,-3.99236781775768,-3.86711239928348),
 .UNSPECIFIED.);
#26935=B_SPLINE_CURVE_WITH_KNOTS('',3,(#454942,#454943,#454944,#454945,
#454946,#454947,#454948,#454949,#454950,#454951,#454952,#454953,#454954,
#454955,#454956,#454957,#454958,#454959,#454960,#454961,#454962,#454963),
 .UNSPECIFIED.,.F.,.F.,(4,3,3,3,3,3,3,4),(7.59113618205511,7.98473563551536,
8.98282758995478,9.9809195443942,10.9790114988336,11.977103453273,12.9751954077125,
13.8743214892347),.UNSPECIFIED.);
#30615=LINE('',#449396,#34417);
#30616=LINE('',#449409,#34418);
#30617=LINE('',#449456,#34419);
#30618=LINE('',#449504,#34420);
#30619=LINE('',#449555,#34421);
#30620=LINE('',#449606,#34422);
#30621=LINE('',#449654,#34423);
#30622=LINE('',#449705,#34424);
#30623=LINE('',#449744,#34425);
#30624=LINE('',#449765,#34426);
#30625=LINE('',#449789,#34427);
#30626=LINE('',#449814,#34428);
#30627=LINE('',#449838,#34429);
#30628=LINE('',#449863,#34430);
#30629=LINE('',#449888,#34431);
#30630=LINE('',#449912,#34432);
#30631=LINE('',#449929,#34433);
#30632=LINE('',#449942,#34434);
#30633=LINE('',#449989,#34435);
#30634=LINE('',#450037,#34436);
#30635=LINE('',#450088,#34437);
#30636=LINE('',#450139,#34438);
#30637=LINE('',#450187,#34439);
#30638=LINE('',#450238,#34440);
#30639=LINE('',#450277,#34441);
#30640=LINE('',#450298,#34442);
#30641=LINE('',#450322,#34443);
#30642=LINE('',#450347,#34444);
#30643=LINE('',#450371,#34445);
#30644=LINE('',#450396,#34446);
#30645=LINE('',#450421,#34447);
#30646=LINE('',#450445,#34448);
#30647=LINE('',#450462,#34449);
#30648=LINE('',#450475,#34450);
#30649=LINE('',#450522,#34451);
#30650=LINE('',#450570,#34452);
#30651=LINE('',#450621,#34453);
#30652=LINE('',#450672,#34454);
#30653=LINE('',#450720,#34455);
#30654=LINE('',#450771,#34456);
#30655=LINE('',#450810,#34457);
#30656=LINE('',#450831,#34458);
#30657=LINE('',#450855,#34459);
#30658=LINE('',#450880,#34460);
#30659=LINE('',#450904,#34461);
#30660=LINE('',#450929,#34462);
#30661=LINE('',#450954,#34463);
#30662=LINE('',#450978,#34464);
#30663=LINE('',#450995,#34465);
#30664=LINE('',#451008,#34466);
#30665=LINE('',#451055,#34467);
#30666=LINE('',#451103,#34468);
#30667=LINE('',#451154,#34469);
#30668=LINE('',#451205,#34470);
#30669=LINE('',#451253,#34471);
#30670=LINE('',#451304,#34472);
#30671=LINE('',#451343,#34473);
#30672=LINE('',#451364,#34474);
#30673=LINE('',#451388,#34475);
#30674=LINE('',#451413,#34476);
#30675=LINE('',#451437,#34477);
#30676=LINE('',#451462,#34478);
#30677=LINE('',#451487,#34479);
#30678=LINE('',#451511,#34480);
#30679=LINE('',#451529,#34481);
#30680=LINE('',#451536,#34482);
#30681=LINE('',#453315,#34483);
#30682=LINE('',#453319,#34484);
#30683=LINE('',#453323,#34485);
#30684=LINE('',#453328,#34486);
#30685=LINE('',#453331,#34487);
#30686=LINE('',#453336,#34488);
#30687=LINE('',#453341,#34489);
#30688=LINE('',#453347,#34490);
#30689=LINE('',#453353,#34491);
#30690=LINE('',#453359,#34492);
#30691=LINE('',#453365,#34493);
#30692=LINE('',#453371,#34494);
#30693=LINE('',#453377,#34495);
#30694=LINE('',#453383,#34496);
#30695=LINE('',#453389,#34497);
#30696=LINE('',#453395,#34498);
#30697=LINE('',#453401,#34499);
#30698=LINE('',#453407,#34500);
#30699=LINE('',#453413,#34501);
#30700=LINE('',#453419,#34502);
#30701=LINE('',#453425,#34503);
#30702=LINE('',#453431,#34504);
#30703=LINE('',#453437,#34505);
#34417=VECTOR('',#129689,1.25);
#34418=VECTOR('',#129694,1.25);
#34419=VECTOR('',#129699,1.25);
#34420=VECTOR('',#129702,1.25);
#34421=VECTOR('',#129705,1.25);
#34422=VECTOR('',#129708,1.25);
#34423=VECTOR('',#129711,1.25);
#34424=VECTOR('',#129714,1.25);
#34425=VECTOR('',#129719,1.29);
#34426=VECTOR('',#129724,1.29);
#34427=VECTOR('',#129727,1.29);
#34428=VECTOR('',#129730,1.29);
#34429=VECTOR('',#129733,1.29);
#34430=VECTOR('',#129736,1.29);
#34431=VECTOR('',#129739,1.29);
#34432=VECTOR('',#129742,1.29);
#34433=VECTOR('',#129747,1.25);
#34434=VECTOR('',#129752,1.25);
#34435=VECTOR('',#129757,1.25);
#34436=VECTOR('',#129760,1.25);
#34437=VECTOR('',#129763,1.25);
#34438=VECTOR('',#129766,1.25);
#34439=VECTOR('',#129769,1.25);
#34440=VECTOR('',#129772,1.25);
#34441=VECTOR('',#129777,1.29);
#34442=VECTOR('',#129782,1.29);
#34443=VECTOR('',#129785,1.29);
#34444=VECTOR('',#129788,1.29);
#34445=VECTOR('',#129791,1.29);
#34446=VECTOR('',#129794,1.29);
#34447=VECTOR('',#129797,1.29);
#34448=VECTOR('',#129800,1.29);
#34449=VECTOR('',#129805,1.25);
#34450=VECTOR('',#129810,1.25);
#34451=VECTOR('',#129815,1.25);
#34452=VECTOR('',#129818,1.25);
#34453=VECTOR('',#129821,1.25);
#34454=VECTOR('',#129824,1.25);
#34455=VECTOR('',#129827,1.25);
#34456=VECTOR('',#129830,1.25);
#34457=VECTOR('',#129835,1.29);
#34458=VECTOR('',#129840,1.29);
#34459=VECTOR('',#129843,1.29);
#34460=VECTOR('',#129846,1.29);
#34461=VECTOR('',#129849,1.29);
#34462=VECTOR('',#129852,1.29);
#34463=VECTOR('',#129855,1.29);
#34464=VECTOR('',#129858,1.29);
#34465=VECTOR('',#129863,1.25);
#34466=VECTOR('',#129868,1.25);
#34467=VECTOR('',#129873,1.25);
#34468=VECTOR('',#129876,1.25);
#34469=VECTOR('',#129879,1.25);
#34470=VECTOR('',#129882,1.25);
#34471=VECTOR('',#129885,1.25);
#34472=VECTOR('',#129888,1.25);
#34473=VECTOR('',#129893,1.29);
#34474=VECTOR('',#129898,1.29);
#34475=VECTOR('',#129901,1.29);
#34476=VECTOR('',#129904,1.29);
#34477=VECTOR('',#129907,1.29);
#34478=VECTOR('',#129910,1.29);
#34479=VECTOR('',#129913,1.29);
#34480=VECTOR('',#129916,1.29);
#34481=VECTOR('',#129923,2.25);
#34482=VECTOR('',#129932,2.1);
#34483=VECTOR('',#129951,11.15);
#34484=VECTOR('',#129956,1.99999999999997);
#34485=VECTOR('',#129961,3.5);
#34486=VECTOR('',#129968,11.15);
#34487=VECTOR('',#129971,11.15);
#34488=VECTOR('',#129978,4.95184441433916);
#34489=VECTOR('',#129983,11.15);
#34490=VECTOR('',#129990,5.08286386254677);
#34491=VECTOR('',#129997,11.15);
#34492=VECTOR('',#130004,5.21388331075437);
#34493=VECTOR('',#130011,11.15);
#34494=VECTOR('',#130018,5.34490275896198);
#34495=VECTOR('',#130025,11.15);
#34496=VECTOR('',#130032,5.47592220716958);
#34497=VECTOR('',#130039,11.15);
#34498=VECTOR('',#130046,5.60694165537719);
#34499=VECTOR('',#130053,11.15);
#34500=VECTOR('',#130060,5.73796110358479);
#34501=VECTOR('',#130067,11.15);
#34502=VECTOR('',#130074,5.8689805517924);
#34503=VECTOR('',#130081,11.15);
#34504=VECTOR('',#130088,6.);
#34505=VECTOR('',#130095,11.15);
#43111=VERTEX_POINT('',#449394);
#43112=VERTEX_POINT('',#449395);
#43113=VERTEX_POINT('',#449397);
#43114=VERTEX_POINT('',#449407);
#43115=VERTEX_POINT('',#449408);
#43116=VERTEX_POINT('',#449410);
#43117=VERTEX_POINT('',#449454);
#43118=VERTEX_POINT('',#449455);
#43119=VERTEX_POINT('',#449502);
#43120=VERTEX_POINT('',#449503);
#43121=VERTEX_POINT('',#449553);
#43122=VERTEX_POINT('',#449554);
#43123=VERTEX_POINT('',#449604);
#43124=VERTEX_POINT('',#449605);
#43125=VERTEX_POINT('',#449652);
#43126=VERTEX_POINT('',#449653);
#43127=VERTEX_POINT('',#449703);
#43128=VERTEX_POINT('',#449704);
#43129=VERTEX_POINT('',#449706);
#43130=VERTEX_POINT('',#449720);
#43131=VERTEX_POINT('',#449742);
#43132=VERTEX_POINT('',#449743);
#43133=VERTEX_POINT('',#449745);
#43134=VERTEX_POINT('',#449753);
#43135=VERTEX_POINT('',#449763);
#43136=VERTEX_POINT('',#449764);
#43137=VERTEX_POINT('',#449787);
#43138=VERTEX_POINT('',#449788);
#43139=VERTEX_POINT('',#449812);
#43140=VERTEX_POINT('',#449813);
#43141=VERTEX_POINT('',#449836);
#43142=VERTEX_POINT('',#449837);
#43143=VERTEX_POINT('',#449861);
#43144=VERTEX_POINT('',#449862);
#43145=VERTEX_POINT('',#449886);
#43146=VERTEX_POINT('',#449887);
#43147=VERTEX_POINT('',#449910);
#43148=VERTEX_POINT('',#449911);
#43149=VERTEX_POINT('',#449913);
#43150=VERTEX_POINT('',#449919);
#43151=VERTEX_POINT('',#449927);
#43152=VERTEX_POINT('',#449928);
#43153=VERTEX_POINT('',#449930);
#43154=VERTEX_POINT('',#449940);
#43155=VERTEX_POINT('',#449941);
#43156=VERTEX_POINT('',#449943);
#43157=VERTEX_POINT('',#449987);
#43158=VERTEX_POINT('',#449988);
#43159=VERTEX_POINT('',#450035);
#43160=VERTEX_POINT('',#450036);
#43161=VERTEX_POINT('',#450086);
#43162=VERTEX_POINT('',#450087);
#43163=VERTEX_POINT('',#450137);
#43164=VERTEX_POINT('',#450138);
#43165=VERTEX_POINT('',#450185);
#43166=VERTEX_POINT('',#450186);
#43167=VERTEX_POINT('',#450236);
#43168=VERTEX_POINT('',#450237);
#43169=VERTEX_POINT('',#450239);
#43170=VERTEX_POINT('',#450253);
#43171=VERTEX_POINT('',#450275);
#43172=VERTEX_POINT('',#450276);
#43173=VERTEX_POINT('',#450278);
#43174=VERTEX_POINT('',#450286);
#43175=VERTEX_POINT('',#450296);
#43176=VERTEX_POINT('',#450297);
#43177=VERTEX_POINT('',#450320);
#43178=VERTEX_POINT('',#450321);
#43179=VERTEX_POINT('',#450345);
#43180=VERTEX_POINT('',#450346);
#43181=VERTEX_POINT('',#450369);
#43182=VERTEX_POINT('',#450370);
#43183=VERTEX_POINT('',#450394);
#43184=VERTEX_POINT('',#450395);
#43185=VERTEX_POINT('',#450419);
#43186=VERTEX_POINT('',#450420);
#43187=VERTEX_POINT('',#450443);
#43188=VERTEX_POINT('',#450444);
#43189=VERTEX_POINT('',#450446);
#43190=VERTEX_POINT('',#450452);
#43191=VERTEX_POINT('',#450460);
#43192=VERTEX_POINT('',#450461);
#43193=VERTEX_POINT('',#450463);
#43194=VERTEX_POINT('',#450473);
#43195=VERTEX_POINT('',#450474);
#43196=VERTEX_POINT('',#450476);
#43197=VERTEX_POINT('',#450520);
#43198=VERTEX_POINT('',#450521);
#43199=VERTEX_POINT('',#450568);
#43200=VERTEX_POINT('',#450569);
#43201=VERTEX_POINT('',#450619);
#43202=VERTEX_POINT('',#450620);
#43203=VERTEX_POINT('',#450670);
#43204=VERTEX_POINT('',#450671);
#43205=VERTEX_POINT('',#450718);
#43206=VERTEX_POINT('',#450719);
#43207=VERTEX_POINT('',#450769);
#43208=VERTEX_POINT('',#450770);
#43209=VERTEX_POINT('',#450772);
#43210=VERTEX_POINT('',#450786);
#43211=VERTEX_POINT('',#450808);
#43212=VERTEX_POINT('',#450809);
#43213=VERTEX_POINT('',#450811);
#43214=VERTEX_POINT('',#450819);
#43215=VERTEX_POINT('',#450829);
#43216=VERTEX_POINT('',#450830);
#43217=VERTEX_POINT('',#450853);
#43218=VERTEX_POINT('',#450854);
#43219=VERTEX_POINT('',#450878);
#43220=VERTEX_POINT('',#450879);
#43221=VERTEX_POINT('',#450902);
#43222=VERTEX_POINT('',#450903);
#43223=VERTEX_POINT('',#450927);
#43224=VERTEX_POINT('',#450928);
#43225=VERTEX_POINT('',#450952);
#43226=VERTEX_POINT('',#450953);
#43227=VERTEX_POINT('',#450976);
#43228=VERTEX_POINT('',#450977);
#43229=VERTEX_POINT('',#450979);
#43230=VERTEX_POINT('',#450985);
#43231=VERTEX_POINT('',#450993);
#43232=VERTEX_POINT('',#450994);
#43233=VERTEX_POINT('',#450996);
#43234=VERTEX_POINT('',#451006);
#43235=VERTEX_POINT('',#451007);
#43236=VERTEX_POINT('',#451009);
#43237=VERTEX_POINT('',#451053);
#43238=VERTEX_POINT('',#451054);
#43239=VERTEX_POINT('',#451101);
#43240=VERTEX_POINT('',#451102);
#43241=VERTEX_POINT('',#451152);
#43242=VERTEX_POINT('',#451153);
#43243=VERTEX_POINT('',#451203);
#43244=VERTEX_POINT('',#451204);
#43245=VERTEX_POINT('',#451251);
#43246=VERTEX_POINT('',#451252);
#43247=VERTEX_POINT('',#451302);
#43248=VERTEX_POINT('',#451303);
#43249=VERTEX_POINT('',#451305);
#43250=VERTEX_POINT('',#451319);
#43251=VERTEX_POINT('',#451341);
#43252=VERTEX_POINT('',#451342);
#43253=VERTEX_POINT('',#451344);
#43254=VERTEX_POINT('',#451352);
#43255=VERTEX_POINT('',#451362);
#43256=VERTEX_POINT('',#451363);
#43257=VERTEX_POINT('',#451386);
#43258=VERTEX_POINT('',#451387);
#43259=VERTEX_POINT('',#451411);
#43260=VERTEX_POINT('',#451412);
#43261=VERTEX_POINT('',#451435);
#43262=VERTEX_POINT('',#451436);
#43263=VERTEX_POINT('',#451460);
#43264=VERTEX_POINT('',#451461);
#43265=VERTEX_POINT('',#451485);
#43266=VERTEX_POINT('',#451486);
#43267=VERTEX_POINT('',#451509);
#43268=VERTEX_POINT('',#451510);
#43269=VERTEX_POINT('',#451512);
#43270=VERTEX_POINT('',#451518);
#43271=VERTEX_POINT('',#451526);
#43272=VERTEX_POINT('',#451528);
#43273=VERTEX_POINT('',#451532);
#43274=VERTEX_POINT('',#451533);
#43275=VERTEX_POINT('',#451538);
#43276=VERTEX_POINT('',#452832);
#43277=VERTEX_POINT('',#453308);
#43278=VERTEX_POINT('',#453312);
#43279=VERTEX_POINT('',#453314);
#43280=VERTEX_POINT('',#453318);
#43281=VERTEX_POINT('',#453322);
#43282=VERTEX_POINT('',#453326);
#43283=VERTEX_POINT('',#453330);
#43284=VERTEX_POINT('',#453334);
#43285=VERTEX_POINT('',#453338);
#43286=VERTEX_POINT('',#453340);
#43287=VERTEX_POINT('',#453344);
#43288=VERTEX_POINT('',#453346);
#43289=VERTEX_POINT('',#453350);
#43290=VERTEX_POINT('',#453352);
#43291=VERTEX_POINT('',#453356);
#43292=VERTEX_POINT('',#453358);
#43293=VERTEX_POINT('',#453362);
#43294=VERTEX_POINT('',#453364);
#43295=VERTEX_POINT('',#453368);
#43296=VERTEX_POINT('',#453370);
#43297=VERTEX_POINT('',#453374);
#43298=VERTEX_POINT('',#453376);
#43299=VERTEX_POINT('',#453380);
#43300=VERTEX_POINT('',#453382);
#43301=VERTEX_POINT('',#453386);
#43302=VERTEX_POINT('',#453388);
#43303=VERTEX_POINT('',#453392);
#43304=VERTEX_POINT('',#453394);
#43305=VERTEX_POINT('',#453398);
#43306=VERTEX_POINT('',#453400);
#43307=VERTEX_POINT('',#453404);
#43308=VERTEX_POINT('',#453406);
#43309=VERTEX_POINT('',#453410);
#43310=VERTEX_POINT('',#453412);
#43311=VERTEX_POINT('',#453416);
#43312=VERTEX_POINT('',#453418);
#43313=VERTEX_POINT('',#453422);
#43314=VERTEX_POINT('',#453424);
#43315=VERTEX_POINT('',#453428);
#43316=VERTEX_POINT('',#453430);
#43317=VERTEX_POINT('',#453434);
#43318=VERTEX_POINT('',#453436);
#57403=EDGE_CURVE('',#43111,#43112,#30615,.T.);
#57404=EDGE_CURVE('',#43113,#43112,#23374,.T.);
#57405=EDGE_CURVE('',#43113,#43111,#26780,.T.);
#57406=EDGE_CURVE('',#43114,#43115,#30616,.T.);
#57407=EDGE_CURVE('',#43115,#43116,#26781,.T.);
#57408=EDGE_CURVE('',#43112,#43116,#23375,.T.);
#57409=EDGE_CURVE('',#43111,#43114,#26782,.T.);
#57410=EDGE_CURVE('',#43117,#43118,#30617,.T.);
#57411=EDGE_CURVE('',#43118,#43115,#26783,.T.);
#57412=EDGE_CURVE('',#43114,#43117,#26784,.T.);
#57413=EDGE_CURVE('',#43119,#43120,#30618,.T.);
#57414=EDGE_CURVE('',#43120,#43118,#26785,.T.);
#57415=EDGE_CURVE('',#43117,#43119,#26786,.T.);
#57416=EDGE_CURVE('',#43121,#43122,#30619,.T.);
#57417=EDGE_CURVE('',#43122,#43120,#26787,.T.);
#57418=EDGE_CURVE('',#43119,#43121,#26788,.T.);
#57419=EDGE_CURVE('',#43123,#43124,#30620,.T.);
#57420=EDGE_CURVE('',#43124,#43122,#26789,.T.);
#57421=EDGE_CURVE('',#43121,#43123,#26790,.T.);
#57422=EDGE_CURVE('',#43125,#43126,#30621,.T.);
#57423=EDGE_CURVE('',#43126,#43124,#26791,.T.);
#57424=EDGE_CURVE('',#43123,#43125,#26792,.T.);
#57425=EDGE_CURVE('',#43127,#43128,#30622,.T.);
#57426=EDGE_CURVE('',#43127,#43129,#26793,.T.);
#57427=EDGE_CURVE('',#43130,#43129,#23376,.T.);
#57428=EDGE_CURVE('',#43130,#43128,#26794,.T.);
#57429=EDGE_CURVE('',#43131,#43132,#30623,.T.);
#57430=EDGE_CURVE('',#43132,#43133,#26795,.T.);
#57431=EDGE_CURVE('',#43134,#43133,#23377,.T.);
#57432=EDGE_CURVE('',#43131,#43134,#26796,.T.);
#57433=EDGE_CURVE('',#43135,#43136,#30624,.T.);
#57434=EDGE_CURVE('',#43136,#43132,#26797,.T.);
#57435=EDGE_CURVE('',#43135,#43131,#26798,.T.);
#57436=EDGE_CURVE('',#43137,#43138,#30625,.T.);
#57437=EDGE_CURVE('',#43138,#43136,#26799,.T.);
#57438=EDGE_CURVE('',#43137,#43135,#26800,.T.);
#57439=EDGE_CURVE('',#43139,#43140,#30626,.T.);
#57440=EDGE_CURVE('',#43140,#43138,#26801,.T.);
#57441=EDGE_CURVE('',#43139,#43137,#26802,.T.);
#57442=EDGE_CURVE('',#43141,#43142,#30627,.T.);
#57443=EDGE_CURVE('',#43142,#43140,#26803,.T.);
#57444=EDGE_CURVE('',#43141,#43139,#26804,.T.);
#57445=EDGE_CURVE('',#43143,#43144,#30628,.T.);
#57446=EDGE_CURVE('',#43144,#43142,#26805,.T.);
#57447=EDGE_CURVE('',#43143,#43141,#26806,.T.);
#57448=EDGE_CURVE('',#43145,#43146,#30629,.T.);
#57449=EDGE_CURVE('',#43146,#43144,#26807,.T.);
#57450=EDGE_CURVE('',#43145,#43143,#26808,.T.);
#57451=EDGE_CURVE('',#43147,#43148,#30630,.T.);
#57452=EDGE_CURVE('',#43149,#43147,#26809,.T.);
#57453=EDGE_CURVE('',#43150,#43149,#23378,.T.);
#57454=EDGE_CURVE('',#43150,#43148,#26810,.T.);
#57455=EDGE_CURVE('',#43151,#43152,#30631,.T.);
#57456=EDGE_CURVE('',#43153,#43152,#23379,.T.);
#57457=EDGE_CURVE('',#43153,#43151,#26811,.T.);
#57458=EDGE_CURVE('',#43154,#43155,#30632,.T.);
#57459=EDGE_CURVE('',#43155,#43156,#26812,.T.);
#57460=EDGE_CURVE('',#43152,#43156,#23380,.T.);
#57461=EDGE_CURVE('',#43151,#43154,#26813,.T.);
#57462=EDGE_CURVE('',#43157,#43158,#30633,.T.);
#57463=EDGE_CURVE('',#43158,#43155,#26814,.T.);
#57464=EDGE_CURVE('',#43154,#43157,#26815,.T.);
#57465=EDGE_CURVE('',#43159,#43160,#30634,.T.);
#57466=EDGE_CURVE('',#43160,#43158,#26816,.T.);
#57467=EDGE_CURVE('',#43157,#43159,#26817,.T.);
#57468=EDGE_CURVE('',#43161,#43162,#30635,.T.);
#57469=EDGE_CURVE('',#43162,#43160,#26818,.T.);
#57470=EDGE_CURVE('',#43159,#43161,#26819,.T.);
#57471=EDGE_CURVE('',#43163,#43164,#30636,.T.);
#57472=EDGE_CURVE('',#43164,#43162,#26820,.T.);
#57473=EDGE_CURVE('',#43161,#43163,#26821,.T.);
#57474=EDGE_CURVE('',#43165,#43166,#30637,.T.);
#57475=EDGE_CURVE('',#43166,#43164,#26822,.T.);
#57476=EDGE_CURVE('',#43163,#43165,#26823,.T.);
#57477=EDGE_CURVE('',#43167,#43168,#30638,.T.);
#57478=EDGE_CURVE('',#43167,#43169,#26824,.T.);
#57479=EDGE_CURVE('',#43170,#43169,#23381,.T.);
#57480=EDGE_CURVE('',#43170,#43168,#26825,.T.);
#57481=EDGE_CURVE('',#43171,#43172,#30639,.T.);
#57482=EDGE_CURVE('',#43172,#43173,#26826,.T.);
#57483=EDGE_CURVE('',#43174,#43173,#23382,.T.);
#57484=EDGE_CURVE('',#43171,#43174,#26827,.T.);
#57485=EDGE_CURVE('',#43175,#43176,#30640,.T.);
#57486=EDGE_CURVE('',#43176,#43172,#26828,.T.);
#57487=EDGE_CURVE('',#43175,#43171,#26829,.T.);
#57488=EDGE_CURVE('',#43177,#43178,#30641,.T.);
#57489=EDGE_CURVE('',#43178,#43176,#26830,.T.);
#57490=EDGE_CURVE('',#43177,#43175,#26831,.T.);
#57491=EDGE_CURVE('',#43179,#43180,#30642,.T.);
#57492=EDGE_CURVE('',#43180,#43178,#26832,.T.);
#57493=EDGE_CURVE('',#43179,#43177,#26833,.T.);
#57494=EDGE_CURVE('',#43181,#43182,#30643,.T.);
#57495=EDGE_CURVE('',#43182,#43180,#26834,.T.);
#57496=EDGE_CURVE('',#43181,#43179,#26835,.T.);
#57497=EDGE_CURVE('',#43183,#43184,#30644,.T.);
#57498=EDGE_CURVE('',#43184,#43182,#26836,.T.);
#57499=EDGE_CURVE('',#43183,#43181,#26837,.T.);
#57500=EDGE_CURVE('',#43185,#43186,#30645,.T.);
#57501=EDGE_CURVE('',#43186,#43184,#26838,.T.);
#57502=EDGE_CURVE('',#43185,#43183,#26839,.T.);
#57503=EDGE_CURVE('',#43187,#43188,#30646,.T.);
#57504=EDGE_CURVE('',#43189,#43187,#26840,.T.);
#57505=EDGE_CURVE('',#43190,#43189,#23383,.T.);
#57506=EDGE_CURVE('',#43190,#43188,#26841,.T.);
#57507=EDGE_CURVE('',#43191,#43192,#30647,.T.);
#57508=EDGE_CURVE('',#43193,#43192,#23384,.T.);
#57509=EDGE_CURVE('',#43193,#43191,#26842,.T.);
#57510=EDGE_CURVE('',#43194,#43195,#30648,.T.);
#57511=EDGE_CURVE('',#43195,#43196,#26843,.T.);
#57512=EDGE_CURVE('',#43192,#43196,#23385,.T.);
#57513=EDGE_CURVE('',#43191,#43194,#26844,.T.);
#57514=EDGE_CURVE('',#43197,#43198,#30649,.T.);
#57515=EDGE_CURVE('',#43198,#43195,#26845,.T.);
#57516=EDGE_CURVE('',#43194,#43197,#26846,.T.);
#57517=EDGE_CURVE('',#43199,#43200,#30650,.T.);
#57518=EDGE_CURVE('',#43200,#43198,#26847,.T.);
#57519=EDGE_CURVE('',#43197,#43199,#26848,.T.);
#57520=EDGE_CURVE('',#43201,#43202,#30651,.T.);
#57521=EDGE_CURVE('',#43202,#43200,#26849,.T.);
#57522=EDGE_CURVE('',#43199,#43201,#26850,.T.);
#57523=EDGE_CURVE('',#43203,#43204,#30652,.T.);
#57524=EDGE_CURVE('',#43204,#43202,#26851,.T.);
#57525=EDGE_CURVE('',#43201,#43203,#26852,.T.);
#57526=EDGE_CURVE('',#43205,#43206,#30653,.T.);
#57527=EDGE_CURVE('',#43206,#43204,#26853,.T.);
#57528=EDGE_CURVE('',#43203,#43205,#26854,.T.);
#57529=EDGE_CURVE('',#43207,#43208,#30654,.T.);
#57530=EDGE_CURVE('',#43207,#43209,#26855,.T.);
#57531=EDGE_CURVE('',#43210,#43209,#23386,.T.);
#57532=EDGE_CURVE('',#43210,#43208,#26856,.T.);
#57533=EDGE_CURVE('',#43211,#43212,#30655,.T.);
#57534=EDGE_CURVE('',#43212,#43213,#26857,.T.);
#57535=EDGE_CURVE('',#43214,#43213,#23387,.T.);
#57536=EDGE_CURVE('',#43211,#43214,#26858,.T.);
#57537=EDGE_CURVE('',#43215,#43216,#30656,.T.);
#57538=EDGE_CURVE('',#43216,#43212,#26859,.T.);
#57539=EDGE_CURVE('',#43215,#43211,#26860,.T.);
#57540=EDGE_CURVE('',#43217,#43218,#30657,.T.);
#57541=EDGE_CURVE('',#43218,#43216,#26861,.T.);
#57542=EDGE_CURVE('',#43217,#43215,#26862,.T.);
#57543=EDGE_CURVE('',#43219,#43220,#30658,.T.);
#57544=EDGE_CURVE('',#43220,#43218,#26863,.T.);
#57545=EDGE_CURVE('',#43219,#43217,#26864,.T.);
#57546=EDGE_CURVE('',#43221,#43222,#30659,.T.);
#57547=EDGE_CURVE('',#43222,#43220,#26865,.T.);
#57548=EDGE_CURVE('',#43221,#43219,#26866,.T.);
#57549=EDGE_CURVE('',#43223,#43224,#30660,.T.);
#57550=EDGE_CURVE('',#43224,#43222,#26867,.T.);
#57551=EDGE_CURVE('',#43223,#43221,#26868,.T.);
#57552=EDGE_CURVE('',#43225,#43226,#30661,.T.);
#57553=EDGE_CURVE('',#43226,#43224,#26869,.T.);
#57554=EDGE_CURVE('',#43225,#43223,#26870,.T.);
#57555=EDGE_CURVE('',#43227,#43228,#30662,.T.);
#57556=EDGE_CURVE('',#43229,#43227,#26871,.T.);
#57557=EDGE_CURVE('',#43230,#43229,#23388,.T.);
#57558=EDGE_CURVE('',#43230,#43228,#26872,.T.);
#57559=EDGE_CURVE('',#43231,#43232,#30663,.T.);
#57560=EDGE_CURVE('',#43233,#43232,#23389,.T.);
#57561=EDGE_CURVE('',#43233,#43231,#26873,.T.);
#57562=EDGE_CURVE('',#43234,#43235,#30664,.T.);
#57563=EDGE_CURVE('',#43235,#43236,#26874,.T.);
#57564=EDGE_CURVE('',#43232,#43236,#23390,.T.);
#57565=EDGE_CURVE('',#43231,#43234,#26875,.T.);
#57566=EDGE_CURVE('',#43237,#43238,#30665,.T.);
#57567=EDGE_CURVE('',#43238,#43235,#26876,.T.);
#57568=EDGE_CURVE('',#43234,#43237,#26877,.T.);
#57569=EDGE_CURVE('',#43239,#43240,#30666,.T.);
#57570=EDGE_CURVE('',#43240,#43238,#26878,.T.);
#57571=EDGE_CURVE('',#43237,#43239,#26879,.T.);
#57572=EDGE_CURVE('',#43241,#43242,#30667,.T.);
#57573=EDGE_CURVE('',#43242,#43240,#26880,.T.);
#57574=EDGE_CURVE('',#43239,#43241,#26881,.T.);
#57575=EDGE_CURVE('',#43243,#43244,#30668,.T.);
#57576=EDGE_CURVE('',#43244,#43242,#26882,.T.);
#57577=EDGE_CURVE('',#43241,#43243,#26883,.T.);
#57578=EDGE_CURVE('',#43245,#43246,#30669,.T.);
#57579=EDGE_CURVE('',#43246,#43244,#26884,.T.);
#57580=EDGE_CURVE('',#43243,#43245,#26885,.T.);
#57581=EDGE_CURVE('',#43247,#43248,#30670,.T.);
#57582=EDGE_CURVE('',#43247,#43249,#26886,.T.);
#57583=EDGE_CURVE('',#43250,#43249,#23391,.T.);
#57584=EDGE_CURVE('',#43250,#43248,#26887,.T.);
#57585=EDGE_CURVE('',#43251,#43252,#30671,.T.);
#57586=EDGE_CURVE('',#43252,#43253,#26888,.T.);
#57587=EDGE_CURVE('',#43254,#43253,#23392,.T.);
#57588=EDGE_CURVE('',#43251,#43254,#26889,.T.);
#57589=EDGE_CURVE('',#43255,#43256,#30672,.T.);
#57590=EDGE_CURVE('',#43256,#43252,#26890,.T.);
#57591=EDGE_CURVE('',#43255,#43251,#26891,.T.);
#57592=EDGE_CURVE('',#43257,#43258,#30673,.T.);
#57593=EDGE_CURVE('',#43258,#43256,#26892,.T.);
#57594=EDGE_CURVE('',#43257,#43255,#26893,.T.);
#57595=EDGE_CURVE('',#43259,#43260,#30674,.T.);
#57596=EDGE_CURVE('',#43260,#43258,#26894,.T.);
#57597=EDGE_CURVE('',#43259,#43257,#26895,.T.);
#57598=EDGE_CURVE('',#43261,#43262,#30675,.T.);
#57599=EDGE_CURVE('',#43262,#43260,#26896,.T.);
#57600=EDGE_CURVE('',#43261,#43259,#26897,.T.);
#57601=EDGE_CURVE('',#43263,#43264,#30676,.T.);
#57602=EDGE_CURVE('',#43264,#43262,#26898,.T.);
#57603=EDGE_CURVE('',#43263,#43261,#26899,.T.);
#57604=EDGE_CURVE('',#43265,#43266,#30677,.T.);
#57605=EDGE_CURVE('',#43266,#43264,#26900,.T.);
#57606=EDGE_CURVE('',#43265,#43263,#26901,.T.);
#57607=EDGE_CURVE('',#43267,#43268,#30678,.T.);
#57608=EDGE_CURVE('',#43269,#43267,#26902,.T.);
#57609=EDGE_CURVE('',#43270,#43269,#23393,.T.);
#57610=EDGE_CURVE('',#43270,#43268,#26903,.T.);
#57611=EDGE_CURVE('',#43271,#43271,#23394,.T.);
#57612=EDGE_CURVE('',#43271,#43272,#30679,.T.);
#57613=EDGE_CURVE('',#43272,#43272,#23395,.T.);
#57614=EDGE_CURVE('',#43273,#43274,#23396,.T.);
#57615=EDGE_CURVE('',#43274,#43273,#23397,.T.);
#57616=EDGE_CURVE('',#43273,#43272,#30680,.T.);
#57617=EDGE_CURVE('',#43275,#43275,#23398,.T.);
#57618=EDGE_CURVE('',#43269,#43250,#26904,.T.);
#57619=EDGE_CURVE('',#43249,#43270,#26905,.T.);
#57620=EDGE_CURVE('',#43229,#43210,#26906,.T.);
#57621=EDGE_CURVE('',#43209,#43230,#26907,.T.);
#57622=EDGE_CURVE('',#43189,#43170,#26908,.T.);
#57623=EDGE_CURVE('',#43169,#43190,#26909,.T.);
#57624=EDGE_CURVE('',#43149,#43130,#26910,.T.);
#57625=EDGE_CURVE('',#43129,#43150,#26911,.T.);
#57626=EDGE_CURVE('',#43268,#43266,#26912,.T.);
#57627=EDGE_CURVE('',#43267,#43265,#26913,.T.);
#57628=EDGE_CURVE('',#43253,#43233,#26914,.T.);
#57629=EDGE_CURVE('',#43245,#43247,#26915,.T.);
#57630=EDGE_CURVE('',#43236,#43254,#26916,.T.);
#57631=EDGE_CURVE('',#43248,#43246,#26917,.T.);
#57632=EDGE_CURVE('',#43276,#43276,#23399,.F.);
#57633=EDGE_CURVE('',#43133,#43113,#26918,.T.);
#57634=EDGE_CURVE('',#43116,#43134,#26919,.T.);
#57635=EDGE_CURVE('',#43173,#43153,#26920,.T.);
#57636=EDGE_CURVE('',#43156,#43174,#26921,.T.);
#57637=EDGE_CURVE('',#43213,#43193,#26922,.T.);
#57638=EDGE_CURVE('',#43196,#43214,#26923,.T.);
#57639=EDGE_CURVE('',#43277,#43277,#23400,.T.);
#57640=EDGE_CURVE('',#43278,#43278,#23401,.T.);
#57641=EDGE_CURVE('',#43278,#43279,#30681,.T.);
#57642=EDGE_CURVE('',#43279,#43279,#23402,.T.);
#57643=EDGE_CURVE('',#43274,#43280,#30682,.T.);
#57644=EDGE_CURVE('',#43280,#43280,#23403,.T.);
#57645=EDGE_CURVE('',#43280,#43281,#30683,.T.);
#57646=EDGE_CURVE('',#43281,#43281,#23404,.T.);
#57647=EDGE_CURVE('',#43282,#43282,#23405,.F.);
#57648=EDGE_CURVE('',#43282,#43275,#30684,.T.);
#57649=EDGE_CURVE('',#43276,#43283,#30685,.T.);
#57650=EDGE_CURVE('',#43283,#43283,#23406,.T.);
#57651=EDGE_CURVE('',#43284,#43284,#23407,.T.);
#57652=EDGE_CURVE('',#43284,#43277,#30686,.T.);
#57653=EDGE_CURVE('',#43285,#43285,#23408,.F.);
#57654=EDGE_CURVE('',#43285,#43286,#30687,.T.);
#57655=EDGE_CURVE('',#43286,#43286,#23409,.T.);
#57656=EDGE_CURVE('',#43287,#43287,#23410,.T.);
#57657=EDGE_CURVE('',#43287,#43288,#30688,.T.);
#57658=EDGE_CURVE('',#43288,#43288,#23411,.T.);
#57659=EDGE_CURVE('',#43289,#43289,#23412,.F.);
#57660=EDGE_CURVE('',#43289,#43290,#30689,.T.);
#57661=EDGE_CURVE('',#43290,#43290,#23413,.T.);
#57662=EDGE_CURVE('',#43291,#43291,#23414,.T.);
#57663=EDGE_CURVE('',#43291,#43292,#30690,.T.);
#57664=EDGE_CURVE('',#43292,#43292,#23415,.T.);
#57665=EDGE_CURVE('',#43293,#43293,#23416,.F.);
#57666=EDGE_CURVE('',#43293,#43294,#30691,.T.);
#57667=EDGE_CURVE('',#43294,#43294,#23417,.T.);
#57668=EDGE_CURVE('',#43295,#43295,#23418,.T.);
#57669=EDGE_CURVE('',#43295,#43296,#30692,.T.);
#57670=EDGE_CURVE('',#43296,#43296,#23419,.T.);
#57671=EDGE_CURVE('',#43297,#43297,#23420,.F.);
#57672=EDGE_CURVE('',#43297,#43298,#30693,.T.);
#57673=EDGE_CURVE('',#43298,#43298,#23421,.T.);
#57674=EDGE_CURVE('',#43299,#43299,#23422,.T.);
#57675=EDGE_CURVE('',#43299,#43300,#30694,.T.);
#57676=EDGE_CURVE('',#43300,#43300,#23423,.T.);
#57677=EDGE_CURVE('',#43301,#43301,#23424,.F.);
#57678=EDGE_CURVE('',#43301,#43302,#30695,.T.);
#57679=EDGE_CURVE('',#43302,#43302,#23425,.T.);
#57680=EDGE_CURVE('',#43303,#43303,#23426,.T.);
#57681=EDGE_CURVE('',#43303,#43304,#30696,.T.);
#57682=EDGE_CURVE('',#43304,#43304,#23427,.T.);
#57683=EDGE_CURVE('',#43305,#43305,#23428,.F.);
#57684=EDGE_CURVE('',#43305,#43306,#30697,.T.);
#57685=EDGE_CURVE('',#43306,#43306,#23429,.T.);
#57686=EDGE_CURVE('',#43307,#43307,#23430,.T.);
#57687=EDGE_CURVE('',#43307,#43308,#30698,.T.);
#57688=EDGE_CURVE('',#43308,#43308,#23431,.T.);
#57689=EDGE_CURVE('',#43309,#43309,#23432,.F.);
#57690=EDGE_CURVE('',#43309,#43310,#30699,.T.);
#57691=EDGE_CURVE('',#43310,#43310,#23433,.T.);
#57692=EDGE_CURVE('',#43311,#43311,#23434,.T.);
#57693=EDGE_CURVE('',#43311,#43312,#30700,.T.);
#57694=EDGE_CURVE('',#43312,#43312,#23435,.T.);
#57695=EDGE_CURVE('',#43313,#43313,#23436,.F.);
#57696=EDGE_CURVE('',#43313,#43314,#30701,.T.);
#57697=EDGE_CURVE('',#43314,#43314,#23437,.T.);
#57698=EDGE_CURVE('',#43315,#43315,#23438,.T.);
#57699=EDGE_CURVE('',#43315,#43316,#30702,.T.);
#57700=EDGE_CURVE('',#43316,#43316,#23439,.T.);
#57701=EDGE_CURVE('',#43317,#43317,#23440,.F.);
#57702=EDGE_CURVE('',#43317,#43318,#30703,.T.);
#57703=EDGE_CURVE('',#43318,#43318,#23441,.T.);
#57704=EDGE_CURVE('',#43228,#43226,#26924,.T.);
#57705=EDGE_CURVE('',#43227,#43225,#26925,.T.);
#57706=EDGE_CURVE('',#43205,#43207,#26926,.T.);
#57707=EDGE_CURVE('',#43208,#43206,#26927,.T.);
#57708=EDGE_CURVE('',#43188,#43186,#26928,.T.);
#57709=EDGE_CURVE('',#43187,#43185,#26929,.T.);
#57710=EDGE_CURVE('',#43165,#43167,#26930,.T.);
#57711=EDGE_CURVE('',#43168,#43166,#26931,.T.);
#57712=EDGE_CURVE('',#43148,#43146,#26932,.T.);
#57713=EDGE_CURVE('',#43147,#43145,#26933,.T.);
#57714=EDGE_CURVE('',#43125,#43127,#26934,.T.);
#57715=EDGE_CURVE('',#43128,#43126,#26935,.T.);
#85802=ORIENTED_EDGE('',*,*,#57403,.T.);
#85803=ORIENTED_EDGE('',*,*,#57404,.F.);
#85804=ORIENTED_EDGE('',*,*,#57405,.T.);
#85805=ORIENTED_EDGE('',*,*,#57406,.T.);
#85806=ORIENTED_EDGE('',*,*,#57407,.T.);
#85807=ORIENTED_EDGE('',*,*,#57408,.F.);
#85808=ORIENTED_EDGE('',*,*,#57403,.F.);
#85809=ORIENTED_EDGE('',*,*,#57409,.T.);
#85810=ORIENTED_EDGE('',*,*,#57410,.T.);
#85811=ORIENTED_EDGE('',*,*,#57411,.T.);
#85812=ORIENTED_EDGE('',*,*,#57406,.F.);
#85813=ORIENTED_EDGE('',*,*,#57412,.T.);
#85814=ORIENTED_EDGE('',*,*,#57413,.T.);
#85815=ORIENTED_EDGE('',*,*,#57414,.T.);
#85816=ORIENTED_EDGE('',*,*,#57410,.F.);
#85817=ORIENTED_EDGE('',*,*,#57415,.T.);
#85818=ORIENTED_EDGE('',*,*,#57416,.T.);
#85819=ORIENTED_EDGE('',*,*,#57417,.T.);
#85820=ORIENTED_EDGE('',*,*,#57413,.F.);
#85821=ORIENTED_EDGE('',*,*,#57418,.T.);
#85822=ORIENTED_EDGE('',*,*,#57419,.T.);
#85823=ORIENTED_EDGE('',*,*,#57420,.T.);
#85824=ORIENTED_EDGE('',*,*,#57416,.F.);
#85825=ORIENTED_EDGE('',*,*,#57421,.T.);
#85826=ORIENTED_EDGE('',*,*,#57422,.T.);
#85827=ORIENTED_EDGE('',*,*,#57423,.T.);
#85828=ORIENTED_EDGE('',*,*,#57419,.F.);
#85829=ORIENTED_EDGE('',*,*,#57424,.T.);
#85830=ORIENTED_EDGE('',*,*,#57425,.F.);
#85831=ORIENTED_EDGE('',*,*,#57426,.T.);
#85832=ORIENTED_EDGE('',*,*,#57427,.F.);
#85833=ORIENTED_EDGE('',*,*,#57428,.T.);
#85834=ORIENTED_EDGE('',*,*,#57429,.T.);
#85835=ORIENTED_EDGE('',*,*,#57430,.T.);
#85836=ORIENTED_EDGE('',*,*,#57431,.F.);
#85837=ORIENTED_EDGE('',*,*,#57432,.F.);
#85838=ORIENTED_EDGE('',*,*,#57433,.T.);
#85839=ORIENTED_EDGE('',*,*,#57434,.T.);
#85840=ORIENTED_EDGE('',*,*,#57429,.F.);
#85841=ORIENTED_EDGE('',*,*,#57435,.F.);
#85842=ORIENTED_EDGE('',*,*,#57436,.T.);
#85843=ORIENTED_EDGE('',*,*,#57437,.T.);
#85844=ORIENTED_EDGE('',*,*,#57433,.F.);
#85845=ORIENTED_EDGE('',*,*,#57438,.F.);
#85846=ORIENTED_EDGE('',*,*,#57439,.T.);
#85847=ORIENTED_EDGE('',*,*,#57440,.T.);
#85848=ORIENTED_EDGE('',*,*,#57436,.F.);
#85849=ORIENTED_EDGE('',*,*,#57441,.F.);
#85850=ORIENTED_EDGE('',*,*,#57442,.T.);
#85851=ORIENTED_EDGE('',*,*,#57443,.T.);
#85852=ORIENTED_EDGE('',*,*,#57439,.F.);
#85853=ORIENTED_EDGE('',*,*,#57444,.F.);
#85854=ORIENTED_EDGE('',*,*,#57445,.T.);
#85855=ORIENTED_EDGE('',*,*,#57446,.T.);
#85856=ORIENTED_EDGE('',*,*,#57442,.F.);
#85857=ORIENTED_EDGE('',*,*,#57447,.F.);
#85858=ORIENTED_EDGE('',*,*,#57448,.T.);
#85859=ORIENTED_EDGE('',*,*,#57449,.T.);
#85860=ORIENTED_EDGE('',*,*,#57445,.F.);
#85861=ORIENTED_EDGE('',*,*,#57450,.F.);
#85862=ORIENTED_EDGE('',*,*,#57451,.F.);
#85863=ORIENTED_EDGE('',*,*,#57452,.F.);
#85864=ORIENTED_EDGE('',*,*,#57453,.F.);
#85865=ORIENTED_EDGE('',*,*,#57454,.T.);
#85866=ORIENTED_EDGE('',*,*,#57455,.T.);
#85867=ORIENTED_EDGE('',*,*,#57456,.F.);
#85868=ORIENTED_EDGE('',*,*,#57457,.T.);
#85869=ORIENTED_EDGE('',*,*,#57458,.T.);
#85870=ORIENTED_EDGE('',*,*,#57459,.T.);
#85871=ORIENTED_EDGE('',*,*,#57460,.F.);
#85872=ORIENTED_EDGE('',*,*,#57455,.F.);
#85873=ORIENTED_EDGE('',*,*,#57461,.T.);
#85874=ORIENTED_EDGE('',*,*,#57462,.T.);
#85875=ORIENTED_EDGE('',*,*,#57463,.T.);
#85876=ORIENTED_EDGE('',*,*,#57458,.F.);
#85877=ORIENTED_EDGE('',*,*,#57464,.T.);
#85878=ORIENTED_EDGE('',*,*,#57465,.T.);
#85879=ORIENTED_EDGE('',*,*,#57466,.T.);
#85880=ORIENTED_EDGE('',*,*,#57462,.F.);
#85881=ORIENTED_EDGE('',*,*,#57467,.T.);
#85882=ORIENTED_EDGE('',*,*,#57468,.T.);
#85883=ORIENTED_EDGE('',*,*,#57469,.T.);
#85884=ORIENTED_EDGE('',*,*,#57465,.F.);
#85885=ORIENTED_EDGE('',*,*,#57470,.T.);
#85886=ORIENTED_EDGE('',*,*,#57471,.T.);
#85887=ORIENTED_EDGE('',*,*,#57472,.T.);
#85888=ORIENTED_EDGE('',*,*,#57468,.F.);
#85889=ORIENTED_EDGE('',*,*,#57473,.T.);
#85890=ORIENTED_EDGE('',*,*,#57474,.T.);
#85891=ORIENTED_EDGE('',*,*,#57475,.T.);
#85892=ORIENTED_EDGE('',*,*,#57471,.F.);
#85893=ORIENTED_EDGE('',*,*,#57476,.T.);
#85894=ORIENTED_EDGE('',*,*,#57477,.F.);
#85895=ORIENTED_EDGE('',*,*,#57478,.T.);
#85896=ORIENTED_EDGE('',*,*,#57479,.F.);
#85897=ORIENTED_EDGE('',*,*,#57480,.T.);
#85898=ORIENTED_EDGE('',*,*,#57481,.T.);
#85899=ORIENTED_EDGE('',*,*,#57482,.T.);
#85900=ORIENTED_EDGE('',*,*,#57483,.F.);
#85901=ORIENTED_EDGE('',*,*,#57484,.F.);
#85902=ORIENTED_EDGE('',*,*,#57485,.T.);
#85903=ORIENTED_EDGE('',*,*,#57486,.T.);
#85904=ORIENTED_EDGE('',*,*,#57481,.F.);
#85905=ORIENTED_EDGE('',*,*,#57487,.F.);
#85906=ORIENTED_EDGE('',*,*,#57488,.T.);
#85907=ORIENTED_EDGE('',*,*,#57489,.T.);
#85908=ORIENTED_EDGE('',*,*,#57485,.F.);
#85909=ORIENTED_EDGE('',*,*,#57490,.F.);
#85910=ORIENTED_EDGE('',*,*,#57491,.T.);
#85911=ORIENTED_EDGE('',*,*,#57492,.T.);
#85912=ORIENTED_EDGE('',*,*,#57488,.F.);
#85913=ORIENTED_EDGE('',*,*,#57493,.F.);
#85914=ORIENTED_EDGE('',*,*,#57494,.T.);
#85915=ORIENTED_EDGE('',*,*,#57495,.T.);
#85916=ORIENTED_EDGE('',*,*,#57491,.F.);
#85917=ORIENTED_EDGE('',*,*,#57496,.F.);
#85918=ORIENTED_EDGE('',*,*,#57497,.T.);
#85919=ORIENTED_EDGE('',*,*,#57498,.T.);
#85920=ORIENTED_EDGE('',*,*,#57494,.F.);
#85921=ORIENTED_EDGE('',*,*,#57499,.F.);
#85922=ORIENTED_EDGE('',*,*,#57500,.T.);
#85923=ORIENTED_EDGE('',*,*,#57501,.T.);
#85924=ORIENTED_EDGE('',*,*,#57497,.F.);
#85925=ORIENTED_EDGE('',*,*,#57502,.F.);
#85926=ORIENTED_EDGE('',*,*,#57503,.F.);
#85927=ORIENTED_EDGE('',*,*,#57504,.F.);
#85928=ORIENTED_EDGE('',*,*,#57505,.F.);
#85929=ORIENTED_EDGE('',*,*,#57506,.T.);
#85930=ORIENTED_EDGE('',*,*,#57507,.T.);
#85931=ORIENTED_EDGE('',*,*,#57508,.F.);
#85932=ORIENTED_EDGE('',*,*,#57509,.T.);
#85933=ORIENTED_EDGE('',*,*,#57510,.T.);
#85934=ORIENTED_EDGE('',*,*,#57511,.T.);
#85935=ORIENTED_EDGE('',*,*,#57512,.F.);
#85936=ORIENTED_EDGE('',*,*,#57507,.F.);
#85937=ORIENTED_EDGE('',*,*,#57513,.T.);
#85938=ORIENTED_EDGE('',*,*,#57514,.T.);
#85939=ORIENTED_EDGE('',*,*,#57515,.T.);
#85940=ORIENTED_EDGE('',*,*,#57510,.F.);
#85941=ORIENTED_EDGE('',*,*,#57516,.T.);
#85942=ORIENTED_EDGE('',*,*,#57517,.T.);
#85943=ORIENTED_EDGE('',*,*,#57518,.T.);
#85944=ORIENTED_EDGE('',*,*,#57514,.F.);
#85945=ORIENTED_EDGE('',*,*,#57519,.T.);
#85946=ORIENTED_EDGE('',*,*,#57520,.T.);
#85947=ORIENTED_EDGE('',*,*,#57521,.T.);
#85948=ORIENTED_EDGE('',*,*,#57517,.F.);
#85949=ORIENTED_EDGE('',*,*,#57522,.T.);
#85950=ORIENTED_EDGE('',*,*,#57523,.T.);
#85951=ORIENTED_EDGE('',*,*,#57524,.T.);
#85952=ORIENTED_EDGE('',*,*,#57520,.F.);
#85953=ORIENTED_EDGE('',*,*,#57525,.T.);
#85954=ORIENTED_EDGE('',*,*,#57526,.T.);
#85955=ORIENTED_EDGE('',*,*,#57527,.T.);
#85956=ORIENTED_EDGE('',*,*,#57523,.F.);
#85957=ORIENTED_EDGE('',*,*,#57528,.T.);
#85958=ORIENTED_EDGE('',*,*,#57529,.F.);
#85959=ORIENTED_EDGE('',*,*,#57530,.T.);
#85960=ORIENTED_EDGE('',*,*,#57531,.F.);
#85961=ORIENTED_EDGE('',*,*,#57532,.T.);
#85962=ORIENTED_EDGE('',*,*,#57533,.T.);
#85963=ORIENTED_EDGE('',*,*,#57534,.T.);
#85964=ORIENTED_EDGE('',*,*,#57535,.F.);
#85965=ORIENTED_EDGE('',*,*,#57536,.F.);
#85966=ORIENTED_EDGE('',*,*,#57537,.T.);
#85967=ORIENTED_EDGE('',*,*,#57538,.T.);
#85968=ORIENTED_EDGE('',*,*,#57533,.F.);
#85969=ORIENTED_EDGE('',*,*,#57539,.F.);
#85970=ORIENTED_EDGE('',*,*,#57540,.T.);
#85971=ORIENTED_EDGE('',*,*,#57541,.T.);
#85972=ORIENTED_EDGE('',*,*,#57537,.F.);
#85973=ORIENTED_EDGE('',*,*,#57542,.F.);
#85974=ORIENTED_EDGE('',*,*,#57543,.T.);
#85975=ORIENTED_EDGE('',*,*,#57544,.T.);
#85976=ORIENTED_EDGE('',*,*,#57540,.F.);
#85977=ORIENTED_EDGE('',*,*,#57545,.F.);
#85978=ORIENTED_EDGE('',*,*,#57546,.T.);
#85979=ORIENTED_EDGE('',*,*,#57547,.T.);
#85980=ORIENTED_EDGE('',*,*,#57543,.F.);
#85981=ORIENTED_EDGE('',*,*,#57548,.F.);
#85982=ORIENTED_EDGE('',*,*,#57549,.T.);
#85983=ORIENTED_EDGE('',*,*,#57550,.T.);
#85984=ORIENTED_EDGE('',*,*,#57546,.F.);
#85985=ORIENTED_EDGE('',*,*,#57551,.F.);
#85986=ORIENTED_EDGE('',*,*,#57552,.T.);
#85987=ORIENTED_EDGE('',*,*,#57553,.T.);
#85988=ORIENTED_EDGE('',*,*,#57549,.F.);
#85989=ORIENTED_EDGE('',*,*,#57554,.F.);
#85990=ORIENTED_EDGE('',*,*,#57555,.F.);
#85991=ORIENTED_EDGE('',*,*,#57556,.F.);
#85992=ORIENTED_EDGE('',*,*,#57557,.F.);
#85993=ORIENTED_EDGE('',*,*,#57558,.T.);
#85994=ORIENTED_EDGE('',*,*,#57559,.T.);
#85995=ORIENTED_EDGE('',*,*,#57560,.F.);
#85996=ORIENTED_EDGE('',*,*,#57561,.T.);
#85997=ORIENTED_EDGE('',*,*,#57562,.T.);
#85998=ORIENTED_EDGE('',*,*,#57563,.T.);
#85999=ORIENTED_EDGE('',*,*,#57564,.F.);
#86000=ORIENTED_EDGE('',*,*,#57559,.F.);
#86001=ORIENTED_EDGE('',*,*,#57565,.T.);
#86002=ORIENTED_EDGE('',*,*,#57566,.T.);
#86003=ORIENTED_EDGE('',*,*,#57567,.T.);
#86004=ORIENTED_EDGE('',*,*,#57562,.F.);
#86005=ORIENTED_EDGE('',*,*,#57568,.T.);
#86006=ORIENTED_EDGE('',*,*,#57569,.T.);
#86007=ORIENTED_EDGE('',*,*,#57570,.T.);
#86008=ORIENTED_EDGE('',*,*,#57566,.F.);
#86009=ORIENTED_EDGE('',*,*,#57571,.T.);
#86010=ORIENTED_EDGE('',*,*,#57572,.T.);
#86011=ORIENTED_EDGE('',*,*,#57573,.T.);
#86012=ORIENTED_EDGE('',*,*,#57569,.F.);
#86013=ORIENTED_EDGE('',*,*,#57574,.T.);
#86014=ORIENTED_EDGE('',*,*,#57575,.T.);
#86015=ORIENTED_EDGE('',*,*,#57576,.T.);
#86016=ORIENTED_EDGE('',*,*,#57572,.F.);
#86017=ORIENTED_EDGE('',*,*,#57577,.T.);
#86018=ORIENTED_EDGE('',*,*,#57578,.T.);
#86019=ORIENTED_EDGE('',*,*,#57579,.T.);
#86020=ORIENTED_EDGE('',*,*,#57575,.F.);
#86021=ORIENTED_EDGE('',*,*,#57580,.T.);
#86022=ORIENTED_EDGE('',*,*,#57581,.F.);
#86023=ORIENTED_EDGE('',*,*,#57582,.T.);
#86024=ORIENTED_EDGE('',*,*,#57583,.F.);
#86025=ORIENTED_EDGE('',*,*,#57584,.T.);
#86026=ORIENTED_EDGE('',*,*,#57585,.T.);
#86027=ORIENTED_EDGE('',*,*,#57586,.T.);
#86028=ORIENTED_EDGE('',*,*,#57587,.F.);
#86029=ORIENTED_EDGE('',*,*,#57588,.F.);
#86030=ORIENTED_EDGE('',*,*,#57589,.T.);
#86031=ORIENTED_EDGE('',*,*,#57590,.T.);
#86032=ORIENTED_EDGE('',*,*,#57585,.F.);
#86033=ORIENTED_EDGE('',*,*,#57591,.F.);
#86034=ORIENTED_EDGE('',*,*,#57592,.T.);
#86035=ORIENTED_EDGE('',*,*,#57593,.T.);
#86036=ORIENTED_EDGE('',*,*,#57589,.F.);
#86037=ORIENTED_EDGE('',*,*,#57594,.F.);
#86038=ORIENTED_EDGE('',*,*,#57595,.T.);
#86039=ORIENTED_EDGE('',*,*,#57596,.T.);
#86040=ORIENTED_EDGE('',*,*,#57592,.F.);
#86041=ORIENTED_EDGE('',*,*,#57597,.F.);
#86042=ORIENTED_EDGE('',*,*,#57598,.T.);
#86043=ORIENTED_EDGE('',*,*,#57599,.T.);
#86044=ORIENTED_EDGE('',*,*,#57595,.F.);
#86045=ORIENTED_EDGE('',*,*,#57600,.F.);
#86046=ORIENTED_EDGE('',*,*,#57601,.T.);
#86047=ORIENTED_EDGE('',*,*,#57602,.T.);
#86048=ORIENTED_EDGE('',*,*,#57598,.F.);
#86049=ORIENTED_EDGE('',*,*,#57603,.F.);
#86050=ORIENTED_EDGE('',*,*,#57604,.T.);
#86051=ORIENTED_EDGE('',*,*,#57605,.T.);
#86052=ORIENTED_EDGE('',*,*,#57601,.F.);
#86053=ORIENTED_EDGE('',*,*,#57606,.F.);
#86054=ORIENTED_EDGE('',*,*,#57607,.F.);
#86055=ORIENTED_EDGE('',*,*,#57608,.F.);
#86056=ORIENTED_EDGE('',*,*,#57609,.F.);
#86057=ORIENTED_EDGE('',*,*,#57610,.T.);
#86058=ORIENTED_EDGE('',*,*,#57611,.T.);
#86059=ORIENTED_EDGE('',*,*,#57612,.T.);
#86060=ORIENTED_EDGE('',*,*,#57613,.T.);
#86061=ORIENTED_EDGE('',*,*,#57612,.F.);
#86062=ORIENTED_EDGE('',*,*,#57614,.T.);
#86063=ORIENTED_EDGE('',*,*,#57615,.T.);
#86064=ORIENTED_EDGE('',*,*,#57616,.T.);
#86065=ORIENTED_EDGE('',*,*,#57613,.F.);
#86066=ORIENTED_EDGE('',*,*,#57616,.F.);
#86067=ORIENTED_EDGE('',*,*,#57617,.F.);
#86068=ORIENTED_EDGE('',*,*,#57618,.T.);
#86069=ORIENTED_EDGE('',*,*,#57583,.T.);
#86070=ORIENTED_EDGE('',*,*,#57619,.T.);
#86071=ORIENTED_EDGE('',*,*,#57609,.T.);
#86072=ORIENTED_EDGE('',*,*,#57557,.T.);
#86073=ORIENTED_EDGE('',*,*,#57620,.T.);
#86074=ORIENTED_EDGE('',*,*,#57531,.T.);
#86075=ORIENTED_EDGE('',*,*,#57621,.T.);
#86076=ORIENTED_EDGE('',*,*,#57505,.T.);
#86077=ORIENTED_EDGE('',*,*,#57622,.T.);
#86078=ORIENTED_EDGE('',*,*,#57479,.T.);
#86079=ORIENTED_EDGE('',*,*,#57623,.T.);
#86080=ORIENTED_EDGE('',*,*,#57453,.T.);
#86081=ORIENTED_EDGE('',*,*,#57624,.T.);
#86082=ORIENTED_EDGE('',*,*,#57427,.T.);
#86083=ORIENTED_EDGE('',*,*,#57625,.T.);
#86084=ORIENTED_EDGE('',*,*,#57611,.F.);
#86085=ORIENTED_EDGE('',*,*,#57607,.T.);
#86086=ORIENTED_EDGE('',*,*,#57626,.T.);
#86087=ORIENTED_EDGE('',*,*,#57604,.F.);
#86088=ORIENTED_EDGE('',*,*,#57627,.F.);
#86089=ORIENTED_EDGE('',*,*,#57628,.F.);
#86090=ORIENTED_EDGE('',*,*,#57586,.F.);
#86091=ORIENTED_EDGE('',*,*,#57590,.F.);
#86092=ORIENTED_EDGE('',*,*,#57593,.F.);
#86093=ORIENTED_EDGE('',*,*,#57596,.F.);
#86094=ORIENTED_EDGE('',*,*,#57599,.F.);
#86095=ORIENTED_EDGE('',*,*,#57602,.F.);
#86096=ORIENTED_EDGE('',*,*,#57605,.F.);
#86097=ORIENTED_EDGE('',*,*,#57626,.F.);
#86098=ORIENTED_EDGE('',*,*,#57610,.F.);
#86099=ORIENTED_EDGE('',*,*,#57619,.F.);
#86100=ORIENTED_EDGE('',*,*,#57582,.F.);
#86101=ORIENTED_EDGE('',*,*,#57629,.F.);
#86102=ORIENTED_EDGE('',*,*,#57580,.F.);
#86103=ORIENTED_EDGE('',*,*,#57577,.F.);
#86104=ORIENTED_EDGE('',*,*,#57574,.F.);
#86105=ORIENTED_EDGE('',*,*,#57571,.F.);
#86106=ORIENTED_EDGE('',*,*,#57568,.F.);
#86107=ORIENTED_EDGE('',*,*,#57565,.F.);
#86108=ORIENTED_EDGE('',*,*,#57561,.F.);
#86109=ORIENTED_EDGE('',*,*,#57630,.F.);
#86110=ORIENTED_EDGE('',*,*,#57563,.F.);
#86111=ORIENTED_EDGE('',*,*,#57567,.F.);
#86112=ORIENTED_EDGE('',*,*,#57570,.F.);
#86113=ORIENTED_EDGE('',*,*,#57573,.F.);
#86114=ORIENTED_EDGE('',*,*,#57576,.F.);
#86115=ORIENTED_EDGE('',*,*,#57579,.F.);
#86116=ORIENTED_EDGE('',*,*,#57631,.F.);
#86117=ORIENTED_EDGE('',*,*,#57584,.F.);
#86118=ORIENTED_EDGE('',*,*,#57618,.F.);
#86119=ORIENTED_EDGE('',*,*,#57608,.T.);
#86120=ORIENTED_EDGE('',*,*,#57627,.T.);
#86121=ORIENTED_EDGE('',*,*,#57606,.T.);
#86122=ORIENTED_EDGE('',*,*,#57603,.T.);
#86123=ORIENTED_EDGE('',*,*,#57600,.T.);
#86124=ORIENTED_EDGE('',*,*,#57597,.T.);
#86125=ORIENTED_EDGE('',*,*,#57594,.T.);
#86126=ORIENTED_EDGE('',*,*,#57591,.T.);
#86127=ORIENTED_EDGE('',*,*,#57588,.T.);
#86128=ORIENTED_EDGE('',*,*,#57632,.T.);
#86129=ORIENTED_EDGE('',*,*,#57431,.T.);
#86130=ORIENTED_EDGE('',*,*,#57633,.T.);
#86131=ORIENTED_EDGE('',*,*,#57404,.T.);
#86132=ORIENTED_EDGE('',*,*,#57408,.T.);
#86133=ORIENTED_EDGE('',*,*,#57634,.T.);
#86134=ORIENTED_EDGE('',*,*,#57483,.T.);
#86135=ORIENTED_EDGE('',*,*,#57635,.T.);
#86136=ORIENTED_EDGE('',*,*,#57456,.T.);
#86137=ORIENTED_EDGE('',*,*,#57460,.T.);
#86138=ORIENTED_EDGE('',*,*,#57636,.T.);
#86139=ORIENTED_EDGE('',*,*,#57535,.T.);
#86140=ORIENTED_EDGE('',*,*,#57637,.T.);
#86141=ORIENTED_EDGE('',*,*,#57508,.T.);
#86142=ORIENTED_EDGE('',*,*,#57512,.T.);
#86143=ORIENTED_EDGE('',*,*,#57638,.T.);
#86144=ORIENTED_EDGE('',*,*,#57639,.F.);
#86145=ORIENTED_EDGE('',*,*,#57630,.T.);
#86146=ORIENTED_EDGE('',*,*,#57587,.T.);
#86147=ORIENTED_EDGE('',*,*,#57628,.T.);
#86148=ORIENTED_EDGE('',*,*,#57560,.T.);
#86149=ORIENTED_EDGE('',*,*,#57564,.T.);
#86150=ORIENTED_EDGE('',*,*,#57581,.T.);
#86151=ORIENTED_EDGE('',*,*,#57631,.T.);
#86152=ORIENTED_EDGE('',*,*,#57578,.F.);
#86153=ORIENTED_EDGE('',*,*,#57629,.T.);
#86154=ORIENTED_EDGE('',*,*,#57640,.F.);
#86155=ORIENTED_EDGE('',*,*,#57641,.T.);
#86156=ORIENTED_EDGE('',*,*,#57642,.F.);
#86157=ORIENTED_EDGE('',*,*,#57641,.F.);
#86158=ORIENTED_EDGE('',*,*,#57614,.F.);
#86159=ORIENTED_EDGE('',*,*,#57615,.F.);
#86160=ORIENTED_EDGE('',*,*,#57643,.T.);
#86161=ORIENTED_EDGE('',*,*,#57644,.F.);
#86162=ORIENTED_EDGE('',*,*,#57643,.F.);
#86163=ORIENTED_EDGE('',*,*,#57644,.T.);
#86164=ORIENTED_EDGE('',*,*,#57645,.T.);
#86165=ORIENTED_EDGE('',*,*,#57646,.T.);
#86166=ORIENTED_EDGE('',*,*,#57645,.F.);
#86167=ORIENTED_EDGE('',*,*,#57647,.F.);
#86168=ORIENTED_EDGE('',*,*,#57648,.T.);
#86169=ORIENTED_EDGE('',*,*,#57617,.T.);
#86170=ORIENTED_EDGE('',*,*,#57648,.F.);
#86171=ORIENTED_EDGE('',*,*,#57632,.F.);
#86172=ORIENTED_EDGE('',*,*,#57649,.T.);
#86173=ORIENTED_EDGE('',*,*,#57650,.T.);
#86174=ORIENTED_EDGE('',*,*,#57649,.F.);
#86175=ORIENTED_EDGE('',*,*,#57651,.F.);
#86176=ORIENTED_EDGE('',*,*,#57652,.T.);
#86177=ORIENTED_EDGE('',*,*,#57639,.T.);
#86178=ORIENTED_EDGE('',*,*,#57652,.F.);
#86179=ORIENTED_EDGE('',*,*,#57653,.F.);
#86180=ORIENTED_EDGE('',*,*,#57654,.T.);
#86181=ORIENTED_EDGE('',*,*,#57655,.T.);
#86182=ORIENTED_EDGE('',*,*,#57654,.F.);
#86183=ORIENTED_EDGE('',*,*,#57656,.F.);
#86184=ORIENTED_EDGE('',*,*,#57657,.T.);
#86185=ORIENTED_EDGE('',*,*,#57658,.T.);
#86186=ORIENTED_EDGE('',*,*,#57657,.F.);
#86187=ORIENTED_EDGE('',*,*,#57659,.F.);
#86188=ORIENTED_EDGE('',*,*,#57660,.T.);
#86189=ORIENTED_EDGE('',*,*,#57661,.T.);
#86190=ORIENTED_EDGE('',*,*,#57660,.F.);
#86191=ORIENTED_EDGE('',*,*,#57662,.F.);
#86192=ORIENTED_EDGE('',*,*,#57663,.T.);
#86193=ORIENTED_EDGE('',*,*,#57664,.T.);
#86194=ORIENTED_EDGE('',*,*,#57663,.F.);
#86195=ORIENTED_EDGE('',*,*,#57665,.F.);
#86196=ORIENTED_EDGE('',*,*,#57666,.T.);
#86197=ORIENTED_EDGE('',*,*,#57667,.T.);
#86198=ORIENTED_EDGE('',*,*,#57666,.F.);
#86199=ORIENTED_EDGE('',*,*,#57668,.F.);
#86200=ORIENTED_EDGE('',*,*,#57669,.T.);
#86201=ORIENTED_EDGE('',*,*,#57670,.T.);
#86202=ORIENTED_EDGE('',*,*,#57669,.F.);
#86203=ORIENTED_EDGE('',*,*,#57671,.F.);
#86204=ORIENTED_EDGE('',*,*,#57672,.T.);
#86205=ORIENTED_EDGE('',*,*,#57673,.T.);
#86206=ORIENTED_EDGE('',*,*,#57672,.F.);
#86207=ORIENTED_EDGE('',*,*,#57674,.F.);
#86208=ORIENTED_EDGE('',*,*,#57675,.T.);
#86209=ORIENTED_EDGE('',*,*,#57676,.T.);
#86210=ORIENTED_EDGE('',*,*,#57675,.F.);
#86211=ORIENTED_EDGE('',*,*,#57677,.F.);
#86212=ORIENTED_EDGE('',*,*,#57678,.T.);
#86213=ORIENTED_EDGE('',*,*,#57679,.T.);
#86214=ORIENTED_EDGE('',*,*,#57678,.F.);
#86215=ORIENTED_EDGE('',*,*,#57680,.F.);
#86216=ORIENTED_EDGE('',*,*,#57681,.T.);
#86217=ORIENTED_EDGE('',*,*,#57682,.T.);
#86218=ORIENTED_EDGE('',*,*,#57681,.F.);
#86219=ORIENTED_EDGE('',*,*,#57683,.F.);
#86220=ORIENTED_EDGE('',*,*,#57684,.T.);
#86221=ORIENTED_EDGE('',*,*,#57685,.T.);
#86222=ORIENTED_EDGE('',*,*,#57684,.F.);
#86223=ORIENTED_EDGE('',*,*,#57686,.F.);
#86224=ORIENTED_EDGE('',*,*,#57687,.T.);
#86225=ORIENTED_EDGE('',*,*,#57688,.T.);
#86226=ORIENTED_EDGE('',*,*,#57687,.F.);
#86227=ORIENTED_EDGE('',*,*,#57689,.F.);
#86228=ORIENTED_EDGE('',*,*,#57690,.T.);
#86229=ORIENTED_EDGE('',*,*,#57691,.T.);
#86230=ORIENTED_EDGE('',*,*,#57690,.F.);
#86231=ORIENTED_EDGE('',*,*,#57692,.F.);
#86232=ORIENTED_EDGE('',*,*,#57693,.T.);
#86233=ORIENTED_EDGE('',*,*,#57694,.T.);
#86234=ORIENTED_EDGE('',*,*,#57693,.F.);
#86235=ORIENTED_EDGE('',*,*,#57695,.F.);
#86236=ORIENTED_EDGE('',*,*,#57696,.T.);
#86237=ORIENTED_EDGE('',*,*,#57697,.T.);
#86238=ORIENTED_EDGE('',*,*,#57696,.F.);
#86239=ORIENTED_EDGE('',*,*,#57698,.F.);
#86240=ORIENTED_EDGE('',*,*,#57699,.T.);
#86241=ORIENTED_EDGE('',*,*,#57700,.T.);
#86242=ORIENTED_EDGE('',*,*,#57699,.F.);
#86243=ORIENTED_EDGE('',*,*,#57701,.F.);
#86244=ORIENTED_EDGE('',*,*,#57702,.T.);
#86245=ORIENTED_EDGE('',*,*,#57703,.T.);
#86246=ORIENTED_EDGE('',*,*,#57702,.F.);
#86247=ORIENTED_EDGE('',*,*,#57701,.T.);
#86248=ORIENTED_EDGE('',*,*,#57646,.F.);
#86249=ORIENTED_EDGE('',*,*,#57703,.F.);
#86250=ORIENTED_EDGE('',*,*,#57698,.T.);
#86251=ORIENTED_EDGE('',*,*,#57695,.T.);
#86252=ORIENTED_EDGE('',*,*,#57700,.F.);
#86253=ORIENTED_EDGE('',*,*,#57697,.F.);
#86254=ORIENTED_EDGE('',*,*,#57692,.T.);
#86255=ORIENTED_EDGE('',*,*,#57689,.T.);
#86256=ORIENTED_EDGE('',*,*,#57694,.F.);
#86257=ORIENTED_EDGE('',*,*,#57691,.F.);
#86258=ORIENTED_EDGE('',*,*,#57686,.T.);
#86259=ORIENTED_EDGE('',*,*,#57683,.T.);
#86260=ORIENTED_EDGE('',*,*,#57688,.F.);
#86261=ORIENTED_EDGE('',*,*,#57685,.F.);
#86262=ORIENTED_EDGE('',*,*,#57680,.T.);
#86263=ORIENTED_EDGE('',*,*,#57677,.T.);
#86264=ORIENTED_EDGE('',*,*,#57682,.F.);
#86265=ORIENTED_EDGE('',*,*,#57679,.F.);
#86266=ORIENTED_EDGE('',*,*,#57674,.T.);
#86267=ORIENTED_EDGE('',*,*,#57671,.T.);
#86268=ORIENTED_EDGE('',*,*,#57676,.F.);
#86269=ORIENTED_EDGE('',*,*,#57673,.F.);
#86270=ORIENTED_EDGE('',*,*,#57668,.T.);
#86271=ORIENTED_EDGE('',*,*,#57665,.T.);
#86272=ORIENTED_EDGE('',*,*,#57670,.F.);
#86273=ORIENTED_EDGE('',*,*,#57667,.F.);
#86274=ORIENTED_EDGE('',*,*,#57662,.T.);
#86275=ORIENTED_EDGE('',*,*,#57659,.T.);
#86276=ORIENTED_EDGE('',*,*,#57664,.F.);
#86277=ORIENTED_EDGE('',*,*,#57661,.F.);
#86278=ORIENTED_EDGE('',*,*,#57656,.T.);
#86279=ORIENTED_EDGE('',*,*,#57653,.T.);
#86280=ORIENTED_EDGE('',*,*,#57658,.F.);
#86281=ORIENTED_EDGE('',*,*,#57655,.F.);
#86282=ORIENTED_EDGE('',*,*,#57651,.T.);
#86283=ORIENTED_EDGE('',*,*,#57650,.F.);
#86284=ORIENTED_EDGE('',*,*,#57640,.T.);
#86285=ORIENTED_EDGE('',*,*,#57647,.T.);
#86286=ORIENTED_EDGE('',*,*,#57642,.T.);
#86287=ORIENTED_EDGE('',*,*,#57555,.T.);
#86288=ORIENTED_EDGE('',*,*,#57704,.T.);
#86289=ORIENTED_EDGE('',*,*,#57552,.F.);
#86290=ORIENTED_EDGE('',*,*,#57705,.F.);
#86291=ORIENTED_EDGE('',*,*,#57637,.F.);
#86292=ORIENTED_EDGE('',*,*,#57534,.F.);
#86293=ORIENTED_EDGE('',*,*,#57538,.F.);
#86294=ORIENTED_EDGE('',*,*,#57541,.F.);
#86295=ORIENTED_EDGE('',*,*,#57544,.F.);
#86296=ORIENTED_EDGE('',*,*,#57547,.F.);
#86297=ORIENTED_EDGE('',*,*,#57550,.F.);
#86298=ORIENTED_EDGE('',*,*,#57553,.F.);
#86299=ORIENTED_EDGE('',*,*,#57704,.F.);
#86300=ORIENTED_EDGE('',*,*,#57558,.F.);
#86301=ORIENTED_EDGE('',*,*,#57621,.F.);
#86302=ORIENTED_EDGE('',*,*,#57530,.F.);
#86303=ORIENTED_EDGE('',*,*,#57706,.F.);
#86304=ORIENTED_EDGE('',*,*,#57528,.F.);
#86305=ORIENTED_EDGE('',*,*,#57525,.F.);
#86306=ORIENTED_EDGE('',*,*,#57522,.F.);
#86307=ORIENTED_EDGE('',*,*,#57519,.F.);
#86308=ORIENTED_EDGE('',*,*,#57516,.F.);
#86309=ORIENTED_EDGE('',*,*,#57513,.F.);
#86310=ORIENTED_EDGE('',*,*,#57509,.F.);
#86311=ORIENTED_EDGE('',*,*,#57638,.F.);
#86312=ORIENTED_EDGE('',*,*,#57511,.F.);
#86313=ORIENTED_EDGE('',*,*,#57515,.F.);
#86314=ORIENTED_EDGE('',*,*,#57518,.F.);
#86315=ORIENTED_EDGE('',*,*,#57521,.F.);
#86316=ORIENTED_EDGE('',*,*,#57524,.F.);
#86317=ORIENTED_EDGE('',*,*,#57527,.F.);
#86318=ORIENTED_EDGE('',*,*,#57707,.F.);
#86319=ORIENTED_EDGE('',*,*,#57532,.F.);
#86320=ORIENTED_EDGE('',*,*,#57620,.F.);
#86321=ORIENTED_EDGE('',*,*,#57556,.T.);
#86322=ORIENTED_EDGE('',*,*,#57705,.T.);
#86323=ORIENTED_EDGE('',*,*,#57554,.T.);
#86324=ORIENTED_EDGE('',*,*,#57551,.T.);
#86325=ORIENTED_EDGE('',*,*,#57548,.T.);
#86326=ORIENTED_EDGE('',*,*,#57545,.T.);
#86327=ORIENTED_EDGE('',*,*,#57542,.T.);
#86328=ORIENTED_EDGE('',*,*,#57539,.T.);
#86329=ORIENTED_EDGE('',*,*,#57536,.T.);
#86330=ORIENTED_EDGE('',*,*,#57529,.T.);
#86331=ORIENTED_EDGE('',*,*,#57707,.T.);
#86332=ORIENTED_EDGE('',*,*,#57526,.F.);
#86333=ORIENTED_EDGE('',*,*,#57706,.T.);
#86334=ORIENTED_EDGE('',*,*,#57503,.T.);
#86335=ORIENTED_EDGE('',*,*,#57708,.T.);
#86336=ORIENTED_EDGE('',*,*,#57500,.F.);
#86337=ORIENTED_EDGE('',*,*,#57709,.F.);
#86338=ORIENTED_EDGE('',*,*,#57635,.F.);
#86339=ORIENTED_EDGE('',*,*,#57482,.F.);
#86340=ORIENTED_EDGE('',*,*,#57486,.F.);
#86341=ORIENTED_EDGE('',*,*,#57489,.F.);
#86342=ORIENTED_EDGE('',*,*,#57492,.F.);
#86343=ORIENTED_EDGE('',*,*,#57495,.F.);
#86344=ORIENTED_EDGE('',*,*,#57498,.F.);
#86345=ORIENTED_EDGE('',*,*,#57501,.F.);
#86346=ORIENTED_EDGE('',*,*,#57708,.F.);
#86347=ORIENTED_EDGE('',*,*,#57506,.F.);
#86348=ORIENTED_EDGE('',*,*,#57623,.F.);
#86349=ORIENTED_EDGE('',*,*,#57478,.F.);
#86350=ORIENTED_EDGE('',*,*,#57710,.F.);
#86351=ORIENTED_EDGE('',*,*,#57476,.F.);
#86352=ORIENTED_EDGE('',*,*,#57473,.F.);
#86353=ORIENTED_EDGE('',*,*,#57470,.F.);
#86354=ORIENTED_EDGE('',*,*,#57467,.F.);
#86355=ORIENTED_EDGE('',*,*,#57464,.F.);
#86356=ORIENTED_EDGE('',*,*,#57461,.F.);
#86357=ORIENTED_EDGE('',*,*,#57457,.F.);
#86358=ORIENTED_EDGE('',*,*,#57636,.F.);
#86359=ORIENTED_EDGE('',*,*,#57459,.F.);
#86360=ORIENTED_EDGE('',*,*,#57463,.F.);
#86361=ORIENTED_EDGE('',*,*,#57466,.F.);
#86362=ORIENTED_EDGE('',*,*,#57469,.F.);
#86363=ORIENTED_EDGE('',*,*,#57472,.F.);
#86364=ORIENTED_EDGE('',*,*,#57475,.F.);
#86365=ORIENTED_EDGE('',*,*,#57711,.F.);
#86366=ORIENTED_EDGE('',*,*,#57480,.F.);
#86367=ORIENTED_EDGE('',*,*,#57622,.F.);
#86368=ORIENTED_EDGE('',*,*,#57504,.T.);
#86369=ORIENTED_EDGE('',*,*,#57709,.T.);
#86370=ORIENTED_EDGE('',*,*,#57502,.T.);
#86371=ORIENTED_EDGE('',*,*,#57499,.T.);
#86372=ORIENTED_EDGE('',*,*,#57496,.T.);
#86373=ORIENTED_EDGE('',*,*,#57493,.T.);
#86374=ORIENTED_EDGE('',*,*,#57490,.T.);
#86375=ORIENTED_EDGE('',*,*,#57487,.T.);
#86376=ORIENTED_EDGE('',*,*,#57484,.T.);
#86377=ORIENTED_EDGE('',*,*,#57477,.T.);
#86378=ORIENTED_EDGE('',*,*,#57711,.T.);
#86379=ORIENTED_EDGE('',*,*,#57474,.F.);
#86380=ORIENTED_EDGE('',*,*,#57710,.T.);
#86381=ORIENTED_EDGE('',*,*,#57451,.T.);
#86382=ORIENTED_EDGE('',*,*,#57712,.T.);
#86383=ORIENTED_EDGE('',*,*,#57448,.F.);
#86384=ORIENTED_EDGE('',*,*,#57713,.F.);
#86385=ORIENTED_EDGE('',*,*,#57633,.F.);
#86386=ORIENTED_EDGE('',*,*,#57430,.F.);
#86387=ORIENTED_EDGE('',*,*,#57434,.F.);
#86388=ORIENTED_EDGE('',*,*,#57437,.F.);
#86389=ORIENTED_EDGE('',*,*,#57440,.F.);
#86390=ORIENTED_EDGE('',*,*,#57443,.F.);
#86391=ORIENTED_EDGE('',*,*,#57446,.F.);
#86392=ORIENTED_EDGE('',*,*,#57449,.F.);
#86393=ORIENTED_EDGE('',*,*,#57712,.F.);
#86394=ORIENTED_EDGE('',*,*,#57454,.F.);
#86395=ORIENTED_EDGE('',*,*,#57625,.F.);
#86396=ORIENTED_EDGE('',*,*,#57426,.F.);
#86397=ORIENTED_EDGE('',*,*,#57714,.F.);
#86398=ORIENTED_EDGE('',*,*,#57424,.F.);
#86399=ORIENTED_EDGE('',*,*,#57421,.F.);
#86400=ORIENTED_EDGE('',*,*,#57418,.F.);
#86401=ORIENTED_EDGE('',*,*,#57415,.F.);
#86402=ORIENTED_EDGE('',*,*,#57412,.F.);
#86403=ORIENTED_EDGE('',*,*,#57409,.F.);
#86404=ORIENTED_EDGE('',*,*,#57405,.F.);
#86405=ORIENTED_EDGE('',*,*,#57634,.F.);
#86406=ORIENTED_EDGE('',*,*,#57407,.F.);
#86407=ORIENTED_EDGE('',*,*,#57411,.F.);
#86408=ORIENTED_EDGE('',*,*,#57414,.F.);
#86409=ORIENTED_EDGE('',*,*,#57417,.F.);
#86410=ORIENTED_EDGE('',*,*,#57420,.F.);
#86411=ORIENTED_EDGE('',*,*,#57423,.F.);
#86412=ORIENTED_EDGE('',*,*,#57715,.F.);
#86413=ORIENTED_EDGE('',*,*,#57428,.F.);
#86414=ORIENTED_EDGE('',*,*,#57624,.F.);
#86415=ORIENTED_EDGE('',*,*,#57452,.T.);
#86416=ORIENTED_EDGE('',*,*,#57713,.T.);
#86417=ORIENTED_EDGE('',*,*,#57450,.T.);
#86418=ORIENTED_EDGE('',*,*,#57447,.T.);
#86419=ORIENTED_EDGE('',*,*,#57444,.T.);
#86420=ORIENTED_EDGE('',*,*,#57441,.T.);
#86421=ORIENTED_EDGE('',*,*,#57438,.T.);
#86422=ORIENTED_EDGE('',*,*,#57435,.T.);
#86423=ORIENTED_EDGE('',*,*,#57432,.T.);
#86424=ORIENTED_EDGE('',*,*,#57425,.T.);
#86425=ORIENTED_EDGE('',*,*,#57715,.T.);
#86426=ORIENTED_EDGE('',*,*,#57422,.F.);
#86427=ORIENTED_EDGE('',*,*,#57714,.T.);
#88656=CYLINDRICAL_SURFACE('',#105176,1.03775);
#88657=CYLINDRICAL_SURFACE('',#105178,1.03775);
#88658=CYLINDRICAL_SURFACE('',#105180,1.03775);
#88659=CYLINDRICAL_SURFACE('',#105181,1.03775);
#88660=CYLINDRICAL_SURFACE('',#105182,1.03775);
#88661=CYLINDRICAL_SURFACE('',#105183,1.03775);
#88662=CYLINDRICAL_SURFACE('',#105184,1.03775);
#88663=CYLINDRICAL_SURFACE('',#105185,1.03775);
#88664=CYLINDRICAL_SURFACE('',#105187,1.29);
#88665=CYLINDRICAL_SURFACE('',#105189,1.29);
#88666=CYLINDRICAL_SURFACE('',#105190,1.29);
#88667=CYLINDRICAL_SURFACE('',#105191,1.29);
#88668=CYLINDRICAL_SURFACE('',#105192,1.29);
#88669=CYLINDRICAL_SURFACE('',#105193,1.29);
#88670=CYLINDRICAL_SURFACE('',#105194,1.29);
#88671=CYLINDRICAL_SURFACE('',#105195,1.29);
#88672=CYLINDRICAL_SURFACE('',#105197,1.03775);
#88673=CYLINDRICAL_SURFACE('',#105199,1.03775);
#88674=CYLINDRICAL_SURFACE('',#105201,1.03775);
#88675=CYLINDRICAL_SURFACE('',#105202,1.03775);
#88676=CYLINDRICAL_SURFACE('',#105203,1.03775);
#88677=CYLINDRICAL_SURFACE('',#105204,1.03775);
#88678=CYLINDRICAL_SURFACE('',#105205,1.03775);
#88679=CYLINDRICAL_SURFACE('',#105206,1.03775);
#88680=CYLINDRICAL_SURFACE('',#105208,1.29);
#88681=CYLINDRICAL_SURFACE('',#105210,1.29);
#88682=CYLINDRICAL_SURFACE('',#105211,1.29);
#88683=CYLINDRICAL_SURFACE('',#105212,1.29);
#88684=CYLINDRICAL_SURFACE('',#105213,1.29);
#88685=CYLINDRICAL_SURFACE('',#105214,1.29);
#88686=CYLINDRICAL_SURFACE('',#105215,1.29);
#88687=CYLINDRICAL_SURFACE('',#105216,1.29);
#88688=CYLINDRICAL_SURFACE('',#105218,1.03775);
#88689=CYLINDRICAL_SURFACE('',#105220,1.03775);
#88690=CYLINDRICAL_SURFACE('',#105222,1.03775);
#88691=CYLINDRICAL_SURFACE('',#105223,1.03775);
#88692=CYLINDRICAL_SURFACE('',#105224,1.03775);
#88693=CYLINDRICAL_SURFACE('',#105225,1.03775);
#88694=CYLINDRICAL_SURFACE('',#105226,1.03775);
#88695=CYLINDRICAL_SURFACE('',#105227,1.03775);
#88696=CYLINDRICAL_SURFACE('',#105229,1.29);
#88697=CYLINDRICAL_SURFACE('',#105231,1.29);
#88698=CYLINDRICAL_SURFACE('',#105232,1.29);
#88699=CYLINDRICAL_SURFACE('',#105233,1.29);
#88700=CYLINDRICAL_SURFACE('',#105234,1.29);
#88701=CYLINDRICAL_SURFACE('',#105235,1.29);
#88702=CYLINDRICAL_SURFACE('',#105236,1.29);
#88703=CYLINDRICAL_SURFACE('',#105237,1.29);
#88704=CYLINDRICAL_SURFACE('',#105239,1.03775);
#88705=CYLINDRICAL_SURFACE('',#105241,1.03775);
#88706=CYLINDRICAL_SURFACE('',#105243,1.03775);
#88707=CYLINDRICAL_SURFACE('',#105244,1.03775);
#88708=CYLINDRICAL_SURFACE('',#105245,1.03775);
#88709=CYLINDRICAL_SURFACE('',#105246,1.03775);
#88710=CYLINDRICAL_SURFACE('',#105247,1.03775);
#88711=CYLINDRICAL_SURFACE('',#105248,1.03775);
#88712=CYLINDRICAL_SURFACE('',#105250,1.29);
#88713=CYLINDRICAL_SURFACE('',#105252,1.29);
#88714=CYLINDRICAL_SURFACE('',#105253,1.29);
#88715=CYLINDRICAL_SURFACE('',#105254,1.29);
#88716=CYLINDRICAL_SURFACE('',#105255,1.29);
#88717=CYLINDRICAL_SURFACE('',#105256,1.29);
#88718=CYLINDRICAL_SURFACE('',#105257,1.29);
#88719=CYLINDRICAL_SURFACE('',#105258,1.29);
#88720=CYLINDRICAL_SURFACE('',#105263,2.1);
#88721=CYLINDRICAL_SURFACE('',#105268,1.29);
#88722=CYLINDRICAL_SURFACE('',#105272,1.03775);
#88723=CYLINDRICAL_SURFACE('',#105273,9.8);
#88724=CYLINDRICAL_SURFACE('',#105278,3.5);
#88725=CYLINDRICAL_SURFACE('',#105280,10.5);
#88726=CYLINDRICAL_SURFACE('',#105282,10.5);
#88727=CYLINDRICAL_SURFACE('',#105284,4.95184441433916);
#88728=CYLINDRICAL_SURFACE('',#105286,10.5);
#88729=CYLINDRICAL_SURFACE('',#105289,5.08286386254677);
#88730=CYLINDRICAL_SURFACE('',#105292,10.5);
#88731=CYLINDRICAL_SURFACE('',#105295,5.21388331075437);
#88732=CYLINDRICAL_SURFACE('',#105298,10.5);
#88733=CYLINDRICAL_SURFACE('',#105301,5.34490275896198);
#88734=CYLINDRICAL_SURFACE('',#105304,10.5);
#88735=CYLINDRICAL_SURFACE('',#105307,5.47592220716958);
#88736=CYLINDRICAL_SURFACE('',#105310,10.5);
#88737=CYLINDRICAL_SURFACE('',#105313,5.60694165537719);
#88738=CYLINDRICAL_SURFACE('',#105316,10.5);
#88739=CYLINDRICAL_SURFACE('',#105319,5.73796110358479);
#88740=CYLINDRICAL_SURFACE('',#105322,10.5);
#88741=CYLINDRICAL_SURFACE('',#105325,5.8689805517924);
#88742=CYLINDRICAL_SURFACE('',#105328,10.5);
#88743=CYLINDRICAL_SURFACE('',#105331,6.);
#88744=CYLINDRICAL_SURFACE('',#105334,10.5);
#88745=CYLINDRICAL_SURFACE('',#105357,1.29);
#88746=CYLINDRICAL_SURFACE('',#105358,1.03775);
#88747=CYLINDRICAL_SURFACE('',#105359,1.29);
#88748=CYLINDRICAL_SURFACE('',#105360,1.03775);
#88749=CYLINDRICAL_SURFACE('',#105361,1.29);
#88750=CYLINDRICAL_SURFACE('',#105362,1.03775);
#94367=ADVANCED_FACE('',(#11903),#88656,.F.);
#94368=ADVANCED_FACE('',(#11904),#88657,.F.);
#94369=ADVANCED_FACE('',(#11905),#88658,.F.);
#94370=ADVANCED_FACE('',(#11906),#88659,.F.);
#94371=ADVANCED_FACE('',(#11907),#88660,.F.);
#94372=ADVANCED_FACE('',(#11908),#88661,.F.);
#94373=ADVANCED_FACE('',(#11909),#88662,.F.);
#94374=ADVANCED_FACE('',(#11910),#88663,.F.);
#94375=ADVANCED_FACE('',(#11911),#88664,.F.);
#94376=ADVANCED_FACE('',(#11912),#88665,.F.);
#94377=ADVANCED_FACE('',(#11913),#88666,.F.);
#94378=ADVANCED_FACE('',(#11914),#88667,.F.);
#94379=ADVANCED_FACE('',(#11915),#88668,.F.);
#94380=ADVANCED_FACE('',(#11916),#88669,.F.);
#94381=ADVANCED_FACE('',(#11917),#88670,.F.);
#94382=ADVANCED_FACE('',(#11918),#88671,.F.);
#94383=ADVANCED_FACE('',(#11919),#88672,.F.);
#94384=ADVANCED_FACE('',(#11920),#88673,.F.);
#94385=ADVANCED_FACE('',(#11921),#88674,.F.);
#94386=ADVANCED_FACE('',(#11922),#88675,.F.);
#94387=ADVANCED_FACE('',(#11923),#88676,.F.);
#94388=ADVANCED_FACE('',(#11924),#88677,.F.);
#94389=ADVANCED_FACE('',(#11925),#88678,.F.);
#94390=ADVANCED_FACE('',(#11926),#88679,.F.);
#94391=ADVANCED_FACE('',(#11927),#88680,.F.);
#94392=ADVANCED_FACE('',(#11928),#88681,.F.);
#94393=ADVANCED_FACE('',(#11929),#88682,.F.);
#94394=ADVANCED_FACE('',(#11930),#88683,.F.);
#94395=ADVANCED_FACE('',(#11931),#88684,.F.);
#94396=ADVANCED_FACE('',(#11932),#88685,.F.);
#94397=ADVANCED_FACE('',(#11933),#88686,.F.);
#94398=ADVANCED_FACE('',(#11934),#88687,.F.);
#94399=ADVANCED_FACE('',(#11935),#88688,.F.);
#94400=ADVANCED_FACE('',(#11936),#88689,.F.);
#94401=ADVANCED_FACE('',(#11937),#88690,.F.);
#94402=ADVANCED_FACE('',(#11938),#88691,.F.);
#94403=ADVANCED_FACE('',(#11939),#88692,.F.);
#94404=ADVANCED_FACE('',(#11940),#88693,.F.);
#94405=ADVANCED_FACE('',(#11941),#88694,.F.);
#94406=ADVANCED_FACE('',(#11942),#88695,.F.);
#94407=ADVANCED_FACE('',(#11943),#88696,.F.);
#94408=ADVANCED_FACE('',(#11944),#88697,.F.);
#94409=ADVANCED_FACE('',(#11945),#88698,.F.);
#94410=ADVANCED_FACE('',(#11946),#88699,.F.);
#94411=ADVANCED_FACE('',(#11947),#88700,.F.);
#94412=ADVANCED_FACE('',(#11948),#88701,.F.);
#94413=ADVANCED_FACE('',(#11949),#88702,.F.);
#94414=ADVANCED_FACE('',(#11950),#88703,.F.);
#94415=ADVANCED_FACE('',(#11951),#88704,.F.);
#94416=ADVANCED_FACE('',(#11952),#88705,.F.);
#94417=ADVANCED_FACE('',(#11953),#88706,.F.);
#94418=ADVANCED_FACE('',(#11954),#88707,.F.);
#94419=ADVANCED_FACE('',(#11955),#88708,.F.);
#94420=ADVANCED_FACE('',(#11956),#88709,.F.);
#94421=ADVANCED_FACE('',(#11957),#88710,.F.);
#94422=ADVANCED_FACE('',(#11958),#88711,.F.);
#94423=ADVANCED_FACE('',(#11959),#88712,.F.);
#94424=ADVANCED_FACE('',(#11960),#88713,.F.);
#94425=ADVANCED_FACE('',(#11961),#88714,.F.);
#94426=ADVANCED_FACE('',(#11962),#88715,.F.);
#94427=ADVANCED_FACE('',(#11963),#88716,.F.);
#94428=ADVANCED_FACE('',(#11964),#88717,.F.);
#94429=ADVANCED_FACE('',(#11965),#88718,.F.);
#94430=ADVANCED_FACE('',(#11966),#88719,.F.);
#94431=ADVANCED_FACE('',(#11967),#5105,.F.);
#94432=ADVANCED_FACE('',(#11968),#88720,.F.);
#94433=ADVANCED_FACE('',(#11969,#5230,#5231,#5232,#5233,#5234),#6106,.T.);
#94434=ADVANCED_FACE('',(#11970),#88721,.F.);
#94435=ADVANCED_FACE('',(#11971),#6337,.F.);
#94436=ADVANCED_FACE('',(#11972),#6338,.F.);
#94437=ADVANCED_FACE('',(#11973,#5235,#5236,#5237,#5238,#5239),#6107,.T.);
#94438=ADVANCED_FACE('',(#11974),#88722,.F.);
#94439=ADVANCED_FACE('',(#11975),#88723,.T.);
#94440=ADVANCED_FACE('',(#11976),#5106,.F.);
#94441=ADVANCED_FACE('',(#11977),#88724,.F.);
#94442=ADVANCED_FACE('',(#11978),#88725,.T.);
#94443=ADVANCED_FACE('',(#11979),#88726,.T.);
#94444=ADVANCED_FACE('',(#11980),#88727,.T.);
#94445=ADVANCED_FACE('',(#11981),#88728,.T.);
#94446=ADVANCED_FACE('',(#11982),#88729,.T.);
#94447=ADVANCED_FACE('',(#11983),#88730,.T.);
#94448=ADVANCED_FACE('',(#11984),#88731,.T.);
#94449=ADVANCED_FACE('',(#11985),#88732,.T.);
#94450=ADVANCED_FACE('',(#11986),#88733,.T.);
#94451=ADVANCED_FACE('',(#11987),#88734,.T.);
#94452=ADVANCED_FACE('',(#11988),#88735,.T.);
#94453=ADVANCED_FACE('',(#11989),#88736,.T.);
#94454=ADVANCED_FACE('',(#11990),#88737,.T.);
#94455=ADVANCED_FACE('',(#11991),#88738,.T.);
#94456=ADVANCED_FACE('',(#11992),#88739,.T.);
#94457=ADVANCED_FACE('',(#11993),#88740,.T.);
#94458=ADVANCED_FACE('',(#11994),#88741,.T.);
#94459=ADVANCED_FACE('',(#11995),#88742,.T.);
#94460=ADVANCED_FACE('',(#11996),#88743,.T.);
#94461=ADVANCED_FACE('',(#11997),#88744,.T.);
#94462=ADVANCED_FACE('',(#11998,#5240),#6108,.T.);
#94463=ADVANCED_FACE('',(#11999,#5241),#6109,.T.);
#94464=ADVANCED_FACE('',(#12000,#5242),#6110,.T.);
#94465=ADVANCED_FACE('',(#12001,#5243),#6111,.T.);
#94466=ADVANCED_FACE('',(#12002,#5244),#6112,.T.);
#94467=ADVANCED_FACE('',(#12003,#5245),#6113,.T.);
#94468=ADVANCED_FACE('',(#12004,#5246),#6114,.T.);
#94469=ADVANCED_FACE('',(#12005,#5247),#6115,.T.);
#94470=ADVANCED_FACE('',(#12006,#5248),#6116,.T.);
#94471=ADVANCED_FACE('',(#12007,#5249),#6117,.T.);
#94472=ADVANCED_FACE('',(#12008,#5250),#6118,.T.);
#94473=ADVANCED_FACE('',(#12009,#5251),#6119,.T.);
#94474=ADVANCED_FACE('',(#12010,#5252),#6120,.T.);
#94475=ADVANCED_FACE('',(#12011,#5253),#6121,.T.);
#94476=ADVANCED_FACE('',(#12012,#5254),#6122,.T.);
#94477=ADVANCED_FACE('',(#12013,#5255),#6123,.T.);
#94478=ADVANCED_FACE('',(#12014,#5256),#6124,.T.);
#94479=ADVANCED_FACE('',(#12015,#5257),#6125,.T.);
#94480=ADVANCED_FACE('',(#12016,#5258),#6126,.T.);
#94481=ADVANCED_FACE('',(#12017,#5259),#6127,.T.);
#94482=ADVANCED_FACE('',(#12018),#88745,.F.);
#94483=ADVANCED_FACE('',(#12019),#6339,.F.);
#94484=ADVANCED_FACE('',(#12020),#6340,.F.);
#94485=ADVANCED_FACE('',(#12021),#88746,.F.);
#94486=ADVANCED_FACE('',(#12022),#88747,.F.);
#94487=ADVANCED_FACE('',(#12023),#6341,.F.);
#94488=ADVANCED_FACE('',(#12024),#6342,.F.);
#94489=ADVANCED_FACE('',(#12025),#88748,.F.);
#94490=ADVANCED_FACE('',(#12026),#88749,.F.);
#94491=ADVANCED_FACE('',(#12027),#6343,.F.);
#94492=ADVANCED_FACE('',(#12028),#6344,.F.);
#94493=ADVANCED_FACE('',(#12029),#88750,.F.);
#94667=CLOSED_SHELL('',(#94367,#94368,#94369,#94370,#94371,#94372,#94373,
#94374,#94375,#94376,#94377,#94378,#94379,#94380,#94381,#94382,#94383,#94384,
#94385,#94386,#94387,#94388,#94389,#94390,#94391,#94392,#94393,#94394,#94395,
#94396,#94397,#94398,#94399,#94400,#94401,#94402,#94403,#94404,#94405,#94406,
#94407,#94408,#94409,#94410,#94411,#94412,#94413,#94414,#94415,#94416,#94417,
#94418,#94419,#94420,#94421,#94422,#94423,#94424,#94425,#94426,#94427,#94428,
#94429,#94430,#94431,#94432,#94433,#94434,#94435,#94436,#94437,#94438,#94439,
#94440,#94441,#94442,#94443,#94444,#94445,#94446,#94447,#94448,#94449,#94450,
#94451,#94452,#94453,#94454,#94455,#94456,#94457,#94458,#94459,#94460,#94461,
#94462,#94463,#94464,#94465,#94466,#94467,#94468,#94469,#94470,#94471,#94472,
#94473,#94474,#94475,#94476,#94477,#94478,#94479,#94480,#94481,#94482,#94483,
#94484,#94485,#94486,#94487,#94488,#94489,#94490,#94491,#94492,#94493));
#105175=AXIS2_PLACEMENT_3D('',#449392,#129685,#129686);
#105176=AXIS2_PLACEMENT_3D('',#449393,#129687,#129688);
#105177=AXIS2_PLACEMENT_3D('',#449398,#129690,#129691);
#105178=AXIS2_PLACEMENT_3D('',#449406,#129692,#129693);
#105179=AXIS2_PLACEMENT_3D('',#449430,#129695,#129696);
#105180=AXIS2_PLACEMENT_3D('',#449453,#129697,#129698);
#105181=AXIS2_PLACEMENT_3D('',#449501,#129700,#129701);
#105182=AXIS2_PLACEMENT_3D('',#449552,#129703,#129704);
#105183=AXIS2_PLACEMENT_3D('',#449603,#129706,#129707);
#105184=AXIS2_PLACEMENT_3D('',#449651,#129709,#129710);
#105185=AXIS2_PLACEMENT_3D('',#449702,#129712,#129713);
#105186=AXIS2_PLACEMENT_3D('',#449721,#129715,#129716);
#105187=AXIS2_PLACEMENT_3D('',#449741,#129717,#129718);
#105188=AXIS2_PLACEMENT_3D('',#449754,#129720,#129721);
#105189=AXIS2_PLACEMENT_3D('',#449762,#129722,#129723);
#105190=AXIS2_PLACEMENT_3D('',#449786,#129725,#129726);
#105191=AXIS2_PLACEMENT_3D('',#449811,#129728,#129729);
#105192=AXIS2_PLACEMENT_3D('',#449835,#129731,#129732);
#105193=AXIS2_PLACEMENT_3D('',#449860,#129734,#129735);
#105194=AXIS2_PLACEMENT_3D('',#449885,#129737,#129738);
#105195=AXIS2_PLACEMENT_3D('',#449909,#129740,#129741);
#105196=AXIS2_PLACEMENT_3D('',#449920,#129743,#129744);
#105197=AXIS2_PLACEMENT_3D('',#449926,#129745,#129746);
#105198=AXIS2_PLACEMENT_3D('',#449931,#129748,#129749);
#105199=AXIS2_PLACEMENT_3D('',#449939,#129750,#129751);
#105200=AXIS2_PLACEMENT_3D('',#449963,#129753,#129754);
#105201=AXIS2_PLACEMENT_3D('',#449986,#129755,#129756);
#105202=AXIS2_PLACEMENT_3D('',#450034,#129758,#129759);
#105203=AXIS2_PLACEMENT_3D('',#450085,#129761,#129762);
#105204=AXIS2_PLACEMENT_3D('',#450136,#129764,#129765);
#105205=AXIS2_PLACEMENT_3D('',#450184,#129767,#129768);
#105206=AXIS2_PLACEMENT_3D('',#450235,#129770,#129771);
#105207=AXIS2_PLACEMENT_3D('',#450254,#129773,#129774);
#105208=AXIS2_PLACEMENT_3D('',#450274,#129775,#129776);
#105209=AXIS2_PLACEMENT_3D('',#450287,#129778,#129779);
#105210=AXIS2_PLACEMENT_3D('',#450295,#129780,#129781);
#105211=AXIS2_PLACEMENT_3D('',#450319,#129783,#129784);
#105212=AXIS2_PLACEMENT_3D('',#450344,#129786,#129787);
#105213=AXIS2_PLACEMENT_3D('',#450368,#129789,#129790);
#105214=AXIS2_PLACEMENT_3D('',#450393,#129792,#129793);
#105215=AXIS2_PLACEMENT_3D('',#450418,#129795,#129796);
#105216=AXIS2_PLACEMENT_3D('',#450442,#129798,#129799);
#105217=AXIS2_PLACEMENT_3D('',#450453,#129801,#129802);
#105218=AXIS2_PLACEMENT_3D('',#450459,#129803,#129804);
#105219=AXIS2_PLACEMENT_3D('',#450464,#129806,#129807);
#105220=AXIS2_PLACEMENT_3D('',#450472,#129808,#129809);
#105221=AXIS2_PLACEMENT_3D('',#450496,#129811,#129812);
#105222=AXIS2_PLACEMENT_3D('',#450519,#129813,#129814);
#105223=AXIS2_PLACEMENT_3D('',#450567,#129816,#129817);
#105224=AXIS2_PLACEMENT_3D('',#450618,#129819,#129820);
#105225=AXIS2_PLACEMENT_3D('',#450669,#129822,#129823);
#105226=AXIS2_PLACEMENT_3D('',#450717,#129825,#129826);
#105227=AXIS2_PLACEMENT_3D('',#450768,#129828,#129829);
#105228=AXIS2_PLACEMENT_3D('',#450787,#129831,#129832);
#105229=AXIS2_PLACEMENT_3D('',#450807,#129833,#129834);
#105230=AXIS2_PLACEMENT_3D('',#450820,#129836,#129837);
#105231=AXIS2_PLACEMENT_3D('',#450828,#129838,#129839);
#105232=AXIS2_PLACEMENT_3D('',#450852,#129841,#129842);
#105233=AXIS2_PLACEMENT_3D('',#450877,#129844,#129845);
#105234=AXIS2_PLACEMENT_3D('',#450901,#129847,#129848);
#105235=AXIS2_PLACEMENT_3D('',#450926,#129850,#129851);
#105236=AXIS2_PLACEMENT_3D('',#450951,#129853,#129854);
#105237=AXIS2_PLACEMENT_3D('',#450975,#129856,#129857);
#105238=AXIS2_PLACEMENT_3D('',#450986,#129859,#129860);
#105239=AXIS2_PLACEMENT_3D('',#450992,#129861,#129862);
#105240=AXIS2_PLACEMENT_3D('',#450997,#129864,#129865);
#105241=AXIS2_PLACEMENT_3D('',#451005,#129866,#129867);
#105242=AXIS2_PLACEMENT_3D('',#451029,#129869,#129870);
#105243=AXIS2_PLACEMENT_3D('',#451052,#129871,#129872);
#105244=AXIS2_PLACEMENT_3D('',#451100,#129874,#129875);
#105245=AXIS2_PLACEMENT_3D('',#451151,#129877,#129878);
#105246=AXIS2_PLACEMENT_3D('',#451202,#129880,#129881);
#105247=AXIS2_PLACEMENT_3D('',#451250,#129883,#129884);
#105248=AXIS2_PLACEMENT_3D('',#451301,#129886,#129887);
#105249=AXIS2_PLACEMENT_3D('',#451320,#129889,#129890);
#105250=AXIS2_PLACEMENT_3D('',#451340,#129891,#129892);
#105251=AXIS2_PLACEMENT_3D('',#451353,#129894,#129895);
#105252=AXIS2_PLACEMENT_3D('',#451361,#129896,#129897);
#105253=AXIS2_PLACEMENT_3D('',#451385,#129899,#129900);
#105254=AXIS2_PLACEMENT_3D('',#451410,#129902,#129903);
#105255=AXIS2_PLACEMENT_3D('',#451434,#129905,#129906);
#105256=AXIS2_PLACEMENT_3D('',#451459,#129908,#129909);
#105257=AXIS2_PLACEMENT_3D('',#451484,#129911,#129912);
#105258=AXIS2_PLACEMENT_3D('',#451508,#129914,#129915);
#105259=AXIS2_PLACEMENT_3D('',#451519,#129917,#129918);
#105260=AXIS2_PLACEMENT_3D('',#451525,#129919,#129920);
#105261=AXIS2_PLACEMENT_3D('',#451527,#129921,#129922);
#105262=AXIS2_PLACEMENT_3D('',#451530,#129924,#129925);
#105263=AXIS2_PLACEMENT_3D('',#451531,#129926,#129927);
#105264=AXIS2_PLACEMENT_3D('',#451534,#129928,#129929);
#105265=AXIS2_PLACEMENT_3D('',#451535,#129930,#129931);
#105266=AXIS2_PLACEMENT_3D('',#451537,#129933,#129934);
#105267=AXIS2_PLACEMENT_3D('',#451539,#129935,#129936);
#105268=AXIS2_PLACEMENT_3D('',#452172,#129937,#129938);
#105269=AXIS2_PLACEMENT_3D('',#452831,#129939,#129940);
#105270=AXIS2_PLACEMENT_3D('',#452833,#129941,#129942);
#105271=AXIS2_PLACEMENT_3D('',#453309,#129943,#129944);
#105272=AXIS2_PLACEMENT_3D('',#453310,#129945,#129946);
#105273=AXIS2_PLACEMENT_3D('',#453311,#129947,#129948);
#105274=AXIS2_PLACEMENT_3D('',#453313,#129949,#129950);
#105275=AXIS2_PLACEMENT_3D('',#453316,#129952,#129953);
#105276=AXIS2_PLACEMENT_3D('',#453317,#129954,#129955);
#105277=AXIS2_PLACEMENT_3D('',#453320,#129957,#129958);
#105278=AXIS2_PLACEMENT_3D('',#453321,#129959,#129960);
#105279=AXIS2_PLACEMENT_3D('',#453324,#129962,#129963);
#105280=AXIS2_PLACEMENT_3D('',#453325,#129964,#129965);
#105281=AXIS2_PLACEMENT_3D('',#453327,#129966,#129967);
#105282=AXIS2_PLACEMENT_3D('',#453329,#129969,#129970);
#105283=AXIS2_PLACEMENT_3D('',#453332,#129972,#129973);
#105284=AXIS2_PLACEMENT_3D('',#453333,#129974,#129975);
#105285=AXIS2_PLACEMENT_3D('',#453335,#129976,#129977);
#105286=AXIS2_PLACEMENT_3D('',#453337,#129979,#129980);
#105287=AXIS2_PLACEMENT_3D('',#453339,#129981,#129982);
#105288=AXIS2_PLACEMENT_3D('',#453342,#129984,#129985);
#105289=AXIS2_PLACEMENT_3D('',#453343,#129986,#129987);
#105290=AXIS2_PLACEMENT_3D('',#453345,#129988,#129989);
#105291=AXIS2_PLACEMENT_3D('',#453348,#129991,#129992);
#105292=AXIS2_PLACEMENT_3D('',#453349,#129993,#129994);
#105293=AXIS2_PLACEMENT_3D('',#453351,#129995,#129996);
#105294=AXIS2_PLACEMENT_3D('',#453354,#129998,#129999);
#105295=AXIS2_PLACEMENT_3D('',#453355,#130000,#130001);
#105296=AXIS2_PLACEMENT_3D('',#453357,#130002,#130003);
#105297=AXIS2_PLACEMENT_3D('',#453360,#130005,#130006);
#105298=AXIS2_PLACEMENT_3D('',#453361,#130007,#130008);
#105299=AXIS2_PLACEMENT_3D('',#453363,#130009,#130010);
#105300=AXIS2_PLACEMENT_3D('',#453366,#130012,#130013);
#105301=AXIS2_PLACEMENT_3D('',#453367,#130014,#130015);
#105302=AXIS2_PLACEMENT_3D('',#453369,#130016,#130017);
#105303=AXIS2_PLACEMENT_3D('',#453372,#130019,#130020);
#105304=AXIS2_PLACEMENT_3D('',#453373,#130021,#130022);
#105305=AXIS2_PLACEMENT_3D('',#453375,#130023,#130024);
#105306=AXIS2_PLACEMENT_3D('',#453378,#130026,#130027);
#105307=AXIS2_PLACEMENT_3D('',#453379,#130028,#130029);
#105308=AXIS2_PLACEMENT_3D('',#453381,#130030,#130031);
#105309=AXIS2_PLACEMENT_3D('',#453384,#130033,#130034);
#105310=AXIS2_PLACEMENT_3D('',#453385,#130035,#130036);
#105311=AXIS2_PLACEMENT_3D('',#453387,#130037,#130038);
#105312=AXIS2_PLACEMENT_3D('',#453390,#130040,#130041);
#105313=AXIS2_PLACEMENT_3D('',#453391,#130042,#130043);
#105314=AXIS2_PLACEMENT_3D('',#453393,#130044,#130045);
#105315=AXIS2_PLACEMENT_3D('',#453396,#130047,#130048);
#105316=AXIS2_PLACEMENT_3D('',#453397,#130049,#130050);
#105317=AXIS2_PLACEMENT_3D('',#453399,#130051,#130052);
#105318=AXIS2_PLACEMENT_3D('',#453402,#130054,#130055);
#105319=AXIS2_PLACEMENT_3D('',#453403,#130056,#130057);
#105320=AXIS2_PLACEMENT_3D('',#453405,#130058,#130059);
#105321=AXIS2_PLACEMENT_3D('',#453408,#130061,#130062);
#105322=AXIS2_PLACEMENT_3D('',#453409,#130063,#130064);
#105323=AXIS2_PLACEMENT_3D('',#453411,#130065,#130066);
#105324=AXIS2_PLACEMENT_3D('',#453414,#130068,#130069);
#105325=AXIS2_PLACEMENT_3D('',#453415,#130070,#130071);
#105326=AXIS2_PLACEMENT_3D('',#453417,#130072,#130073);
#105327=AXIS2_PLACEMENT_3D('',#453420,#130075,#130076);
#105328=AXIS2_PLACEMENT_3D('',#453421,#130077,#130078);
#105329=AXIS2_PLACEMENT_3D('',#453423,#130079,#130080);
#105330=AXIS2_PLACEMENT_3D('',#453426,#130082,#130083);
#105331=AXIS2_PLACEMENT_3D('',#453427,#130084,#130085);
#105332=AXIS2_PLACEMENT_3D('',#453429,#130086,#130087);
#105333=AXIS2_PLACEMENT_3D('',#453432,#130089,#130090);
#105334=AXIS2_PLACEMENT_3D('',#453433,#130091,#130092);
#105335=AXIS2_PLACEMENT_3D('',#453435,#130093,#130094);
#105336=AXIS2_PLACEMENT_3D('',#453438,#130096,#130097);
#105337=AXIS2_PLACEMENT_3D('',#453439,#130098,#130099);
#105338=AXIS2_PLACEMENT_3D('',#453440,#130100,#130101);
#105339=AXIS2_PLACEMENT_3D('',#453441,#130102,#130103);
#105340=AXIS2_PLACEMENT_3D('',#453442,#130104,#130105);
#105341=AXIS2_PLACEMENT_3D('',#453443,#130106,#130107);
#105342=AXIS2_PLACEMENT_3D('',#453444,#130108,#130109);
#105343=AXIS2_PLACEMENT_3D('',#453445,#130110,#130111);
#105344=AXIS2_PLACEMENT_3D('',#453446,#130112,#130113);
#105345=AXIS2_PLACEMENT_3D('',#453447,#130114,#130115);
#105346=AXIS2_PLACEMENT_3D('',#453448,#130116,#130117);
#105347=AXIS2_PLACEMENT_3D('',#453449,#130118,#130119);
#105348=AXIS2_PLACEMENT_3D('',#453450,#130120,#130121);
#105349=AXIS2_PLACEMENT_3D('',#453451,#130122,#130123);
#105350=AXIS2_PLACEMENT_3D('',#453452,#130124,#130125);
#105351=AXIS2_PLACEMENT_3D('',#453453,#130126,#130127);
#105352=AXIS2_PLACEMENT_3D('',#453454,#130128,#130129);
#105353=AXIS2_PLACEMENT_3D('',#453455,#130130,#130131);
#105354=AXIS2_PLACEMENT_3D('',#453456,#130132,#130133);
#105355=AXIS2_PLACEMENT_3D('',#453457,#130134,#130135);
#105356=AXIS2_PLACEMENT_3D('',#453458,#130136,#130137);
#105357=AXIS2_PLACEMENT_3D('',#453459,#130138,#130139);
#105358=AXIS2_PLACEMENT_3D('',#453960,#130140,#130141);
#105359=AXIS2_PLACEMENT_3D('',#453961,#130142,#130143);
#105360=AXIS2_PLACEMENT_3D('',#454462,#130144,#130145);
#105361=AXIS2_PLACEMENT_3D('',#454463,#130146,#130147);
#105362=AXIS2_PLACEMENT_3D('',#454964,#130148,#130149);
#129685=DIRECTION('axis',(0.,0.,1.));
#129686=DIRECTION('refdir',(1.,0.,0.));
#129687=DIRECTION('center_axis',(0.,-1.,0.));
#129688=DIRECTION('ref_axis',(0.707106781186548,0.,0.707106781186547));
#129689=DIRECTION('',(0.,-1.,0.));
#129690=DIRECTION('center_axis',(0.,1.,0.));
#129691=DIRECTION('ref_axis',(0.707106781186548,0.,0.707106781186547));
#129692=DIRECTION('center_axis',(0.,-1.,0.));
#129693=DIRECTION('ref_axis',(0.707106781186548,0.,0.707106781186547));
#129694=DIRECTION('',(0.,-1.,0.));
#129695=DIRECTION('center_axis',(0.,1.,0.));
#129696=DIRECTION('ref_axis',(0.707106781186548,0.,0.707106781186547));
#129697=DIRECTION('center_axis',(0.,-1.,0.));
#129698=DIRECTION('ref_axis',(0.707106781186548,0.,0.707106781186547));
#129699=DIRECTION('',(0.,-1.,0.));
#129700=DIRECTION('center_axis',(0.,-1.,0.));
#129701=DIRECTION('ref_axis',(0.707106781186548,0.,0.707106781186547));
#129702=DIRECTION('',(0.,-1.,0.));
#129703=DIRECTION('center_axis',(0.,-1.,0.));
#129704=DIRECTION('ref_axis',(0.707106781186548,0.,0.707106781186547));
#129705=DIRECTION('',(0.,-1.,0.));
#129706=DIRECTION('center_axis',(0.,-1.,0.));
#129707=DIRECTION('ref_axis',(0.707106781186548,0.,0.707106781186547));
#129708=DIRECTION('',(0.,-1.,0.));
#129709=DIRECTION('center_axis',(0.,-1.,0.));
#129710=DIRECTION('ref_axis',(0.707106781186548,0.,0.707106781186547));
#129711=DIRECTION('',(0.,-1.,0.));
#129712=DIRECTION('center_axis',(0.,-1.,0.));
#129713=DIRECTION('ref_axis',(0.409955339817897,0.,0.912105596603152));
#129714=DIRECTION('',(0.,-1.,0.));
#129715=DIRECTION('center_axis',(0.,-1.,0.));
#129716=DIRECTION('ref_axis',(0.707106781186548,0.,0.707106781186547));
#129717=DIRECTION('center_axis',(0.,-1.,0.));
#129718=DIRECTION('ref_axis',(0.843556936084309,0.,-0.53703975233129));
#129719=DIRECTION('',(8.6595605623547E-17,-1.,8.65956056235516E-17));
#129720=DIRECTION('center_axis',(0.,1.,0.));
#129721=DIRECTION('ref_axis',(0.707106781186529,0.,0.707106781186566));
#129722=DIRECTION('center_axis',(0.,-1.,0.));
#129723=DIRECTION('ref_axis',(0.707106781186529,0.,0.707106781186566));
#129724=DIRECTION('',(8.6595605623547E-17,-1.,8.65956056235516E-17));
#129725=DIRECTION('center_axis',(0.,-1.,0.));
#129726=DIRECTION('ref_axis',(0.707106781186529,0.,0.707106781186566));
#129727=DIRECTION('',(8.6595605623547E-17,-1.,8.65956056235516E-17));
#129728=DIRECTION('center_axis',(0.,-1.,0.));
#129729=DIRECTION('ref_axis',(0.707106781186529,0.,0.707106781186566));
#129730=DIRECTION('',(8.6595605623547E-17,-1.,8.65956056235516E-17));
#129731=DIRECTION('center_axis',(0.,-1.,0.));
#129732=DIRECTION('ref_axis',(0.707106781186529,0.,0.707106781186566));
#129733=DIRECTION('',(8.6595605623547E-17,-1.,8.65956056235516E-17));
#129734=DIRECTION('center_axis',(0.,-1.,0.));
#129735=DIRECTION('ref_axis',(0.707106781186529,0.,0.707106781186566));
#129736=DIRECTION('',(8.6595605623547E-17,-1.,8.65956056235516E-17));
#129737=DIRECTION('center_axis',(0.,-1.,0.));
#129738=DIRECTION('ref_axis',(0.707106781186529,0.,0.707106781186566));
#129739=DIRECTION('',(8.6595605623547E-17,-1.,8.65956056235516E-17));
#129740=DIRECTION('center_axis',(0.,-1.,0.));
#129741=DIRECTION('ref_axis',(-0.991406989026756,0.,0.130813539470888));
#129742=DIRECTION('',(8.6595605623547E-17,-1.,8.65956056235516E-17));
#129743=DIRECTION('center_axis',(0.,-1.,0.));
#129744=DIRECTION('ref_axis',(0.707106781186529,0.,0.707106781186566));
#129745=DIRECTION('center_axis',(0.,-1.,0.));
#129746=DIRECTION('ref_axis',(0.707106781186547,0.,-0.707106781186548));
#129747=DIRECTION('',(0.,-1.,0.));
#129748=DIRECTION('center_axis',(0.,1.,0.));
#129749=DIRECTION('ref_axis',(0.707106781186547,0.,-0.707106781186548));
#129750=DIRECTION('center_axis',(0.,-1.,0.));
#129751=DIRECTION('ref_axis',(0.707106781186547,0.,-0.707106781186548));
#129752=DIRECTION('',(0.,-1.,0.));
#129753=DIRECTION('center_axis',(0.,1.,0.));
#129754=DIRECTION('ref_axis',(0.707106781186547,0.,-0.707106781186548));
#129755=DIRECTION('center_axis',(0.,-1.,0.));
#129756=DIRECTION('ref_axis',(0.707106781186547,0.,-0.707106781186548));
#129757=DIRECTION('',(0.,-1.,0.));
#129758=DIRECTION('center_axis',(0.,-1.,0.));
#129759=DIRECTION('ref_axis',(0.707106781186547,0.,-0.707106781186548));
#129760=DIRECTION('',(0.,-1.,0.));
#129761=DIRECTION('center_axis',(0.,-1.,0.));
#129762=DIRECTION('ref_axis',(0.707106781186547,0.,-0.707106781186548));
#129763=DIRECTION('',(0.,-1.,0.));
#129764=DIRECTION('center_axis',(0.,-1.,0.));
#129765=DIRECTION('ref_axis',(0.707106781186547,0.,-0.707106781186548));
#129766=DIRECTION('',(0.,-1.,0.));
#129767=DIRECTION('center_axis',(0.,-1.,0.));
#129768=DIRECTION('ref_axis',(0.707106781186547,0.,-0.707106781186548));
#129769=DIRECTION('',(0.,-1.,0.));
#129770=DIRECTION('center_axis',(0.,-1.,0.));
#129771=DIRECTION('ref_axis',(0.912105596603152,0.,-0.409955339817897));
#129772=DIRECTION('',(0.,-1.,0.));
#129773=DIRECTION('center_axis',(0.,-1.,0.));
#129774=DIRECTION('ref_axis',(0.707106781186547,0.,-0.707106781186548));
#129775=DIRECTION('center_axis',(0.,-1.,0.));
#129776=DIRECTION('ref_axis',(-0.53703975233129,0.,-0.843556936084309));
#129777=DIRECTION('',(8.65956056235516E-17,-1.,-8.6595605623547E-17));
#129778=DIRECTION('center_axis',(0.,1.,0.));
#129779=DIRECTION('ref_axis',(0.707106781186566,0.,-0.707106781186529));
#129780=DIRECTION('center_axis',(0.,-1.,0.));
#129781=DIRECTION('ref_axis',(0.707106781186566,0.,-0.707106781186529));
#129782=DIRECTION('',(8.65956056235516E-17,-1.,-8.6595605623547E-17));
#129783=DIRECTION('center_axis',(0.,-1.,0.));
#129784=DIRECTION('ref_axis',(0.707106781186566,0.,-0.707106781186529));
#129785=DIRECTION('',(8.65956056235516E-17,-1.,-8.6595605623547E-17));
#129786=DIRECTION('center_axis',(0.,-1.,0.));
#129787=DIRECTION('ref_axis',(0.707106781186566,0.,-0.707106781186529));
#129788=DIRECTION('',(8.65956056235516E-17,-1.,-8.6595605623547E-17));
#129789=DIRECTION('center_axis',(0.,-1.,0.));
#129790=DIRECTION('ref_axis',(0.707106781186566,0.,-0.707106781186529));
#129791=DIRECTION('',(8.65956056235516E-17,-1.,-8.6595605623547E-17));
#129792=DIRECTION('center_axis',(0.,-1.,0.));
#129793=DIRECTION('ref_axis',(0.707106781186566,0.,-0.707106781186529));
#129794=DIRECTION('',(8.65956056235516E-17,-1.,-8.6595605623547E-17));
#129795=DIRECTION('center_axis',(0.,-1.,0.));
#129796=DIRECTION('ref_axis',(0.707106781186566,0.,-0.707106781186529));
#129797=DIRECTION('',(8.65956056235516E-17,-1.,-8.6595605623547E-17));
#129798=DIRECTION('center_axis',(0.,-1.,0.));
#129799=DIRECTION('ref_axis',(0.130813539470888,0.,0.991406989026756));
#129800=DIRECTION('',(8.65956056235516E-17,-1.,-8.6595605623547E-17));
#129801=DIRECTION('center_axis',(0.,-1.,0.));
#129802=DIRECTION('ref_axis',(0.707106781186566,0.,-0.707106781186529));
#129803=DIRECTION('center_axis',(0.,-1.,0.));
#129804=DIRECTION('ref_axis',(-0.707106781186548,0.,-0.707106781186547));
#129805=DIRECTION('',(0.,-1.,0.));
#129806=DIRECTION('center_axis',(0.,1.,0.));
#129807=DIRECTION('ref_axis',(-0.707106781186548,0.,-0.707106781186547));
#129808=DIRECTION('center_axis',(0.,-1.,0.));
#129809=DIRECTION('ref_axis',(-0.707106781186548,0.,-0.707106781186547));
#129810=DIRECTION('',(0.,-1.,0.));
#129811=DIRECTION('center_axis',(0.,1.,0.));
#129812=DIRECTION('ref_axis',(-0.707106781186548,0.,-0.707106781186547));
#129813=DIRECTION('center_axis',(0.,-1.,0.));
#129814=DIRECTION('ref_axis',(-0.707106781186548,0.,-0.707106781186547));
#129815=DIRECTION('',(0.,-1.,0.));
#129816=DIRECTION('center_axis',(0.,-1.,0.));
#129817=DIRECTION('ref_axis',(-0.707106781186548,0.,-0.707106781186547));
#129818=DIRECTION('',(0.,-1.,0.));
#129819=DIRECTION('center_axis',(0.,-1.,0.));
#129820=DIRECTION('ref_axis',(-0.707106781186548,0.,-0.707106781186547));
#129821=DIRECTION('',(0.,-1.,0.));
#129822=DIRECTION('center_axis',(0.,-1.,0.));
#129823=DIRECTION('ref_axis',(-0.707106781186548,0.,-0.707106781186547));
#129824=DIRECTION('',(0.,-1.,0.));
#129825=DIRECTION('center_axis',(0.,-1.,0.));
#129826=DIRECTION('ref_axis',(-0.707106781186548,0.,-0.707106781186547));
#129827=DIRECTION('',(0.,-1.,0.));
#129828=DIRECTION('center_axis',(0.,-1.,0.));
#129829=DIRECTION('ref_axis',(-0.409955339817898,0.,-0.912105596603152));
#129830=DIRECTION('',(0.,-1.,0.));
#129831=DIRECTION('center_axis',(0.,-1.,0.));
#129832=DIRECTION('ref_axis',(-0.707106781186548,0.,-0.707106781186547));
#129833=DIRECTION('center_axis',(0.,-1.,0.));
#129834=DIRECTION('ref_axis',(-0.843556936084309,0.,0.53703975233129));
#129835=DIRECTION('',(-8.6595605623547E-17,-1.,-8.65956056235516E-17));
#129836=DIRECTION('center_axis',(0.,1.,0.));
#129837=DIRECTION('ref_axis',(-0.707106781186529,0.,-0.707106781186566));
#129838=DIRECTION('center_axis',(0.,-1.,0.));
#129839=DIRECTION('ref_axis',(-0.707106781186529,0.,-0.707106781186566));
#129840=DIRECTION('',(-8.6595605623547E-17,-1.,-8.65956056235516E-17));
#129841=DIRECTION('center_axis',(0.,-1.,0.));
#129842=DIRECTION('ref_axis',(-0.707106781186529,0.,-0.707106781186566));
#129843=DIRECTION('',(-8.6595605623547E-17,-1.,-8.65956056235516E-17));
#129844=DIRECTION('center_axis',(0.,-1.,0.));
#129845=DIRECTION('ref_axis',(-0.707106781186529,0.,-0.707106781186566));
#129846=DIRECTION('',(-8.6595605623547E-17,-1.,-8.65956056235516E-17));
#129847=DIRECTION('center_axis',(0.,-1.,0.));
#129848=DIRECTION('ref_axis',(-0.707106781186529,0.,-0.707106781186566));
#129849=DIRECTION('',(-8.6595605623547E-17,-1.,-8.65956056235516E-17));
#129850=DIRECTION('center_axis',(0.,-1.,0.));
#129851=DIRECTION('ref_axis',(-0.707106781186529,0.,-0.707106781186566));
#129852=DIRECTION('',(-8.6595605623547E-17,-1.,-8.65956056235516E-17));
#129853=DIRECTION('center_axis',(0.,-1.,0.));
#129854=DIRECTION('ref_axis',(-0.707106781186529,0.,-0.707106781186566));
#129855=DIRECTION('',(-8.6595605623547E-17,-1.,-8.65956056235516E-17));
#129856=DIRECTION('center_axis',(0.,-1.,0.));
#129857=DIRECTION('ref_axis',(0.991406989026756,0.,-0.130813539470888));
#129858=DIRECTION('',(-8.6595605623547E-17,-1.,-8.65956056235516E-17));
#129859=DIRECTION('center_axis',(0.,-1.,0.));
#129860=DIRECTION('ref_axis',(-0.707106781186529,0.,-0.707106781186566));
#129861=DIRECTION('center_axis',(0.,-1.,0.));
#129862=DIRECTION('ref_axis',(-0.707106781186547,0.,0.707106781186548));
#129863=DIRECTION('',(0.,-1.,0.));
#129864=DIRECTION('center_axis',(0.,1.,0.));
#129865=DIRECTION('ref_axis',(-0.707106781186547,0.,0.707106781186548));
#129866=DIRECTION('center_axis',(0.,-1.,0.));
#129867=DIRECTION('ref_axis',(-0.707106781186547,0.,0.707106781186548));
#129868=DIRECTION('',(0.,-1.,0.));
#129869=DIRECTION('center_axis',(0.,1.,0.));
#129870=DIRECTION('ref_axis',(-0.707106781186547,0.,0.707106781186548));
#129871=DIRECTION('center_axis',(0.,-1.,0.));
#129872=DIRECTION('ref_axis',(-0.707106781186547,0.,0.707106781186548));
#129873=DIRECTION('',(0.,-1.,0.));
#129874=DIRECTION('center_axis',(0.,-1.,0.));
#129875=DIRECTION('ref_axis',(-0.707106781186547,0.,0.707106781186548));
#129876=DIRECTION('',(0.,-1.,0.));
#129877=DIRECTION('center_axis',(0.,-1.,0.));
#129878=DIRECTION('ref_axis',(-0.707106781186547,0.,0.707106781186548));
#129879=DIRECTION('',(0.,-1.,0.));
#129880=DIRECTION('center_axis',(0.,-1.,0.));
#129881=DIRECTION('ref_axis',(-0.707106781186547,0.,0.707106781186548));
#129882=DIRECTION('',(0.,-1.,0.));
#129883=DIRECTION('center_axis',(0.,-1.,0.));
#129884=DIRECTION('ref_axis',(-0.707106781186547,0.,0.707106781186548));
#129885=DIRECTION('',(0.,-1.,0.));
#129886=DIRECTION('center_axis',(0.,-1.,0.));
#129887=DIRECTION('ref_axis',(-0.912105596603152,0.,0.409955339817897));
#129888=DIRECTION('',(0.,-1.,0.));
#129889=DIRECTION('center_axis',(0.,-1.,0.));
#129890=DIRECTION('ref_axis',(-0.707106781186547,0.,0.707106781186548));
#129891=DIRECTION('center_axis',(0.,-1.,0.));
#129892=DIRECTION('ref_axis',(0.537039752331291,0.,0.843556936084308));
#129893=DIRECTION('',(-8.65956056235516E-17,-1.,8.6595605623547E-17));
#129894=DIRECTION('center_axis',(0.,1.,0.));
#129895=DIRECTION('ref_axis',(-0.707106781186566,0.,0.707106781186529));
#129896=DIRECTION('center_axis',(0.,-1.,0.));
#129897=DIRECTION('ref_axis',(-0.707106781186566,0.,0.707106781186529));
#129898=DIRECTION('',(-8.65956056235516E-17,-1.,8.6595605623547E-17));
#129899=DIRECTION('center_axis',(0.,-1.,0.));
#129900=DIRECTION('ref_axis',(-0.707106781186566,0.,0.707106781186529));
#129901=DIRECTION('',(-8.65956056235516E-17,-1.,8.6595605623547E-17));
#129902=DIRECTION('center_axis',(0.,-1.,0.));
#129903=DIRECTION('ref_axis',(-0.707106781186566,0.,0.707106781186529));
#129904=DIRECTION('',(-8.65956056235516E-17,-1.,8.6595605623547E-17));
#129905=DIRECTION('center_axis',(0.,-1.,0.));
#129906=DIRECTION('ref_axis',(-0.707106781186566,0.,0.707106781186529));
#129907=DIRECTION('',(-8.65956056235516E-17,-1.,8.6595605623547E-17));
#129908=DIRECTION('center_axis',(0.,-1.,0.));
#129909=DIRECTION('ref_axis',(-0.707106781186566,0.,0.707106781186529));
#129910=DIRECTION('',(-8.65956056235516E-17,-1.,8.6595605623547E-17));
#129911=DIRECTION('center_axis',(0.,-1.,0.));
#129912=DIRECTION('ref_axis',(-0.707106781186566,0.,0.707106781186529));
#129913=DIRECTION('',(-8.65956056235516E-17,-1.,8.6595605623547E-17));
#129914=DIRECTION('center_axis',(0.,-1.,0.));
#129915=DIRECTION('ref_axis',(-0.130813539470888,0.,-0.991406989026756));
#129916=DIRECTION('',(-8.65956056235516E-17,-1.,8.6595605623547E-17));
#129917=DIRECTION('center_axis',(0.,-1.,0.));
#129918=DIRECTION('ref_axis',(-0.707106781186566,0.,0.707106781186529));
#129919=DIRECTION('center_axis',(0.,1.,0.));
#129920=DIRECTION('ref_axis',(0.707106781186548,0.,0.707106781186547));
#129921=DIRECTION('center_axis',(0.,1.,0.));
#129922=DIRECTION('ref_axis',(0.707106781186548,0.,0.707106781186547));
#129923=DIRECTION('',(0.500000000000002,-0.707106781186545,0.500000000000001));
#129924=DIRECTION('center_axis',(0.,-1.,0.));
#129925=DIRECTION('ref_axis',(0.707106781186548,0.,0.707106781186547));
#129926=DIRECTION('center_axis',(0.,1.,0.));
#129927=DIRECTION('ref_axis',(0.707106781186548,0.,0.707106781186547));
#129928=DIRECTION('center_axis',(0.,-1.,0.));
#129929=DIRECTION('ref_axis',(-0.707106781186548,0.,-0.707106781186547));
#129930=DIRECTION('center_axis',(0.,-1.,0.));
#129931=DIRECTION('ref_axis',(-0.707106781186548,0.,-0.707106781186547));
#129932=DIRECTION('',(0.,1.,0.));
#129933=DIRECTION('center_axis',(0.,1.,0.));
#129934=DIRECTION('ref_axis',(0.707106781186548,0.,0.707106781186547));
#129935=DIRECTION('center_axis',(0.,-1.,0.));
#129936=DIRECTION('ref_axis',(-0.707106781186548,0.,-0.707106781186547));
#129937=DIRECTION('center_axis',(0.,-1.,0.));
#129938=DIRECTION('ref_axis',(-0.707106781186566,0.,0.707106781186529));
#129939=DIRECTION('center_axis',(0.,-1.,0.));
#129940=DIRECTION('ref_axis',(-0.707106781186548,0.,-0.707106781186547));
#129941=DIRECTION('center_axis',(0.,1.,0.));
#129942=DIRECTION('ref_axis',(-0.707106781186548,0.,-0.707106781186547));
#129943=DIRECTION('center_axis',(0.,-1.,0.));
#129944=DIRECTION('ref_axis',(-0.707106781186548,0.,-0.707106781186547));
#129945=DIRECTION('center_axis',(0.,-1.,0.));
#129946=DIRECTION('ref_axis',(-0.707106781186547,0.,0.707106781186548));
#129947=DIRECTION('center_axis',(0.,-1.,0.));
#129948=DIRECTION('ref_axis',(-0.707106781186548,0.,-0.707106781186547));
#129949=DIRECTION('center_axis',(0.,-1.,0.));
#129950=DIRECTION('ref_axis',(-0.707106781186548,0.,-0.707106781186547));
#129951=DIRECTION('',(0.,1.,0.));
#129952=DIRECTION('center_axis',(0.,1.,0.));
#129953=DIRECTION('ref_axis',(-0.707106781186548,0.,-0.707106781186547));
#129954=DIRECTION('center_axis',(0.,-1.,0.));
#129955=DIRECTION('ref_axis',(-0.707106781186548,0.,-0.707106781186548));
#129956=DIRECTION('',(0.500000000000003,-0.707106781186543,0.500000000000003));
#129957=DIRECTION('center_axis',(0.,1.,0.));
#129958=DIRECTION('ref_axis',(-0.707106781186548,0.,-0.707106781186547));
#129959=DIRECTION('center_axis',(0.,-1.,0.));
#129960=DIRECTION('ref_axis',(-0.707106781186548,0.,-0.707106781186547));
#129961=DIRECTION('',(0.,-1.,0.));
#129962=DIRECTION('center_axis',(0.,-1.,0.));
#129963=DIRECTION('ref_axis',(-0.707106781186548,0.,-0.707106781186547));
#129964=DIRECTION('center_axis',(0.,-1.,0.));
#129965=DIRECTION('ref_axis',(-0.707106781186548,0.,-0.707106781186547));
#129966=DIRECTION('center_axis',(0.,1.,0.));
#129967=DIRECTION('ref_axis',(-0.707106781186548,0.,-0.707106781186547));
#129968=DIRECTION('',(0.,1.,0.));
#129969=DIRECTION('center_axis',(0.,-1.,0.));
#129970=DIRECTION('ref_axis',(-0.707106781186548,0.,-0.707106781186547));
#129971=DIRECTION('',(0.,1.,0.));
#129972=DIRECTION('center_axis',(0.,-1.,0.));
#129973=DIRECTION('ref_axis',(-0.707106781186548,0.,-0.707106781186547));
#129974=DIRECTION('center_axis',(0.,-1.,0.));
#129975=DIRECTION('ref_axis',(-0.707106781186548,0.,-0.707106781186547));
#129976=DIRECTION('center_axis',(0.,-1.,0.));
#129977=DIRECTION('ref_axis',(-0.707106781186548,0.,-0.707106781186547));
#129978=DIRECTION('',(0.,1.,0.));
#129979=DIRECTION('center_axis',(0.,-1.,0.));
#129980=DIRECTION('ref_axis',(-0.707106781186548,0.,-0.707106781186547));
#129981=DIRECTION('center_axis',(0.,1.,0.));
#129982=DIRECTION('ref_axis',(-0.707106781186548,0.,-0.707106781186547));
#129983=DIRECTION('',(0.,1.,0.));
#129984=DIRECTION('center_axis',(0.,-1.,0.));
#129985=DIRECTION('ref_axis',(-0.707106781186548,0.,-0.707106781186547));
#129986=DIRECTION('center_axis',(0.,-1.,0.));
#129987=DIRECTION('ref_axis',(-0.707106781186548,0.,-0.707106781186547));
#129988=DIRECTION('center_axis',(0.,-1.,0.));
#129989=DIRECTION('ref_axis',(-0.707106781186548,0.,-0.707106781186547));
#129990=DIRECTION('',(0.,1.,0.));
#129991=DIRECTION('center_axis',(0.,-1.,0.));
#129992=DIRECTION('ref_axis',(-0.707106781186548,0.,-0.707106781186547));
#129993=DIRECTION('center_axis',(0.,-1.,0.));
#129994=DIRECTION('ref_axis',(-0.707106781186548,0.,-0.707106781186547));
#129995=DIRECTION('center_axis',(0.,1.,0.));
#129996=DIRECTION('ref_axis',(-0.707106781186548,0.,-0.707106781186547));
#129997=DIRECTION('',(0.,1.,0.));
#129998=DIRECTION('center_axis',(0.,-1.,0.));
#129999=DIRECTION('ref_axis',(-0.707106781186548,0.,-0.707106781186547));
#130000=DIRECTION('center_axis',(0.,-1.,0.));
#130001=DIRECTION('ref_axis',(-0.707106781186548,0.,-0.707106781186547));
#130002=DIRECTION('center_axis',(0.,-1.,0.));
#130003=DIRECTION('ref_axis',(-0.707106781186548,0.,-0.707106781186547));
#130004=DIRECTION('',(0.,1.,0.));
#130005=DIRECTION('center_axis',(0.,-1.,0.));
#130006=DIRECTION('ref_axis',(-0.707106781186548,0.,-0.707106781186547));
#130007=DIRECTION('center_axis',(0.,-1.,0.));
#130008=DIRECTION('ref_axis',(-0.707106781186548,0.,-0.707106781186547));
#130009=DIRECTION('center_axis',(0.,1.,0.));
#130010=DIRECTION('ref_axis',(-0.707106781186548,0.,-0.707106781186547));
#130011=DIRECTION('',(0.,1.,0.));
#130012=DIRECTION('center_axis',(0.,-1.,0.));
#130013=DIRECTION('ref_axis',(-0.707106781186548,0.,-0.707106781186547));
#130014=DIRECTION('center_axis',(0.,-1.,0.));
#130015=DIRECTION('ref_axis',(-0.707106781186548,0.,-0.707106781186547));
#130016=DIRECTION('center_axis',(0.,-1.,0.));
#130017=DIRECTION('ref_axis',(-0.707106781186548,0.,-0.707106781186547));
#130018=DIRECTION('',(0.,1.,0.));
#130019=DIRECTION('center_axis',(0.,-1.,0.));
#130020=DIRECTION('ref_axis',(-0.707106781186548,0.,-0.707106781186547));
#130021=DIRECTION('center_axis',(0.,-1.,0.));
#130022=DIRECTION('ref_axis',(-0.707106781186548,0.,-0.707106781186547));
#130023=DIRECTION('center_axis',(0.,1.,0.));
#130024=DIRECTION('ref_axis',(-0.707106781186548,0.,-0.707106781186547));
#130025=DIRECTION('',(0.,1.,0.));
#130026=DIRECTION('center_axis',(0.,-1.,0.));
#130027=DIRECTION('ref_axis',(-0.707106781186548,0.,-0.707106781186547));
#130028=DIRECTION('center_axis',(0.,-1.,0.));
#130029=DIRECTION('ref_axis',(-0.707106781186548,0.,-0.707106781186547));
#130030=DIRECTION('center_axis',(0.,-1.,0.));
#130031=DIRECTION('ref_axis',(-0.707106781186548,0.,-0.707106781186547));
#130032=DIRECTION('',(0.,1.,0.));
#130033=DIRECTION('center_axis',(0.,-1.,0.));
#130034=DIRECTION('ref_axis',(-0.707106781186548,0.,-0.707106781186547));
#130035=DIRECTION('center_axis',(0.,-1.,0.));
#130036=DIRECTION('ref_axis',(-0.707106781186548,0.,-0.707106781186547));
#130037=DIRECTION('center_axis',(0.,1.,0.));
#130038=DIRECTION('ref_axis',(-0.707106781186548,0.,-0.707106781186547));
#130039=DIRECTION('',(0.,1.,0.));
#130040=DIRECTION('center_axis',(0.,-1.,0.));
#130041=DIRECTION('ref_axis',(-0.707106781186548,0.,-0.707106781186547));
#130042=DIRECTION('center_axis',(0.,-1.,0.));
#130043=DIRECTION('ref_axis',(-0.707106781186548,0.,-0.707106781186547));
#130044=DIRECTION('center_axis',(0.,-1.,0.));
#130045=DIRECTION('ref_axis',(-0.707106781186548,0.,-0.707106781186547));
#130046=DIRECTION('',(0.,1.,0.));
#130047=DIRECTION('center_axis',(0.,-1.,0.));
#130048=DIRECTION('ref_axis',(-0.707106781186548,0.,-0.707106781186547));
#130049=DIRECTION('center_axis',(0.,-1.,0.));
#130050=DIRECTION('ref_axis',(-0.707106781186548,0.,-0.707106781186547));
#130051=DIRECTION('center_axis',(0.,1.,0.));
#130052=DIRECTION('ref_axis',(-0.707106781186548,0.,-0.707106781186547));
#130053=DIRECTION('',(0.,1.,0.));
#130054=DIRECTION('center_axis',(0.,-1.,0.));
#130055=DIRECTION('ref_axis',(-0.707106781186548,0.,-0.707106781186547));
#130056=DIRECTION('center_axis',(0.,-1.,0.));
#130057=DIRECTION('ref_axis',(-0.707106781186548,0.,-0.707106781186547));
#130058=DIRECTION('center_axis',(0.,-1.,0.));
#130059=DIRECTION('ref_axis',(-0.707106781186548,0.,-0.707106781186547));
#130060=DIRECTION('',(0.,1.,0.));
#130061=DIRECTION('center_axis',(0.,-1.,0.));
#130062=DIRECTION('ref_axis',(-0.707106781186548,0.,-0.707106781186547));
#130063=DIRECTION('center_axis',(0.,-1.,0.));
#130064=DIRECTION('ref_axis',(-0.707106781186548,0.,-0.707106781186547));
#130065=DIRECTION('center_axis',(0.,1.,0.));
#130066=DIRECTION('ref_axis',(-0.707106781186548,0.,-0.707106781186547));
#130067=DIRECTION('',(0.,1.,0.));
#130068=DIRECTION('center_axis',(0.,-1.,0.));
#130069=DIRECTION('ref_axis',(-0.707106781186548,0.,-0.707106781186547));
#130070=DIRECTION('center_axis',(0.,-1.,0.));
#130071=DIRECTION('ref_axis',(-0.707106781186548,0.,-0.707106781186547));
#130072=DIRECTION('center_axis',(0.,-1.,0.));
#130073=DIRECTION('ref_axis',(-0.707106781186548,0.,-0.707106781186547));
#130074=DIRECTION('',(0.,1.,0.));
#130075=DIRECTION('center_axis',(0.,-1.,0.));
#130076=DIRECTION('ref_axis',(-0.707106781186548,0.,-0.707106781186547));
#130077=DIRECTION('center_axis',(0.,-1.,0.));
#130078=DIRECTION('ref_axis',(-0.707106781186548,0.,-0.707106781186547));
#130079=DIRECTION('center_axis',(0.,1.,0.));
#130080=DIRECTION('ref_axis',(-0.707106781186548,0.,-0.707106781186547));
#130081=DIRECTION('',(0.,1.,0.));
#130082=DIRECTION('center_axis',(0.,-1.,0.));
#130083=DIRECTION('ref_axis',(-0.707106781186548,0.,-0.707106781186547));
#130084=DIRECTION('center_axis',(0.,-1.,0.));
#130085=DIRECTION('ref_axis',(-0.707106781186548,0.,-0.707106781186547));
#130086=DIRECTION('center_axis',(0.,-1.,0.));
#130087=DIRECTION('ref_axis',(-0.707106781186548,0.,-0.707106781186547));
#130088=DIRECTION('',(0.,1.,0.));
#130089=DIRECTION('center_axis',(0.,-1.,0.));
#130090=DIRECTION('ref_axis',(-0.707106781186548,0.,-0.707106781186547));
#130091=DIRECTION('center_axis',(0.,-1.,0.));
#130092=DIRECTION('ref_axis',(-0.707106781186548,0.,-0.707106781186547));
#130093=DIRECTION('center_axis',(0.,1.,0.));
#130094=DIRECTION('ref_axis',(-0.707106781186548,0.,-0.707106781186547));
#130095=DIRECTION('',(0.,1.,0.));
#130096=DIRECTION('center_axis',(0.,-1.,0.));
#130097=DIRECTION('ref_axis',(-0.707106781186548,0.,-0.707106781186547));
#130098=DIRECTION('center_axis',(0.,-1.,0.));
#130099=DIRECTION('ref_axis',(-0.707106781186548,0.,-0.707106781186547));
#130100=DIRECTION('center_axis',(0.,1.,0.));
#130101=DIRECTION('ref_axis',(0.707106781186548,0.,0.707106781186547));
#130102=DIRECTION('center_axis',(0.,-1.,0.));
#130103=DIRECTION('ref_axis',(-0.707106781186548,0.,-0.707106781186547));
#130104=DIRECTION('center_axis',(0.,1.,0.));
#130105=DIRECTION('ref_axis',(0.707106781186548,0.,0.707106781186547));
#130106=DIRECTION('center_axis',(0.,-1.,0.));
#130107=DIRECTION('ref_axis',(-0.707106781186548,0.,-0.707106781186547));
#130108=DIRECTION('center_axis',(0.,1.,0.));
#130109=DIRECTION('ref_axis',(0.707106781186548,0.,0.707106781186547));
#130110=DIRECTION('center_axis',(0.,-1.,0.));
#130111=DIRECTION('ref_axis',(-0.707106781186548,0.,-0.707106781186547));
#130112=DIRECTION('center_axis',(0.,1.,0.));
#130113=DIRECTION('ref_axis',(0.707106781186548,0.,0.707106781186547));
#130114=DIRECTION('center_axis',(0.,-1.,0.));
#130115=DIRECTION('ref_axis',(-0.707106781186548,0.,-0.707106781186547));
#130116=DIRECTION('center_axis',(0.,1.,0.));
#130117=DIRECTION('ref_axis',(0.707106781186548,0.,0.707106781186547));
#130118=DIRECTION('center_axis',(0.,-1.,0.));
#130119=DIRECTION('ref_axis',(-0.707106781186548,0.,-0.707106781186547));
#130120=DIRECTION('center_axis',(0.,1.,0.));
#130121=DIRECTION('ref_axis',(0.707106781186548,0.,0.707106781186547));
#130122=DIRECTION('center_axis',(0.,-1.,0.));
#130123=DIRECTION('ref_axis',(-0.707106781186548,0.,-0.707106781186547));
#130124=DIRECTION('center_axis',(0.,1.,0.));
#130125=DIRECTION('ref_axis',(0.707106781186548,0.,0.707106781186547));
#130126=DIRECTION('center_axis',(0.,-1.,0.));
#130127=DIRECTION('ref_axis',(-0.707106781186548,0.,-0.707106781186547));
#130128=DIRECTION('center_axis',(0.,1.,0.));
#130129=DIRECTION('ref_axis',(0.707106781186548,0.,0.707106781186547));
#130130=DIRECTION('center_axis',(0.,-1.,0.));
#130131=DIRECTION('ref_axis',(-0.707106781186548,0.,-0.707106781186547));
#130132=DIRECTION('center_axis',(0.,1.,0.));
#130133=DIRECTION('ref_axis',(0.707106781186548,0.,0.707106781186547));
#130134=DIRECTION('center_axis',(0.,1.,0.));
#130135=DIRECTION('ref_axis',(0.707106781186548,0.,0.707106781186547));
#130136=DIRECTION('center_axis',(0.,-1.,0.));
#130137=DIRECTION('ref_axis',(-0.707106781186548,0.,-0.707106781186547));
#130138=DIRECTION('center_axis',(0.,-1.,0.));
#130139=DIRECTION('ref_axis',(-0.707106781186529,0.,-0.707106781186566));
#130140=DIRECTION('center_axis',(0.,-1.,0.));
#130141=DIRECTION('ref_axis',(-0.707106781186548,0.,-0.707106781186547));
#130142=DIRECTION('center_axis',(0.,-1.,0.));
#130143=DIRECTION('ref_axis',(0.707106781186566,0.,-0.707106781186529));
#130144=DIRECTION('center_axis',(0.,-1.,0.));
#130145=DIRECTION('ref_axis',(0.707106781186547,0.,-0.707106781186548));
#130146=DIRECTION('center_axis',(0.,-1.,0.));
#130147=DIRECTION('ref_axis',(0.707106781186529,0.,0.707106781186566));
#130148=DIRECTION('center_axis',(0.,-1.,0.));
#130149=DIRECTION('ref_axis',(0.707106781186548,0.,0.707106781186547));
#449392=CARTESIAN_POINT('',(0.,0.,0.));
#449393=CARTESIAN_POINT('Origin',(5.65685387860011,26.,-5.65685387860012));
#449394=CARTESIAN_POINT('',(4.9222125558517,22.573038475773,-6.39190072013885));
#449395=CARTESIAN_POINT('',(4.92305381642377,22.5,-6.39065394077646));
#449396=CARTESIAN_POINT('',(4.92305381642377,26.,-6.39065394077646));
#449397=CARTESIAN_POINT('',(5.8978925564917,22.5,-6.66622270032004));
#449398=CARTESIAN_POINT('Origin',(5.65685387860011,22.5,-5.65685387860012));
#449399=CARTESIAN_POINT('Ctrl Pts',(5.89851203167784,22.5,-6.66798006829997));
#449400=CARTESIAN_POINT('Ctrl Pts',(5.5764199513446,22.5229375355598,-6.7439998684947));
#449401=CARTESIAN_POINT('Ctrl Pts',(5.21379162224851,22.5458750711197,-6.65366449057419));
#449402=CARTESIAN_POINT('Ctrl Pts',(4.96646199655034,22.5688126066795,-6.43383171727969));
#449403=CARTESIAN_POINT('Ctrl Pts',(4.95127317183385,22.5702212297106,-6.42033150900063));
#449404=CARTESIAN_POINT('Ctrl Pts',(4.93651917810251,22.5716298527418,-6.40634292159547));
#449405=CARTESIAN_POINT('Ctrl Pts',(4.9222125558517,22.573038475773,-6.39190072013885));
#449406=CARTESIAN_POINT('Origin',(5.65685387860011,26.,-5.65685387860012));
#449407=CARTESIAN_POINT('',(4.92436540268704,23.0230384757729,-6.39037461032892));
#449408=CARTESIAN_POINT('',(4.92349966353597,22.9019615242271,-6.38930388760559));
#449409=CARTESIAN_POINT('',(4.92305381642377,26.,-6.39065394077646));
#449410=CARTESIAN_POINT('',(4.62591736201901,22.5,-5.77557608073439));
#449411=CARTESIAN_POINT('Ctrl Pts',(4.92349966353597,22.9019615242271,-6.38930388760559));
#449412=CARTESIAN_POINT('Ctrl Pts',(5.07692511110986,22.8871128006417,-6.54102880287524));
#449413=CARTESIAN_POINT('Ctrl Pts',(5.27640120658105,22.8722640770563,-6.64766299899898));
#449414=CARTESIAN_POINT('Ctrl Pts',(5.48772889025785,22.8574153534709,-6.68249361011691));
#449415=CARTESIAN_POINT('Ctrl Pts',(5.82684562005693,22.8335876632395,-6.73838615923167));
#449416=CARTESIAN_POINT('Ctrl Pts',(6.19648078060475,22.8097599730081,-6.60938089562333));
#449417=CARTESIAN_POINT('Ctrl Pts',(6.42720821100081,22.7859322827767,-6.35472685290066));
#449418=CARTESIAN_POINT('Ctrl Pts',(6.65793564139688,22.7621045925453,-6.10007281017799));
#449419=CARTESIAN_POINT('Ctrl Pts',(6.74975534164119,22.7382769023139,-5.71976998834099));
#449420=CARTESIAN_POINT('Ctrl Pts',(6.66080060824128,22.7144492120825,-5.38773213421059));
#449421=CARTESIAN_POINT('Ctrl Pts',(6.57184587484137,22.6906215218511,-5.05569428008018));
#449422=CARTESIAN_POINT('Ctrl Pts',(6.30211670779724,22.6667938316197,-4.77192139365638));
#449423=CARTESIAN_POINT('Ctrl Pts',(5.97477550103877,22.6429661413884,-4.66700870222797));
#449424=CARTESIAN_POINT('Ctrl Pts',(5.6474342942803,22.619138451157,-4.56209601079956));
#449425=CARTESIAN_POINT('Ctrl Pts',(5.26248104780748,22.5953107609256,-4.63604351436656));
#449426=CARTESIAN_POINT('Ctrl Pts',(4.99722717517853,22.5714830706942,-4.85366607828882));
#449427=CARTESIAN_POINT('Ctrl Pts',(4.73197330254959,22.5476553804628,-5.07128864221107));
#449428=CARTESIAN_POINT('Ctrl Pts',(4.58641880376449,22.5238276902314,-5.43258626648858));
#449429=CARTESIAN_POINT('Ctrl Pts',(4.625917362019,22.5,-5.77557608073438));
#449430=CARTESIAN_POINT('Origin',(5.65685387860011,22.5,-5.65685387860012));
#449431=CARTESIAN_POINT('Ctrl Pts',(4.9222125558517,22.573038475773,-6.39190072013885));
#449432=CARTESIAN_POINT('Ctrl Pts',(4.69451421601594,22.5954575429732,-6.16204455719575));
#449433=CARTESIAN_POINT('Ctrl Pts',(4.58013776446742,22.6178766101734,-5.81728522517979));
#449434=CARTESIAN_POINT('Ctrl Pts',(4.62964039434809,22.6402956773736,-5.49777863793003));
#449435=CARTESIAN_POINT('Ctrl Pts',(4.68225334741615,22.664123367605,-5.15819698094666));
#449436=CARTESIAN_POINT('Ctrl Pts',(4.91998587117151,22.6879510578364,-4.8471410957032));
#449437=CARTESIAN_POINT('Ctrl Pts',(5.23393572436938,22.7117787480678,-4.70728537400252));
#449438=CARTESIAN_POINT('Ctrl Pts',(5.54788557756724,22.7356064382992,-4.56742965230184));
#449439=CARTESIAN_POINT('Ctrl Pts',(5.93805276020761,22.7594341285306,-4.59877409414395));
#449440=CARTESIAN_POINT('Ctrl Pts',(6.22570363532513,22.783261818762,-4.78686738296995));
#449441=CARTESIAN_POINT('Ctrl Pts',(6.51335451044265,22.8070895089934,-4.97496067179595));
#449442=CARTESIAN_POINT('Ctrl Pts',(6.69848907803731,22.8309171992248,-5.31980280760584));
#449443=CARTESIAN_POINT('Ctrl Pts',(6.69629884619592,22.8547448894562,-5.66347121722023));
#449444=CARTESIAN_POINT('Ctrl Pts',(6.69410861435453,22.8785725796876,-6.00713962683461));
#449445=CARTESIAN_POINT('Ctrl Pts',(6.5045935830771,22.902400269919,-6.34963431025348));
#449446=CARTESIAN_POINT('Ctrl Pts',(6.21456908983246,22.9262279601503,-6.53403672593788));
#449447=CARTESIAN_POINT('Ctrl Pts',(5.92454459658782,22.9500556503817,-6.71843914162228));
#449448=CARTESIAN_POINT('Ctrl Pts',(5.53401064137597,22.9738833406131,-6.7447492895722));
#449449=CARTESIAN_POINT('Ctrl Pts',(5.22186823831326,22.9977110308445,-6.60092695407667));
#449450=CARTESIAN_POINT('Ctrl Pts',(5.11127184889382,23.0061535124873,-6.54996870275417));
#449451=CARTESIAN_POINT('Ctrl Pts',(5.0105166042882,23.0145959941301,-6.47765230299322));
#449452=CARTESIAN_POINT('Ctrl Pts',(4.92436540268704,23.0230384757729,-6.39037461032892));
#449453=CARTESIAN_POINT('Origin',(5.65685387860011,26.,-5.65685387860012));
#449454=CARTESIAN_POINT('',(4.92330089590042,23.4730384757729,-6.38935290488262));
#449455=CARTESIAN_POINT('',(4.92169609601798,23.3519615242271,-6.3913110357232));
#449456=CARTESIAN_POINT('',(4.92305381642377,26.,-6.39065394077646));
#449457=CARTESIAN_POINT('Ctrl Pts',(4.92169609601798,23.3519615242271,-6.3913110357232));
#449458=CARTESIAN_POINT('Ctrl Pts',(5.14636061012976,23.33007894203,-6.61334324490838));
#449459=CARTESIAN_POINT('Ctrl Pts',(5.47994522249351,23.308196359833,-6.72868171719176));
#449460=CARTESIAN_POINT('Ctrl Pts',(5.79285848911253,23.286313777636,-6.68738448495221));
#449461=CARTESIAN_POINT('Ctrl Pts',(6.1335861198444,23.2624860874046,-6.64241640721999));
#449462=CARTESIAN_POINT('Ctrl Pts',(6.44980419113038,23.2386583971732,-6.41172882390928));
#449463=CARTESIAN_POINT('Ctrl Pts',(6.59665364733223,23.2148307069418,-6.10100080909856));
#449464=CARTESIAN_POINT('Ctrl Pts',(6.74350310353408,23.1910030167104,-5.79027279428784));
#449465=CARTESIAN_POINT('Ctrl Pts',(6.7209839446518,23.167175326479,-5.39950434797711));
#449466=CARTESIAN_POINT('Ctrl Pts',(6.539415444341,23.1433476362476,-5.1076985472349));
#449467=CARTESIAN_POINT('Ctrl Pts',(6.3578469440302,23.1195199460162,-4.8158927464927));
#449468=CARTESIAN_POINT('Ctrl Pts',(6.01722910229088,23.0956922557848,-4.62304959131903));
#449469=CARTESIAN_POINT('Ctrl Pts',(5.67358993507176,23.0718645655534,-4.61751951301592));
#449470=CARTESIAN_POINT('Ctrl Pts',(5.32995076785264,23.048036875322,-4.61198943471281));
#449471=CARTESIAN_POINT('Ctrl Pts',(4.98329027515371,23.0242091850907,-4.79377243328026));
#449472=CARTESIAN_POINT('Ctrl Pts',(4.7924243254548,23.0003814948593,-5.07957475014376));
#449473=CARTESIAN_POINT('Ctrl Pts',(4.60155837575589,22.9765538046279,-5.36537706700727));
#449474=CARTESIAN_POINT('Ctrl Pts',(4.56648696905699,22.9527261143965,-5.75519870216683));
#449475=CARTESIAN_POINT('Ctrl Pts',(4.70325041523271,22.9288984241651,-6.07050470066555));
#449476=CARTESIAN_POINT('Ctrl Pts',(4.75478685916323,22.9199194575191,-6.18932117076026));
#449477=CARTESIAN_POINT('Ctrl Pts',(4.830723879241,22.9109404908731,-6.29755640872372));
#449478=CARTESIAN_POINT('Ctrl Pts',(4.92349966353597,22.9019615242271,-6.38930388760559));
#449479=CARTESIAN_POINT('Ctrl Pts',(4.92436540268704,23.0230384757729,-6.39037461032892));
#449480=CARTESIAN_POINT('Ctrl Pts',(4.76736722811336,23.0384236843615,-6.23132356780567));
#449481=CARTESIAN_POINT('Ctrl Pts',(4.65886881811934,23.0538088929501,-6.02258634020352));
#449482=CARTESIAN_POINT('Ctrl Pts',(4.62769529041208,23.0691941015387,-5.80287677492702));
#449483=CARTESIAN_POINT('Ctrl Pts',(4.57941559648716,23.0930217917701,-5.46260375021388));
#449484=CARTESIAN_POINT('Ctrl Pts',(4.71660705955086,23.1168494820015,-5.09601251972857));
#449485=CARTESIAN_POINT('Ctrl Pts',(4.97642324075838,23.1406771722329,-4.87103919530453));
#449486=CARTESIAN_POINT('Ctrl Pts',(5.23623942196589,23.1645048624643,-4.64606587088049));
#449487=CARTESIAN_POINT('Ctrl Pts',(5.61868032131722,23.1883325526957,-4.56271045251773));
#449488=CARTESIAN_POINT('Ctrl Pts',(5.94855238336812,23.2121602429271,-4.65915585483332));
#449489=CARTESIAN_POINT('Ctrl Pts',(6.27842444541901,23.2359879331585,-4.75560125714891));
#449490=CARTESIAN_POINT('Ctrl Pts',(6.55572767016945,23.2598156233899,-5.03184748014285));
#449491=CARTESIAN_POINT('Ctrl Pts',(6.65343136663416,23.2836433136212,-5.36134886181892));
#449492=CARTESIAN_POINT('Ctrl Pts',(6.75113506309887,23.3074710038526,-5.690850243495));
#449493=CARTESIAN_POINT('Ctrl Pts',(6.66923923127783,23.331298694084,-6.07360678385322));
#449494=CARTESIAN_POINT('Ctrl Pts',(6.4452597843657,23.3551263843154,-6.33427992409048));
#449495=CARTESIAN_POINT('Ctrl Pts',(6.22128033745358,23.3789540745468,-6.59495306432775));
#449496=CARTESIAN_POINT('Ctrl Pts',(5.85521727545038,23.4027817647782,-6.73354280444407));
#449497=CARTESIAN_POINT('Ctrl Pts',(5.51476156795534,23.4266094550096,-6.6865623548039));
#449498=CARTESIAN_POINT('Ctrl Pts',(5.29363193601897,23.442085795264,-6.65604804910002));
#449499=CARTESIAN_POINT('Ctrl Pts',(5.08330512959901,23.4575621355185,-6.54724832815155));
#449500=CARTESIAN_POINT('Ctrl Pts',(4.92330089590042,23.4730384757729,-6.38935290488262));
#449501=CARTESIAN_POINT('Origin',(5.65685387860011,26.,-5.65685387860012));
#449502=CARTESIAN_POINT('',(4.9216948349357,23.9230384757729,-6.39152331859132));
#449503=CARTESIAN_POINT('',(4.92356615355223,23.8019615242271,-6.39146732321148));
#449504=CARTESIAN_POINT('',(4.92305381642377,26.,-6.39065394077646));
#449505=CARTESIAN_POINT('Ctrl Pts',(4.92356615355223,23.8019615242271,-6.39146732321148));
#449506=CARTESIAN_POINT('Ctrl Pts',(4.97518123721477,23.7968727736498,-6.44404636753914));
#449507=CARTESIAN_POINT('Ctrl Pts',(5.03225965778749,23.7917840230725,-6.49097569651667));
#449508=CARTESIAN_POINT('Ctrl Pts',(5.09396482100832,23.7866952724952,-6.53072214720976));
#449509=CARTESIAN_POINT('Ctrl Pts',(5.38289458727869,23.7628675822638,-6.71683190058211));
#449510=CARTESIAN_POINT('Ctrl Pts',(5.77326614382955,23.7390398920324,-6.74545633697037));
#449511=CARTESIAN_POINT('Ctrl Pts',(6.08625298439034,23.715212201801,-6.60348277515141));
#449512=CARTESIAN_POINT('Ctrl Pts',(6.39923982495114,23.6913845115696,-6.46150921333244));
#449513=CARTESIAN_POINT('Ctrl Pts',(6.63484194952187,23.6675568213382,-6.14893765330626));
#449514=CARTESIAN_POINT('Ctrl Pts',(6.68513161677842,23.6437291311068,-5.80895502137128));
#449515=CARTESIAN_POINT('Ctrl Pts',(6.73542128403497,23.6199014408755,-5.4689723894363));
#449516=CARTESIAN_POINT('Ctrl Pts',(6.60039849397735,23.5960737506441,-5.10157868559252));
#449517=CARTESIAN_POINT('Ctrl Pts',(6.34191631672375,23.5722460604127,-4.87507434314934));
#449518=CARTESIAN_POINT('Ctrl Pts',(6.08343413947014,23.5484183701813,-4.64857000070616));
#449519=CARTESIAN_POINT('Ctrl Pts',(5.70149257502055,23.5245906799499,-4.56295501966359));
#449520=CARTESIAN_POINT('Ctrl Pts',(5.37105630657982,23.5007629897185,-4.65744921450722));
#449521=CARTESIAN_POINT('Ctrl Pts',(5.04062003813909,23.4769352994871,-4.75194340935084));
#449522=CARTESIAN_POINT('Ctrl Pts',(4.76168906570723,23.4531076092557,-5.02654678008065));
#449523=CARTESIAN_POINT('Ctrl Pts',(4.66203997694959,23.4292799190243,-5.35546505814245));
#449524=CARTESIAN_POINT('Ctrl Pts',(4.56239088819195,23.4054522287929,-5.68438333620426));
#449525=CARTESIAN_POINT('Ctrl Pts',(4.64202368310855,23.3816245385615,-6.06761652159808));
#449526=CARTESIAN_POINT('Ctrl Pts',(4.86445867565572,23.3577968483301,-6.32960882821811));
#449527=CARTESIAN_POINT('Ctrl Pts',(4.88261654521522,23.3558517402958,-6.350995850443));
#449528=CARTESIAN_POINT('Ctrl Pts',(4.90172602358781,23.3539066322614,-6.37157494470416));
#449529=CARTESIAN_POINT('Ctrl Pts',(4.92169609601798,23.3519615242271,-6.3913110357232));
#449530=CARTESIAN_POINT('Ctrl Pts',(4.92330089590042,23.4730384757729,-6.38935290488262));
#449531=CARTESIAN_POINT('Ctrl Pts',(4.83695933636888,23.4813898257499,-6.30414930262286));
#449532=CARTESIAN_POINT('Ctrl Pts',(4.76527121936352,23.4897411757268,-6.20464951053553));
#449533=CARTESIAN_POINT('Ctrl Pts',(4.71444637045848,23.4980925257038,-6.09544017298549));
#449534=CARTESIAN_POINT('Ctrl Pts',(4.56943523344352,23.5219202159352,-5.78384908020389));
#449535=CARTESIAN_POINT('Ctrl Pts',(4.59426131240048,23.5457479061666,-5.39321753403732));
#449536=CARTESIAN_POINT('Ctrl Pts',(4.77755195197114,23.569575596398,-5.10249121190879));
#449537=CARTESIAN_POINT('Ctrl Pts',(4.9608425915418,23.5934032866293,-4.81176488978025));
#449538=CARTESIAN_POINT('Ctrl Pts',(5.30259779172617,23.6172309768607,-4.62094379168974));
#449539=CARTESIAN_POINT('Ctrl Pts',(5.64626184853499,23.6410586670921,-4.61744171997954));
#449540=CARTESIAN_POINT('Ctrl Pts',(5.98992590534381,23.6648863573235,-4.61393964826935));
#449541=CARTESIAN_POINT('Ctrl Pts',(6.33549881877709,23.6887140475549,-4.79775660293947));
#449542=CARTESIAN_POINT('Ctrl Pts',(6.52467601704459,23.7125417377863,-5.08468731748426));
#449543=CARTESIAN_POINT('Ctrl Pts',(6.71385321531209,23.7363694280177,-5.37161803202905));
#449544=CARTESIAN_POINT('Ctrl Pts',(6.74663469841383,23.7601971182491,-5.76166250644852));
#449545=CARTESIAN_POINT('Ctrl Pts',(6.60800349462427,23.7840248084805,-6.07614404554655));
#449546=CARTESIAN_POINT('Ctrl Pts',(6.46937229083472,23.8078524987119,-6.39062558464459));
#449547=CARTESIAN_POINT('Ctrl Pts',(6.15932840015388,23.8316801889433,-6.6295441884212));
#449548=CARTESIAN_POINT('Ctrl Pts',(5.81990079386588,23.8555078791747,-6.6834528935629));
#449549=CARTESIAN_POINT('Ctrl Pts',(5.49924097144978,23.8780180780408,-6.73438085433327));
#449550=CARTESIAN_POINT('Ctrl Pts',(5.15235699515365,23.9005282769068,-6.62019259508593));
#449551=CARTESIAN_POINT('Ctrl Pts',(4.9216948349357,23.9230384757729,-6.39152331859132));
#449552=CARTESIAN_POINT('Origin',(5.65685387860011,26.,-5.65685387860012));
#449553=CARTESIAN_POINT('',(4.92377157353715,24.3730384757729,-6.39128196913613));
#449554=CARTESIAN_POINT('',(4.92421628016771,24.2519615242271,-6.38942086037359));
#449555=CARTESIAN_POINT('',(4.92305381642377,26.,-6.39065394077646));
#449556=CARTESIAN_POINT('Ctrl Pts',(4.92421628016771,24.2519615242271,-6.38942086037359));
#449557=CARTESIAN_POINT('Ctrl Pts',(5.04895543667044,24.2398389150381,-6.51405309196749));
#449558=CARTESIAN_POINT('Ctrl Pts',(5.20382475542584,24.2277163058492,-6.60860369693141));
#449559=CARTESIAN_POINT('Ctrl Pts',(5.37198243345446,24.2155936966603,-6.65652287894995));
#449560=CARTESIAN_POINT('Ctrl Pts',(5.70250608555364,24.1917660064289,-6.75071080561528));
#449561=CARTESIAN_POINT('Ctrl Pts',(6.08436822205294,24.1679383161975,-6.66474206054895));
#449562=CARTESIAN_POINT('Ctrl Pts',(6.34264042812557,24.1441106259661,-6.4379983333991));
#449563=CARTESIAN_POINT('Ctrl Pts',(6.60091263419821,24.1202829357347,-6.21125460624925));
#449564=CARTESIAN_POINT('Ctrl Pts',(6.73559490984418,24.0964552455033,-5.84373589701587));
#449565=CARTESIAN_POINT('Ctrl Pts',(6.68499023152592,24.0726275552719,-5.5037999963824));
#449566=CARTESIAN_POINT('Ctrl Pts',(6.63438555320766,24.0487998650405,-5.16386409574893));
#449567=CARTESIAN_POINT('Ctrl Pts',(6.39849392092517,24.0249721748091,-4.85151100371537));
#449568=CARTESIAN_POINT('Ctrl Pts',(6.08537566804496,24.0011444845777,-4.70982751913656));
#449569=CARTESIAN_POINT('Ctrl Pts',(5.77225741516475,23.9773167943464,-4.56814403455775));
#449570=CARTESIAN_POINT('Ctrl Pts',(5.38191254168682,23.9534891041149,-4.59713015743369));
#449571=CARTESIAN_POINT('Ctrl Pts',(5.09315534403941,23.9296614138835,-4.78350754767415));
#449572=CARTESIAN_POINT('Ctrl Pts',(4.804398146392,23.9058337236522,-4.96988493791459));
#449573=CARTESIAN_POINT('Ctrl Pts',(4.61722862457511,23.8820060334208,-5.31365359551954));
#449574=CARTESIAN_POINT('Ctrl Pts',(4.6173878516616,23.8581783431894,-5.65733545950024));
#449575=CARTESIAN_POINT('Ctrl Pts',(4.61751307348277,23.8394394035353,-5.92761905169082));
#449576=CARTESIAN_POINT('Ctrl Pts',(4.73349750638545,23.8207004638812,-6.19784896370209));
#449577=CARTESIAN_POINT('Ctrl Pts',(4.92356615355223,23.8019615242271,-6.39146732321148));
#449578=CARTESIAN_POINT('Ctrl Pts',(4.9216948349357,23.9230384757729,-6.39152331859132));
#449579=CARTESIAN_POINT('Ctrl Pts',(4.90819449199352,23.9243559671382,-6.37813961642664));
#449580=CARTESIAN_POINT('Ctrl Pts',(4.895092278726,23.9256734585035,-6.3643637478711));
#449581=CARTESIAN_POINT('Ctrl Pts',(4.88241675495565,23.9269909498688,-6.35020586507153));
#449582=CARTESIAN_POINT('Ctrl Pts',(4.65317164422858,23.9508186401002,-6.0941513249317));
#449583=CARTESIAN_POINT('Ctrl Pts',(4.56349274466962,23.9746463303316,-5.71314343814525));
#449584=CARTESIAN_POINT('Ctrl Pts',(4.6544613426263,23.998474020563,-5.38171929489582));
#449585=CARTESIAN_POINT('Ctrl Pts',(4.74542994058297,24.0223017107944,-5.0502951516464));
#449586=CARTESIAN_POINT('Ctrl Pts',(5.01704603605528,24.0461294010258,-4.76845475193401));
#449587=CARTESIAN_POINT('Ctrl Pts',(5.34488416612327,24.0699570912572,-4.6653072414873));
#449588=CARTESIAN_POINT('Ctrl Pts',(5.67272229619127,24.0937847814886,-4.56215973104059));
#449589=CARTESIAN_POINT('Ctrl Pts',(6.05678246085496,24.11761247172,-4.63770510985959));
#449590=CARTESIAN_POINT('Ctrl Pts',(6.32112934350159,24.1414401619514,-4.8573365604447));
#449591=CARTESIAN_POINT('Ctrl Pts',(6.58547622614821,24.1652678521828,-5.07696801102981));
#449592=CARTESIAN_POINT('Ctrl Pts',(6.73010982677778,24.1890955424141,-5.44068553338104));
#449593=CARTESIAN_POINT('Ctrl Pts',(6.68877448884911,24.2129232326455,-5.78187263496817));
#449594=CARTESIAN_POINT('Ctrl Pts',(6.64743915092045,24.2367509228769,-6.12305973655531));
#449595=CARTESIAN_POINT('Ctrl Pts',(6.42013487443355,24.2605786131083,-6.44171641737836));
#449596=CARTESIAN_POINT('Ctrl Pts',(6.11098818332588,24.2844063033397,-6.59186824658804));
#449597=CARTESIAN_POINT('Ctrl Pts',(5.80184149221821,24.3082339935711,-6.74202007579772));
#449598=CARTESIAN_POINT('Ctrl Pts',(5.41085238648977,24.3320616838025,-6.72366705339403));
#449599=CARTESIAN_POINT('Ctrl Pts',(5.11713028264445,24.3558893740339,-6.54521657215205));
#449600=CARTESIAN_POINT('Ctrl Pts',(5.04666506349635,24.3616057412803,-6.50240552012982));
#449601=CARTESIAN_POINT('Ctrl Pts',(4.98179796021342,24.3673221085266,-6.45038020112141));
#449602=CARTESIAN_POINT('Ctrl Pts',(4.92377157353715,24.3730384757729,-6.39128196913613));
#449603=CARTESIAN_POINT('Origin',(5.65685387860011,26.,-5.65685387860012));
#449604=CARTESIAN_POINT('',(4.92408802232565,24.8230384757729,-6.38933869113556));
#449605=CARTESIAN_POINT('',(4.92212745780798,24.7019615242271,-6.39028821611916));
#449606=CARTESIAN_POINT('',(4.92305381642377,26.,-6.39065394077646));
#449607=CARTESIAN_POINT('Ctrl Pts',(4.92212745780798,24.7019615242271,-6.39028821611916));
#449608=CARTESIAN_POINT('Ctrl Pts',(5.11995795053563,24.6828050564265,-6.5845155347103));
#449609=CARTESIAN_POINT('Ctrl Pts',(5.39828521249021,24.6636485886259,-6.70087353526984));
#449610=CARTESIAN_POINT('Ctrl Pts',(5.67455106061111,24.6444921208254,-6.69616935490973));
#449611=CARTESIAN_POINT('Ctrl Pts',(6.01818314973456,24.620664430594,-6.69031808036474));
#449612=CARTESIAN_POINT('Ctrl Pts',(6.35862591802897,24.5968367403626,-6.49716519325234));
#449613=CARTESIAN_POINT('Ctrl Pts',(6.53992487743045,24.5730090501312,-6.20519269912468));
#449614=CARTESIAN_POINT('Ctrl Pts',(6.72122383683193,24.5491813598998,-5.91322020499702));
#449615=CARTESIAN_POINT('Ctrl Pts',(6.74337898734047,24.5253536696684,-5.52242810385412));
#449616=CARTESIAN_POINT('Ctrl Pts',(6.59624120723028,24.501525979437,-5.21183556708661));
#449617=CARTESIAN_POINT('Ctrl Pts',(6.44910342712008,24.4776982892056,-4.9012430303191));
#449618=CARTESIAN_POINT('Ctrl Pts',(6.13267271639114,24.4538705989742,-4.670850057927));
#449619=CARTESIAN_POINT('Ctrl Pts',(5.7919038045113,24.4300429087428,-4.62619808347199));
#449620=CARTESIAN_POINT('Ctrl Pts',(5.45113489263147,24.4062152185114,-4.58154610901698));
#449621=CARTESIAN_POINT('Ctrl Pts',(5.08602777960075,24.38238752828,-4.72263513249906));
#449622=CARTESIAN_POINT('Ctrl Pts',(4.86383551964991,24.3585598380486,-4.98483324415836));
#449623=CARTESIAN_POINT('Ctrl Pts',(4.64164325969907,24.3347321478172,-5.24703135581765));
#449624=CARTESIAN_POINT('Ctrl Pts',(4.56236585282811,24.3109044575858,-5.63033855565415));
#449625=CARTESIAN_POINT('Ctrl Pts',(4.66231973324216,24.2870767673545,-5.9591644547709));
#449626=CARTESIAN_POINT('Ctrl Pts',(4.71142093690032,24.275371686312,-6.12069642705377));
#449627=CARTESIAN_POINT('Ctrl Pts',(4.80377340246064,24.2636666052695,-6.26908122485669));
#449628=CARTESIAN_POINT('Ctrl Pts',(4.92421628016771,24.2519615242271,-6.38942086037359));
#449629=CARTESIAN_POINT('Ctrl Pts',(4.92377157353715,24.3730384757729,-6.39128196913613));
#449630=CARTESIAN_POINT('Ctrl Pts',(4.7399249826062,24.391149798758,-6.20403942134221));
#449631=CARTESIAN_POINT('Ctrl Pts',(4.62474754709557,24.4092611217431,-5.94579686164739));
#449632=CARTESIAN_POINT('Ctrl Pts',(4.61775970678069,24.4273724447281,-5.68465923264326));
#449633=CARTESIAN_POINT('Ctrl Pts',(4.60856633672445,24.4512001349595,-5.34110031445674));
#449634=CARTESIAN_POINT('Ctrl Pts',(4.78663469857419,24.4750278251909,-4.99253041816396));
#449635=CARTESIAN_POINT('Ctrl Pts',(5.07039290068915,24.4988555154223,-4.79862701145602));
#449636=CARTESIAN_POINT('Ctrl Pts',(5.35415110280411,24.5226832056536,-4.60472360474809));
#449637=CARTESIAN_POINT('Ctrl Pts',(5.7435991451843,24.546510895885,-4.565486687625));
#449638=CARTESIAN_POINT('Ctrl Pts',(6.06033356407531,24.5703385861164,-4.69889042440694));
#449639=CARTESIAN_POINT('Ctrl Pts',(6.37706798296632,24.5941662763478,-4.83229416118888));
#449640=CARTESIAN_POINT('Ctrl Pts',(6.62108877836816,24.6179939665792,-5.13833855187585));
#449641=CARTESIAN_POINT('Ctrl Pts',(6.68061169925027,24.6418216568106,-5.47682676316715));
#449642=CARTESIAN_POINT('Ctrl Pts',(6.74013462013239,24.665649347042,-5.81531497445846));
#449643=CARTESIAN_POINT('Ctrl Pts',(6.61515966649478,24.6894770372734,-6.18624700635411));
#449644=CARTESIAN_POINT('Ctrl Pts',(6.36293701391879,24.7133047275048,-6.41970146010492));
#449645=CARTESIAN_POINT('Ctrl Pts',(6.1107143613428,24.7371324177362,-6.65315591385573));
#449646=CARTESIAN_POINT('Ctrl Pts',(5.73124400982843,24.7609601079676,-6.74913278946171));
#449647=CARTESIAN_POINT('Ctrl Pts',(5.39835869474429,24.784787798199,-6.6636657201663));
#449648=CARTESIAN_POINT('Ctrl Pts',(5.22023136007979,24.797538024057,-6.61793218802978));
#449649=CARTESIAN_POINT('Ctrl Pts',(5.05544287282308,24.8102882499149,-6.5202452116208));
#449650=CARTESIAN_POINT('Ctrl Pts',(4.92408802232565,24.8230384757729,-6.38933869113556));
#449651=CARTESIAN_POINT('Origin',(5.65685387860011,26.,-5.65685387860012));
#449652=CARTESIAN_POINT('',(4.92197603118329,25.2730384757729,-6.39051881327128));
#449653=CARTESIAN_POINT('',(4.92254817630007,25.1519615242271,-6.39198798715976));
#449654=CARTESIAN_POINT('',(4.92305381642377,26.,-6.39065394077646));
#449655=CARTESIAN_POINT('Ctrl Pts',(4.92254817630007,25.1519615242271,-6.39198798715976));
#449656=CARTESIAN_POINT('Ctrl Pts',(4.94650751599249,25.1495988880462,-6.41627314991444));
#449657=CARTESIAN_POINT('Ctrl Pts',(4.97169983154625,25.1472362518654,-6.43929566708609));
#449658=CARTESIAN_POINT('Ctrl Pts',(4.99805942366946,25.1448736156846,-6.46089355482011));
#449659=CARTESIAN_POINT('Ctrl Pts',(5.26390153716753,25.1210459254532,-6.67871286308055));
#449660=CARTESIAN_POINT('Ctrl Pts',(5.64846913729549,25.0972182352218,-6.75163093056004));
#449661=CARTESIAN_POINT('Ctrl Pts',(5.97559449046916,25.0733905449904,-6.64624470558553));
#449662=CARTESIAN_POINT('Ctrl Pts',(6.30271984364283,25.049562854759,-6.54085848061101));
#449663=CARTESIAN_POINT('Ctrl Pts',(6.57240294986222,25.0257351645276,-6.25716796318249));
#449664=CARTESIAN_POINT('Ctrl Pts',(6.66110381706144,25.0019074742962,-5.92512971718013));
#449665=CARTESIAN_POINT('Ctrl Pts',(6.74980468426065,24.9780797840648,-5.59309147117778));
#449666=CARTESIAN_POINT('Ctrl Pts',(6.65752331243968,24.9542520938335,-5.21270549660159));
#449667=CARTESIAN_POINT('Ctrl Pts',(6.42653317184816,24.9304244036021,-4.95822404429259));
#449668=CARTESIAN_POINT('Ctrl Pts',(6.19554303125664,24.9065967133707,-4.70374259198359));
#449669=CARTESIAN_POINT('Ctrl Pts',(5.82584412189456,24.8827690231393,-4.57516566194178));
#449670=CARTESIAN_POINT('Ctrl Pts',(5.48679296352304,24.8589413329079,-4.63139343216518));
#449671=CARTESIAN_POINT('Ctrl Pts',(5.14774180515151,24.8351136426765,-4.68762120238858));
#449672=CARTESIAN_POINT('Ctrl Pts',(4.83933839777055,24.8112859524451,-4.9286536728772));
#449673=CARTESIAN_POINT('Ctrl Pts',(4.70286022094558,24.7874582622137,-5.24407554312886));
#449674=CARTESIAN_POINT('Ctrl Pts',(4.56638204412062,24.7636305719823,-5.55949741338051));
#449675=CARTESIAN_POINT('Ctrl Pts',(4.60182909785165,24.7398028817509,-5.94930868339519));
#449676=CARTESIAN_POINT('Ctrl Pts',(4.79296332969341,24.7159751915195,-6.23493948741374));
#449677=CARTESIAN_POINT('Ctrl Pts',(4.83043362171106,24.7113039690887,-6.29093505415592));
#449678=CARTESIAN_POINT('Ctrl Pts',(4.87388734148021,24.7066327466579,-6.34292671833547));
#449679=CARTESIAN_POINT('Ctrl Pts',(4.92212745780798,24.7019615242271,-6.39028821611916));
#449680=CARTESIAN_POINT('Ctrl Pts',(4.92408802232565,24.8230384757729,-6.38933869113556));
#449681=CARTESIAN_POINT('Ctrl Pts',(4.80996622614209,24.8341159401463,-6.27560640646284));
#449682=CARTESIAN_POINT('Ctrl Pts',(4.72108089883846,24.8451934045197,-6.13679925493306));
#449683=CARTESIAN_POINT('Ctrl Pts',(4.67061008310121,24.8562708688931,-5.98520281626299));
#449684=CARTESIAN_POINT('Ctrl Pts',(4.56204706519615,24.8800985591245,-5.65911799585187));
#449685=CARTESIAN_POINT('Ctrl Pts',(4.63122130803993,24.9039262493559,-5.27385936922642));
#449686=CARTESIAN_POINT('Ctrl Pts',(4.84644449237099,24.9277539395873,-5.00591117956891));
#449687=CARTESIAN_POINT('Ctrl Pts',(5.06166767670205,24.9515816298187,-4.7379629899114));
#449688=CARTESIAN_POINT('Ctrl Pts',(5.42293980252039,24.9754093200501,-4.58732523722183));
#449689=CARTESIAN_POINT('Ctrl Pts',(5.76476474386039,24.9992370102815,-4.62300419682159));
#449690=CARTESIAN_POINT('Ctrl Pts',(6.10658968520039,25.0230647005129,-4.65868315642135));
#449691=CARTESIAN_POINT('Ctrl Pts',(6.42896744206204,25.0468923907443,-4.88067882831045));
#449692=CARTESIAN_POINT('Ctrl Pts',(6.58421869570625,25.0707200809757,-5.18729621377842));
#449693=CARTESIAN_POINT('Ctrl Pts',(6.73946994935045,25.0945477712071,-5.4939135992464));
#449694=CARTESIAN_POINT('Ctrl Pts',(6.72759469977719,25.1183754614385,-5.88515269829325));
#449695=CARTESIAN_POINT('Ctrl Pts',(6.5540334824637,25.1422031516699,-6.18179018209155));
#449696=CARTESIAN_POINT('Ctrl Pts',(6.38047226515022,25.1660308419013,-6.47842766588984));
#449697=CARTESIAN_POINT('Ctrl Pts',(6.0452250800965,25.1898585321326,-6.68046353443956));
#449698=CARTESIAN_POINT('Ctrl Pts',(5.70186524531576,25.213686222364,-6.69534535485933));
#449699=CARTESIAN_POINT('Ctrl Pts',(5.41677424787487,25.2334703068337,-6.70770170116849));
#449700=CARTESIAN_POINT('Ctrl Pts',(5.12609043162756,25.2532543913033,-6.59103501365993));
#449701=CARTESIAN_POINT('Ctrl Pts',(4.92197603118329,25.2730384757729,-6.39051881327128));
#449702=CARTESIAN_POINT('Origin',(5.65685387860011,26.,-5.65685387860012));
#449703=CARTESIAN_POINT('',(4.92276701974739,25.7230384757729,-6.39190058798136));
#449704=CARTESIAN_POINT('',(4.92443355077908,25.6019615242271,-6.39006796800885));
#449705=CARTESIAN_POINT('',(4.92305381642377,26.,-6.39065394077646));
#449706=CARTESIAN_POINT('',(6.69274404704181,26.,-5.59475217632209));
#449707=CARTESIAN_POINT('Ctrl Pts',(4.92276701974739,25.7230384757729,-6.39190058798136));
#449708=CARTESIAN_POINT('Ctrl Pts',(4.71160994855805,25.7438759131544,-6.17742942344334));
#449709=CARTESIAN_POINT('Ctrl Pts',(4.59523934827088,25.764713350536,-5.86562000134797));
#449710=CARTESIAN_POINT('Ctrl Pts',(4.62142687258513,25.7855507879175,-5.56615422141077));
#449711=CARTESIAN_POINT('Ctrl Pts',(4.65137240791476,25.8093784781489,-5.22371394391399));
#449712=CARTESIAN_POINT('Ctrl Pts',(4.86772710302321,25.8332061683802,-4.8974142264151));
#449713=CARTESIAN_POINT('Ctrl Pts',(5.17187737628347,25.8570338586116,-4.7372531902219));
#449714=CARTESIAN_POINT('Ctrl Pts',(5.47602764954372,25.880861548843,-4.57709215402869));
#449715=CARTESIAN_POINT('Ctrl Pts',(5.86797350095578,25.9046892390744,-4.58306979914119));
#449716=CARTESIAN_POINT('Ctrl Pts',(6.16698733288025,25.9285169293058,-4.75132533448083));
#449717=CARTESIAN_POINT('Ctrl Pts',(6.46600116480472,25.9523446195372,-4.91958086982048));
#449718=CARTESIAN_POINT('Ctrl Pts',(6.67208297724159,25.9761723097686,-5.25011429538726));
#449719=CARTESIAN_POINT('Ctrl Pts',(6.69274404704181,26.,-5.59475217632212));
#449720=CARTESIAN_POINT('',(5.59444809180803,26.,-6.69457727933146));
#449721=CARTESIAN_POINT('Origin',(5.65685387860011,26.,-5.65685387860012));
#449722=CARTESIAN_POINT('Ctrl Pts',(5.59444726164187,26.,-6.69458228414866));
#449723=CARTESIAN_POINT('Ctrl Pts',(5.92484673178863,25.9770624644402,-6.71351646533255));
#449724=CARTESIAN_POINT('Ctrl Pts',(6.26627937525033,25.9541249288804,-6.56158375468957));
#449725=CARTESIAN_POINT('Ctrl Pts',(6.47167795527827,25.9311873933205,-6.30214239804398));
#449726=CARTESIAN_POINT('Ctrl Pts',(6.68504759676004,25.9073597030892,-6.03263270014108));
#449727=CARTESIAN_POINT('Ctrl Pts',(6.75161994353754,25.8835320128578,-5.64710810132191));
#449728=CARTESIAN_POINT('Ctrl Pts',(6.64083855948586,25.8597043226264,-5.32182159136528));
#449729=CARTESIAN_POINT('Ctrl Pts',(6.53005717543418,25.835876632395,-4.99653508140864));
#449730=CARTESIAN_POINT('Ctrl Pts',(6.24192206055332,25.8120489421636,-4.73148666031454));
#449731=CARTESIAN_POINT('Ctrl Pts',(5.90845611919746,25.7882212519322,-4.64827248224482));
#449732=CARTESIAN_POINT('Ctrl Pts',(5.5749901778416,25.7643935617008,-4.56505830417509));
#449733=CARTESIAN_POINT('Ctrl Pts',(5.19619341001074,25.7405658714694,-4.66367836912974));
#449734=CARTESIAN_POINT('Ctrl Pts',(4.94557465216384,25.716738181238,-4.89886414913017));
#449735=CARTESIAN_POINT('Ctrl Pts',(4.69495589431694,25.6929104910066,-5.13404992913059));
#449736=CARTESIAN_POINT('Ctrl Pts',(4.572515146454,25.6690828007752,-5.50580142417678));
#449737=CARTESIAN_POINT('Ctrl Pts',(4.63434949773116,25.6452551105439,-5.84386841174159));
#449738=CARTESIAN_POINT('Ctrl Pts',(4.67179935541582,25.6308239151049,-6.04861804217652));
#449739=CARTESIAN_POINT('Ctrl Pts',(4.7768430935332,25.616392719666,-6.24101187097706));
#449740=CARTESIAN_POINT('Ctrl Pts',(4.92443355077908,25.6019615242271,-6.39006796800885));
#449741=CARTESIAN_POINT('Origin',(5.65685387860011,26.993675081176,-5.65685387860012));
#449742=CARTESIAN_POINT('',(4.74524035180399,22.756324918824,-6.5673434103921));
#449743=CARTESIAN_POINT('',(4.74364038176038,22.718675081176,-6.57057146528766));
#449744=CARTESIAN_POINT('',(4.74468613086949,26.993675081176,-6.56902162633079));
#449745=CARTESIAN_POINT('',(6.64591806159944,22.5,-4.8286920333622));
#449746=CARTESIAN_POINT('Ctrl Pts',(4.74364038176038,22.718675081176,-6.57057146528766));
#449747=CARTESIAN_POINT('Ctrl Pts',(4.76142457130848,22.7172664581449,-6.58852418981576));
#449748=CARTESIAN_POINT('Ctrl Pts',(5.09000197050781,22.6920301448823,-6.9000556810006));
#449749=CARTESIAN_POINT('Ctrl Pts',(6.06611679986992,22.6429661413884,-7.12689194633153));
#449750=CARTESIAN_POINT('Ctrl Pts',(7.11331947438321,22.5714830706942,-6.10694434613243));
#449751=CARTESIAN_POINT('Ctrl Pts',(6.92144528650133,22.5238276902314,-5.15775103452081));
#449752=CARTESIAN_POINT('Ctrl Pts',(6.64591806159944,22.5,-4.8286920333622));
#449753=CARTESIAN_POINT('',(6.09734856608926,22.5,-4.44194770692244));
#449754=CARTESIAN_POINT('Origin',(5.65685387860011,22.5,-5.65685387860012));
#449755=CARTESIAN_POINT('Ctrl Pts',(4.74524035180399,22.756324918824,-6.5673434103921));
#449756=CARTESIAN_POINT('Ctrl Pts',(4.93595953019022,22.7414761952386,-6.75594870135602));
#449757=CARTESIAN_POINT('Ctrl Pts',(5.58182921801751,22.7027997814218,-7.1012121014615));
#449758=CARTESIAN_POINT('Ctrl Pts',(6.78713386963136,22.6402956773736,-6.68055232418451));
#449759=CARTESIAN_POINT('Ctrl Pts',(7.12528591239125,22.5697027613511,-5.27997950888059));
#449760=CARTESIAN_POINT('Ctrl Pts',(6.48370144903282,22.5229375355598,-4.58325719964658));
#449761=CARTESIAN_POINT('Ctrl Pts',(6.09735008669021,22.5,-4.44194158662797));
#449762=CARTESIAN_POINT('Origin',(5.65685387860011,26.993675081176,-5.65685387860012));
#449763=CARTESIAN_POINT('',(4.74299838399068,23.206324918824,-6.56983844394705));
#449764=CARTESIAN_POINT('',(4.74631652959707,23.168675081176,-6.56867439792569));
#449765=CARTESIAN_POINT('',(4.74468613086949,26.993675081176,-6.56902162633079));
#449766=CARTESIAN_POINT('Ctrl Pts',(4.74631652959707,23.168675081176,-6.56867439792569));
#449767=CARTESIAN_POINT('Ctrl Pts',(4.853408844765,23.1602325995332,-6.67716702479821));
#449768=CARTESIAN_POINT('Ctrl Pts',(5.33214451040115,23.127962427659,-7.02077633180239));
#449769=CARTESIAN_POINT('Ctrl Pts',(6.47507582842176,23.0718645655535,-6.94377741359719));
#449770=CARTESIAN_POINT('Ctrl Pts',(7.18181942856023,23.0003814948592,-5.66653874837813));
#449771=CARTESIAN_POINT('Ctrl Pts',(6.49141154940691,22.9288984241651,-4.38054591235379));
#449772=CARTESIAN_POINT('Ctrl Pts',(5.03639155729104,22.8574153534709,-4.26365553420012));
#449773=CARTESIAN_POINT('Ctrl Pts',(4.16730445086878,22.7873409058079,-5.40079341912851));
#449774=CARTESIAN_POINT('Ctrl Pts',(4.46059450521194,22.7410941483762,-6.28484325502835));
#449775=CARTESIAN_POINT('Ctrl Pts',(4.74364038176038,22.718675081176,-6.57057146528766));
#449776=CARTESIAN_POINT('Ctrl Pts',(4.74299838399068,23.206324918824,-6.56983844394705));
#449777=CARTESIAN_POINT('Ctrl Pts',(5.02227299078827,23.184442336627,-6.84584090104065));
#449778=CARTESIAN_POINT('Ctrl Pts',(5.8884730690954,23.1387320641985,-7.14533371342118));
#449779=CARTESIAN_POINT('Ctrl Pts',(7.03563221165043,23.0691941015387,-6.3084575374563));
#449780=CARTESIAN_POINT('Ctrl Pts',(6.95165327175697,22.9977110308445,-4.85119529970874));
#449781=CARTESIAN_POINT('Ctrl Pts',(5.68141376558385,22.9262279601503,-4.13204038713624));
#449782=CARTESIAN_POINT('Ctrl Pts',(4.38863987327371,22.8547448894562,-4.80994952176022));
#449783=CARTESIAN_POINT('Ctrl Pts',(4.28501879514302,22.7981105423474,-5.9617065202947));
#449784=CARTESIAN_POINT('Ctrl Pts',(4.62991319040622,22.76530388547,-6.45329450867432));
#449785=CARTESIAN_POINT('Ctrl Pts',(4.74524035180399,22.756324918824,-6.5673434103921));
#449786=CARTESIAN_POINT('Origin',(5.65685387860011,26.993675081176,-5.65685387860012));
#449787=CARTESIAN_POINT('',(4.74532300381163,23.656324918824,-6.57003272085371));
#449788=CARTESIAN_POINT('',(4.74499326893249,23.618675081176,-6.56740434249263));
#449789=CARTESIAN_POINT('',(4.74468613086949,26.993675081176,-6.56902162633079));
#449790=CARTESIAN_POINT('Ctrl Pts',(4.74499326893249,23.618675081176,-6.56740434249264));
#449791=CARTESIAN_POINT('Ctrl Pts',(4.94389036502613,23.6031987409216,-6.76368003125862));
#449792=CARTESIAN_POINT('Ctrl Pts',(5.60787864620878,23.5638947104357,-7.10715379447204));
#449793=CARTESIAN_POINT('Ctrl Pts',(6.81352117024561,23.5007629897185,-6.65070324968042));
#449794=CARTESIAN_POINT('Ctrl Pts',(7.11892889768229,23.4292799190243,-5.22331918686542));
#449795=CARTESIAN_POINT('Ctrl Pts',(6.08480364614364,23.3577968483302,-4.19313572939824));
#449796=CARTESIAN_POINT('Ctrl Pts',(4.65859667867589,23.2863137776359,-4.50398657889369));
#449797=CARTESIAN_POINT('Ctrl Pts',(4.20740365817457,23.2232731885846,-5.70962577012502));
#449798=CARTESIAN_POINT('Ctrl Pts',(4.55115618731809,23.1840602897646,-6.37096218895919));
#449799=CARTESIAN_POINT('Ctrl Pts',(4.74631652959707,23.168675081176,-6.56867439792569));
#449800=CARTESIAN_POINT('Ctrl Pts',(4.74532300381163,23.656324918824,-6.57003272085371));
#449801=CARTESIAN_POINT('Ctrl Pts',(4.80948437015677,23.6512361682467,-6.63539236159828));
#449802=CARTESIAN_POINT('Ctrl Pts',(5.21266771861286,23.622319727438,-6.9668858368575));
#449803=CARTESIAN_POINT('Ctrl Pts',(6.28682364983267,23.569575596398,-7.04564953674368));
#449804=CARTESIAN_POINT('Ctrl Pts',(7.16543624640093,23.4980925257038,-5.88000083782647));
#449805=CARTESIAN_POINT('Ctrl Pts',(6.66190630419616,23.4266094550096,-4.50990820099157));
#449806=CARTESIAN_POINT('Ctrl Pts',(5.23756146736659,23.3551263843154,-4.19063094092434));
#449807=CARTESIAN_POINT('Ctrl Pts',(4.19736598356861,23.2836433136212,-5.21468783779197));
#449808=CARTESIAN_POINT('Ctrl Pts',(4.40342562281452,23.2340428251241,-6.20635078283889));
#449809=CARTESIAN_POINT('Ctrl Pts',(4.71817410701172,23.2082700268584,-6.54530502316694));
#449810=CARTESIAN_POINT('Ctrl Pts',(4.74299838399068,23.206324918824,-6.56983844394705));
#449811=CARTESIAN_POINT('Origin',(5.65685387860011,26.993675081176,-5.65685387860012));
#449812=CARTESIAN_POINT('',(4.74613115927677,24.106324918824,-6.56748881619374));
#449813=CARTESIAN_POINT('',(4.74299681637215,24.068675081176,-6.57010232725217));
#449814=CARTESIAN_POINT('',(4.74468613086949,26.993675081176,-6.56902162633079));
#449815=CARTESIAN_POINT('Ctrl Pts',(4.74299681637215,24.068675081176,-6.57010232725218));
#449816=CARTESIAN_POINT('Ctrl Pts',(5.02972694085412,24.0461648823099,-6.85435514987614));
#449817=CARTESIAN_POINT('Ctrl Pts',(5.91736950865738,23.9998269932124,-7.14655186859909));
#449818=CARTESIAN_POINT('Ctrl Pts',(7.0522818436793,23.9296614138836,-6.27199288310558));
#449819=CARTESIAN_POINT('Ctrl Pts',(6.93003241982605,23.8581783431894,-4.81743049717126));
#449820=CARTESIAN_POINT('Ctrl Pts',(5.64131435190337,23.7866952724952,-4.13193628895796));
#449821=CARTESIAN_POINT('Ctrl Pts',(4.3668333837381,23.715212201801,-4.84355050202496));
#449822=CARTESIAN_POINT('Ctrl Pts',(4.29429575151248,23.6592054713613,-5.98491025846012));
#449823=CARTESIAN_POINT('Ctrl Pts',(4.63766432477859,23.627026431153,-6.4614899633887));
#449824=CARTESIAN_POINT('Ctrl Pts',(4.74499326893249,23.618675081176,-6.56740434249264));
#449825=CARTESIAN_POINT('Ctrl Pts',(4.74613115927677,24.106324918824,-6.56748881619374));
#449826=CARTESIAN_POINT('Ctrl Pts',(4.90119115627847,24.0942023096351,-6.72241589762581));
#449827=CARTESIAN_POINT('Ctrl Pts',(5.47210261995127,24.0582520102147,-7.07096798466868));
#449828=CARTESIAN_POINT('Ctrl Pts',(6.662968703113,23.998474020563,-6.80286792203874));
#449829=CARTESIAN_POINT('Ctrl Pts',(7.16522879152533,23.9269909498688,-5.43230911237055));
#449830=CARTESIAN_POINT('Ctrl Pts',(6.2855365564656,23.8555078791747,-4.26747512907024));
#449831=CARTESIAN_POINT('Ctrl Pts',(4.82985391579145,23.7840248084805,-4.37557081254884));
#449832=CARTESIAN_POINT('Ctrl Pts',(4.18154636230721,23.7176304883636,-5.56629788826614));
#449833=CARTESIAN_POINT('Ctrl Pts',(4.50905361827065,23.6750638584781,-6.32935078034096));
#449834=CARTESIAN_POINT('Ctrl Pts',(4.74532300381163,23.656324918824,-6.57003272085371));
#449835=CARTESIAN_POINT('Origin',(5.65685387860011,26.993675081176,-5.65685387860012));
#449836=CARTESIAN_POINT('',(4.74353459859835,24.556324918824,-6.56856700353347));
#449837=CARTESIAN_POINT('',(4.74557835604531,24.518675081176,-6.56980231202958));
#449838=CARTESIAN_POINT('',(4.74468613086949,26.993675081176,-6.56902162633079));
#449839=CARTESIAN_POINT('Ctrl Pts',(4.74557835604531,24.518675081176,-6.56980231202958));
#449840=CARTESIAN_POINT('Ctrl Pts',(4.81770944620421,24.5129587139297,-6.64326578517921));
#449841=CARTESIAN_POINT('Ctrl Pts',(5.23445549419879,24.4834146564519,-6.97750833641272));
#449842=CARTESIAN_POINT('Ctrl Pts',(6.32311258055821,24.4300429087428,-7.02860988272989));
#449843=CARTESIAN_POINT('Ctrl Pts',(7.17078066054311,24.3585598380486,-5.84026841822957));
#449844=CARTESIAN_POINT('Ctrl Pts',(6.63140987332417,24.2870767673545,-4.4838850778304));
#449845=CARTESIAN_POINT('Ctrl Pts',(5.19916430623342,24.2155936966603,-4.2021595986403));
#449846=CARTESIAN_POINT('Ctrl Pts',(4.18624762160045,24.1441106259661,-5.25320498229437));
#449847=CARTESIAN_POINT('Ctrl Pts',(4.41536649518845,24.095137754138,-6.22663461042285));
#449848=CARTESIAN_POINT('Ctrl Pts',(4.72621489163553,24.0699925725413,-6.55346539562853));
#449849=CARTESIAN_POINT('Ctrl Pts',(4.74299681637215,24.068675081176,-6.57010232725218));
#449850=CARTESIAN_POINT('Ctrl Pts',(4.74353459859835,24.556324918824,-6.56856700353346));
#449851=CARTESIAN_POINT('Ctrl Pts',(4.98945253222269,24.5371684510234,-6.81000592522228));
#449852=CARTESIAN_POINT('Ctrl Pts',(5.76578134653658,24.4941842929915,-7.13455935910424));
#449853=CARTESIAN_POINT('Ctrl Pts',(6.95240396480877,24.4273724447281,-6.46131966662841));
#449854=CARTESIAN_POINT('Ctrl Pts',(7.03502543671246,24.3558893740339,-5.00396921476326));
#449855=CARTESIAN_POINT('Ctrl Pts',(5.85498510857852,24.2844063033397,-4.14478270244581));
#449856=CARTESIAN_POINT('Ctrl Pts',(4.49341967622111,24.2129232326456,-4.67093497503137));
#449857=CARTESIAN_POINT('Ctrl Pts',(4.24791389261248,24.1535627711403,-5.85795834238072));
#449858=CARTESIAN_POINT('Ctrl Pts',(4.5964117545626,24.1180299998665,-6.41789774915756));
#449859=CARTESIAN_POINT('Ctrl Pts',(4.74613115927677,24.106324918824,-6.56748881619374));
#449860=CARTESIAN_POINT('Origin',(5.65685387860011,26.993675081176,-5.65685387860012));
#449861=CARTESIAN_POINT('',(4.74405758279953,25.006324918824,-6.57067994464874));
#449862=CARTESIAN_POINT('',(4.74597172529335,24.968675081176,-6.56738667375376));
#449863=CARTESIAN_POINT('',(4.74468613086949,26.993675081176,-6.56902162633079));
#449864=CARTESIAN_POINT('Ctrl Pts',(4.74597172529335,24.968675081176,-6.56738667375376));
#449865=CARTESIAN_POINT('Ctrl Pts',(4.90925551921452,24.955924855318,-6.73011316031215));
#449866=CARTESIAN_POINT('Ctrl Pts',(5.49691387622178,24.9193469392286,-7.0784783223036));
#449867=CARTESIAN_POINT('Ctrl Pts',(6.69274573713214,24.8589413329079,-6.77602463836695));
#449868=CARTESIAN_POINT('Ctrl Pts',(7.15880506797054,24.7874582622137,-5.39273679116275));
#449869=CARTESIAN_POINT('Ctrl Pts',(6.24879737998679,24.7159751915195,-4.25142935492228));
#449870=CARTESIAN_POINT('Ctrl Pts',(4.79645922145989,24.6444921208253,-4.39775252453571));
#449871=CARTESIAN_POINT('Ctrl Pts',(4.18550614000559,24.5787254173775,-5.59369688000734));
#449872=CARTESIAN_POINT('Ctrl Pts',(4.51704344657683,24.5367864041611,-6.33704597702196));
#449873=CARTESIAN_POINT('Ctrl Pts',(4.74557835604531,24.518675081176,-6.56980231202958));
#449874=CARTESIAN_POINT('Ctrl Pts',(4.74405758279953,25.006324918824,-6.57067994464874));
#449875=CARTESIAN_POINT('Ctrl Pts',(4.77384081402403,25.0039622826432,-6.60086819803687));
#449876=CARTESIAN_POINT('Ctrl Pts',(5.12098437694123,24.9777719562309,-6.91811250300101));
#449877=CARTESIAN_POINT('Ctrl Pts',(6.12447699388038,24.9277539395874,-7.10838527255516));
#449878=CARTESIAN_POINT('Ctrl Pts',(7.13018513270865,24.8562708688931,-6.05044038944422));
#449879=CARTESIAN_POINT('Ctrl Pts',(6.78604742232836,24.784787798199,-4.63189669239788));
#449880=CARTESIAN_POINT('Ctrl Pts',(5.40735816264999,24.7133047275048,-4.15240479236239));
#449881=CARTESIAN_POINT('Ctrl Pts',(4.25725342975252,24.6418216568106,-5.0512683537124));
#449882=CARTESIAN_POINT('Ctrl Pts',(4.35401829743014,24.589495053917,-6.11539165852711));
#449883=CARTESIAN_POINT('Ctrl Pts',(4.68356856625642,24.5609961412548,-6.50969315902277));
#449884=CARTESIAN_POINT('Ctrl Pts',(4.74353459859835,24.556324918824,-6.56856700353346));
#449885=CARTESIAN_POINT('Origin',(5.65685387860011,26.993675081176,-5.65685387860012));
#449886=CARTESIAN_POINT('',(4.74640124271564,25.456324918824,-6.56829321884323));
#449887=CARTESIAN_POINT('',(4.74334636410459,25.418675081176,-6.56885365284802));
#449888=CARTESIAN_POINT('',(4.74468613086949,26.993675081176,-6.56902162633079));
#449889=CARTESIAN_POINT('Ctrl Pts',(4.74334636410459,25.418675081176,-6.56885365284802));
#449890=CARTESIAN_POINT('Ctrl Pts',(4.99707565976646,25.3988909967064,-6.81811011972481));
#449891=CARTESIAN_POINT('Ctrl Pts',(5.79361205385018,25.3552792220053,-7.13780202337966));
#449892=CARTESIAN_POINT('Ctrl Pts',(6.97310209577086,25.287839757073,-6.42698533143036));
#449893=CARTESIAN_POINT('Ctrl Pts',(7.01738753624157,25.2163566863788,-4.96796792520408));
#449894=CARTESIAN_POINT('Ctrl Pts',(5.81516935358236,25.1448736156846,-4.14009680960707));
#449895=CARTESIAN_POINT('Ctrl Pts',(4.46790543942481,25.0733905449904,-4.70185841202445));
#449896=CARTESIAN_POINT('Ctrl Pts',(4.25595199715398,25.0146577001542,-5.88231068328694));
#449897=CARTESIAN_POINT('Ctrl Pts',(4.604109892408,24.9797525455494,-6.4260090324839));
#449898=CARTESIAN_POINT('Ctrl Pts',(4.74597172529335,24.968675081176,-6.56738667375376));
#449899=CARTESIAN_POINT('Ctrl Pts',(4.74640124271564,25.456324918824,-6.56829321884323));
#449900=CARTESIAN_POINT('Ctrl Pts',(4.86586022639608,25.4469284240315,-6.68893848409318));
#449901=CARTESIAN_POINT('Ctrl Pts',(5.36752678600608,25.4137042390077,-7.03476003379299));
#449902=CARTESIAN_POINT('Ctrl Pts',(6.5258341885166,25.3566523637524,-6.9100356033464));
#449903=CARTESIAN_POINT('Ctrl Pts',(7.18099123031483,25.2851692930582,-5.60564496305001));
#449904=CARTESIAN_POINT('Ctrl Pts',(6.43975200870338,25.213686222364,-4.34815567114858));
#449905=CARTESIAN_POINT('Ctrl Pts',(4.98123363545819,25.1422031516699,-4.2896855842815));
#449906=CARTESIAN_POINT('Ctrl Pts',(4.16945626611646,25.0730827171565,-5.44432497425889));
#449907=CARTESIAN_POINT('Ctrl Pts',(4.47347056935133,25.0277899728745,-6.29641321838457));
#449908=CARTESIAN_POINT('Ctrl Pts',(4.74405758279953,25.006324918824,-6.57067994464874));
#449909=CARTESIAN_POINT('Origin',(5.65685387860011,26.993675081176,-5.65685387860012));
#449910=CARTESIAN_POINT('',(4.74450601134849,25.906324918824,-6.56704169373441));
#449911=CARTESIAN_POINT('',(4.74432962138981,25.868675081176,-6.57057130100612));
#449912=CARTESIAN_POINT('',(4.74468613086949,26.993675081176,-6.56902162633079));
#449913=CARTESIAN_POINT('',(4.53900700771687,26.,-5.01302286563433));
#449914=CARTESIAN_POINT('Ctrl Pts',(4.53900700771688,26.,-5.01302286563431));
#449915=CARTESIAN_POINT('Ctrl Pts',(4.32480615636363,25.9761723097686,-5.38492752167559));
#449916=CARTESIAN_POINT('Ctrl Pts',(4.30899334914827,25.9449472827099,-6.01924597306242));
#449917=CARTESIAN_POINT('Ctrl Pts',(4.64940368207851,25.9137222556513,-6.47338425157137));
#449918=CARTESIAN_POINT('Ctrl Pts',(4.74450601134849,25.906324918824,-6.56704169373441));
#449919=CARTESIAN_POINT('',(5.01208503488091,26.,-4.53689596693371));
#449920=CARTESIAN_POINT('Origin',(5.65685387860011,26.,-5.65685387860012));
#449921=CARTESIAN_POINT('Ctrl Pts',(5.01208247494518,26.,-4.5368902045627));
#449922=CARTESIAN_POINT('Ctrl Pts',(4.65613984562121,25.9770624644402,-4.74314812622022));
#449923=CARTESIAN_POINT('Ctrl Pts',(4.17795197796789,25.9332874914989,-5.48969900651177));
#449924=CARTESIAN_POINT('Ctrl Pts',(4.48184576512937,25.8895125185575,-6.3039677816093));
#449925=CARTESIAN_POINT('Ctrl Pts',(4.74432962138981,25.868675081176,-6.57057130100612));
#449926=CARTESIAN_POINT('Origin',(-5.65685387860012,26.,-5.65685387860011));
#449927=CARTESIAN_POINT('',(-6.39190072013885,22.573038475773,-4.9222125558517));
#449928=CARTESIAN_POINT('',(-6.39065394077646,22.5,-4.92305381642377));
#449929=CARTESIAN_POINT('',(-6.39065394077646,26.,-4.92305381642377));
#449930=CARTESIAN_POINT('',(-6.66622270032004,22.5,-5.8978925564917));
#449931=CARTESIAN_POINT('Origin',(-5.65685387860012,22.5,-5.65685387860011));
#449932=CARTESIAN_POINT('Ctrl Pts',(-6.66798006829997,22.5,-5.89851203167784));
#449933=CARTESIAN_POINT('Ctrl Pts',(-6.7439998684947,22.5229375355598,-5.5764199513446));
#449934=CARTESIAN_POINT('Ctrl Pts',(-6.65366449057419,22.5458750711197,
-5.21379162224851));
#449935=CARTESIAN_POINT('Ctrl Pts',(-6.43383171727969,22.5688126066795,
-4.96646199655034));
#449936=CARTESIAN_POINT('Ctrl Pts',(-6.42033150900063,22.5702212297106,
-4.95127317183385));
#449937=CARTESIAN_POINT('Ctrl Pts',(-6.40634292159547,22.5716298527418,
-4.93651917810251));
#449938=CARTESIAN_POINT('Ctrl Pts',(-6.39190072013885,22.573038475773,-4.9222125558517));
#449939=CARTESIAN_POINT('Origin',(-5.65685387860012,26.,-5.65685387860011));
#449940=CARTESIAN_POINT('',(-6.39037461032892,23.0230384757729,-4.92436540268704));
#449941=CARTESIAN_POINT('',(-6.38930388760559,22.9019615242271,-4.92349966353597));
#449942=CARTESIAN_POINT('',(-6.39065394077646,26.,-4.92305381642377));
#449943=CARTESIAN_POINT('',(-5.77557608073439,22.5,-4.62591736201901));
#449944=CARTESIAN_POINT('Ctrl Pts',(-6.38930388760559,22.9019615242271,
-4.92349966353597));
#449945=CARTESIAN_POINT('Ctrl Pts',(-6.54102880287524,22.8871128006417,
-5.07692511110986));
#449946=CARTESIAN_POINT('Ctrl Pts',(-6.64766299899898,22.8722640770563,
-5.27640120658105));
#449947=CARTESIAN_POINT('Ctrl Pts',(-6.68249361011691,22.8574153534709,
-5.48772889025785));
#449948=CARTESIAN_POINT('Ctrl Pts',(-6.73838615923167,22.8335876632395,
-5.82684562005693));
#449949=CARTESIAN_POINT('Ctrl Pts',(-6.60938089562333,22.8097599730081,
-6.19648078060475));
#449950=CARTESIAN_POINT('Ctrl Pts',(-6.35472685290066,22.7859322827767,
-6.42720821100081));
#449951=CARTESIAN_POINT('Ctrl Pts',(-6.10007281017799,22.7621045925453,
-6.65793564139688));
#449952=CARTESIAN_POINT('Ctrl Pts',(-5.71976998834099,22.7382769023139,
-6.74975534164119));
#449953=CARTESIAN_POINT('Ctrl Pts',(-5.38773213421059,22.7144492120825,
-6.66080060824128));
#449954=CARTESIAN_POINT('Ctrl Pts',(-5.05569428008018,22.6906215218511,
-6.57184587484137));
#449955=CARTESIAN_POINT('Ctrl Pts',(-4.77192139365638,22.6667938316197,
-6.30211670779724));
#449956=CARTESIAN_POINT('Ctrl Pts',(-4.66700870222797,22.6429661413884,
-5.97477550103877));
#449957=CARTESIAN_POINT('Ctrl Pts',(-4.56209601079956,22.619138451157,-5.6474342942803));
#449958=CARTESIAN_POINT('Ctrl Pts',(-4.63604351436656,22.5953107609256,
-5.26248104780748));
#449959=CARTESIAN_POINT('Ctrl Pts',(-4.85366607828882,22.5714830706942,
-4.99722717517853));
#449960=CARTESIAN_POINT('Ctrl Pts',(-5.07128864221107,22.5476553804628,
-4.73197330254959));
#449961=CARTESIAN_POINT('Ctrl Pts',(-5.43258626648858,22.5238276902314,
-4.58641880376449));
#449962=CARTESIAN_POINT('Ctrl Pts',(-5.77557608073438,22.5,-4.625917362019));
#449963=CARTESIAN_POINT('Origin',(-5.65685387860012,22.5,-5.65685387860011));
#449964=CARTESIAN_POINT('Ctrl Pts',(-6.39190072013885,22.573038475773,-4.9222125558517));
#449965=CARTESIAN_POINT('Ctrl Pts',(-6.16204455719575,22.5954575429732,
-4.69451421601594));
#449966=CARTESIAN_POINT('Ctrl Pts',(-5.81728522517979,22.6178766101734,
-4.58013776446743));
#449967=CARTESIAN_POINT('Ctrl Pts',(-5.49777863793003,22.6402956773736,
-4.62964039434809));
#449968=CARTESIAN_POINT('Ctrl Pts',(-5.15819698094666,22.664123367605,-4.68225334741615));
#449969=CARTESIAN_POINT('Ctrl Pts',(-4.8471410957032,22.6879510578364,-4.91998587117151));
#449970=CARTESIAN_POINT('Ctrl Pts',(-4.70728537400252,22.7117787480678,
-5.23393572436937));
#449971=CARTESIAN_POINT('Ctrl Pts',(-4.56742965230184,22.7356064382992,
-5.54788557756724));
#449972=CARTESIAN_POINT('Ctrl Pts',(-4.59877409414395,22.7594341285306,
-5.93805276020761));
#449973=CARTESIAN_POINT('Ctrl Pts',(-4.78686738296995,22.783261818762,-6.22570363532513));
#449974=CARTESIAN_POINT('Ctrl Pts',(-4.97496067179595,22.8070895089934,
-6.51335451044265));
#449975=CARTESIAN_POINT('Ctrl Pts',(-5.31980280760584,22.8309171992248,
-6.69848907803731));
#449976=CARTESIAN_POINT('Ctrl Pts',(-5.66347121722023,22.8547448894562,
-6.69629884619592));
#449977=CARTESIAN_POINT('Ctrl Pts',(-6.00713962683461,22.8785725796876,
-6.69410861435453));
#449978=CARTESIAN_POINT('Ctrl Pts',(-6.34963431025348,22.902400269919,-6.5045935830771));
#449979=CARTESIAN_POINT('Ctrl Pts',(-6.53403672593788,22.9262279601503,
-6.21456908983246));
#449980=CARTESIAN_POINT('Ctrl Pts',(-6.71843914162228,22.9500556503817,
-5.92454459658782));
#449981=CARTESIAN_POINT('Ctrl Pts',(-6.7447492895722,22.9738833406131,-5.53401064137597));
#449982=CARTESIAN_POINT('Ctrl Pts',(-6.60092695407667,22.9977110308445,
-5.22186823831326));
#449983=CARTESIAN_POINT('Ctrl Pts',(-6.54996870275417,23.0061535124873,
-5.11127184889382));
#449984=CARTESIAN_POINT('Ctrl Pts',(-6.47765230299322,23.0145959941301,
-5.0105166042882));
#449985=CARTESIAN_POINT('Ctrl Pts',(-6.39037461032892,23.0230384757729,
-4.92436540268704));
#449986=CARTESIAN_POINT('Origin',(-5.65685387860012,26.,-5.65685387860011));
#449987=CARTESIAN_POINT('',(-6.38935290488262,23.4730384757729,-4.92330089590042));
#449988=CARTESIAN_POINT('',(-6.3913110357232,23.3519615242271,-4.92169609601798));
#449989=CARTESIAN_POINT('',(-6.39065394077646,26.,-4.92305381642377));
#449990=CARTESIAN_POINT('Ctrl Pts',(-6.3913110357232,23.3519615242271,-4.92169609601798));
#449991=CARTESIAN_POINT('Ctrl Pts',(-6.61334324490838,23.33007894203,-5.14636061012976));
#449992=CARTESIAN_POINT('Ctrl Pts',(-6.72868171719176,23.308196359833,-5.47994522249351));
#449993=CARTESIAN_POINT('Ctrl Pts',(-6.68738448495221,23.286313777636,-5.79285848911253));
#449994=CARTESIAN_POINT('Ctrl Pts',(-6.64241640721999,23.2624860874046,
-6.1335861198444));
#449995=CARTESIAN_POINT('Ctrl Pts',(-6.41172882390928,23.2386583971732,
-6.44980419113038));
#449996=CARTESIAN_POINT('Ctrl Pts',(-6.10100080909856,23.2148307069418,
-6.59665364733223));
#449997=CARTESIAN_POINT('Ctrl Pts',(-5.79027279428784,23.1910030167104,
-6.74350310353408));
#449998=CARTESIAN_POINT('Ctrl Pts',(-5.39950434797711,23.167175326479,-6.7209839446518));
#449999=CARTESIAN_POINT('Ctrl Pts',(-5.1076985472349,23.1433476362476,-6.539415444341));
#450000=CARTESIAN_POINT('Ctrl Pts',(-4.8158927464927,23.1195199460162,-6.3578469440302));
#450001=CARTESIAN_POINT('Ctrl Pts',(-4.62304959131903,23.0956922557848,
-6.01722910229088));
#450002=CARTESIAN_POINT('Ctrl Pts',(-4.61751951301592,23.0718645655534,
-5.67358993507176));
#450003=CARTESIAN_POINT('Ctrl Pts',(-4.61198943471281,23.048036875322,-5.32995076785264));
#450004=CARTESIAN_POINT('Ctrl Pts',(-4.79377243328026,23.0242091850907,
-4.98329027515371));
#450005=CARTESIAN_POINT('Ctrl Pts',(-5.07957475014376,23.0003814948593,
-4.7924243254548));
#450006=CARTESIAN_POINT('Ctrl Pts',(-5.36537706700727,22.9765538046279,
-4.60155837575589));
#450007=CARTESIAN_POINT('Ctrl Pts',(-5.75519870216683,22.9527261143965,
-4.56648696905699));
#450008=CARTESIAN_POINT('Ctrl Pts',(-6.07050470066555,22.9288984241651,
-4.70325041523271));
#450009=CARTESIAN_POINT('Ctrl Pts',(-6.18932117076026,22.9199194575191,
-4.75478685916323));
#450010=CARTESIAN_POINT('Ctrl Pts',(-6.29755640872372,22.9109404908731,
-4.830723879241));
#450011=CARTESIAN_POINT('Ctrl Pts',(-6.38930388760559,22.9019615242271,
-4.92349966353597));
#450012=CARTESIAN_POINT('Ctrl Pts',(-6.39037461032892,23.0230384757729,
-4.92436540268704));
#450013=CARTESIAN_POINT('Ctrl Pts',(-6.23132356780567,23.0384236843615,
-4.76736722811336));
#450014=CARTESIAN_POINT('Ctrl Pts',(-6.02258634020352,23.0538088929501,
-4.65886881811934));
#450015=CARTESIAN_POINT('Ctrl Pts',(-5.80287677492702,23.0691941015387,
-4.62769529041208));
#450016=CARTESIAN_POINT('Ctrl Pts',(-5.46260375021388,23.0930217917701,
-4.57941559648716));
#450017=CARTESIAN_POINT('Ctrl Pts',(-5.09601251972857,23.1168494820015,
-4.71660705955086));
#450018=CARTESIAN_POINT('Ctrl Pts',(-4.87103919530453,23.1406771722329,
-4.97642324075838));
#450019=CARTESIAN_POINT('Ctrl Pts',(-4.64606587088049,23.1645048624643,
-5.23623942196589));
#450020=CARTESIAN_POINT('Ctrl Pts',(-4.56271045251773,23.1883325526957,
-5.61868032131723));
#450021=CARTESIAN_POINT('Ctrl Pts',(-4.65915585483332,23.2121602429271,
-5.94855238336812));
#450022=CARTESIAN_POINT('Ctrl Pts',(-4.75560125714891,23.2359879331585,
-6.27842444541901));
#450023=CARTESIAN_POINT('Ctrl Pts',(-5.03184748014285,23.2598156233899,
-6.55572767016945));
#450024=CARTESIAN_POINT('Ctrl Pts',(-5.36134886181892,23.2836433136212,
-6.65343136663416));
#450025=CARTESIAN_POINT('Ctrl Pts',(-5.690850243495,23.3074710038526,-6.75113506309887));
#450026=CARTESIAN_POINT('Ctrl Pts',(-6.07360678385322,23.331298694084,-6.66923923127783));
#450027=CARTESIAN_POINT('Ctrl Pts',(-6.33427992409048,23.3551263843154,
-6.4452597843657));
#450028=CARTESIAN_POINT('Ctrl Pts',(-6.59495306432775,23.3789540745468,
-6.22128033745358));
#450029=CARTESIAN_POINT('Ctrl Pts',(-6.73354280444407,23.4027817647782,
-5.85521727545038));
#450030=CARTESIAN_POINT('Ctrl Pts',(-6.6865623548039,23.4266094550096,-5.51476156795534));
#450031=CARTESIAN_POINT('Ctrl Pts',(-6.65604804910002,23.442085795264,-5.29363193601897));
#450032=CARTESIAN_POINT('Ctrl Pts',(-6.54724832815155,23.4575621355185,
-5.08330512959901));
#450033=CARTESIAN_POINT('Ctrl Pts',(-6.38935290488262,23.4730384757729,
-4.92330089590042));
#450034=CARTESIAN_POINT('Origin',(-5.65685387860012,26.,-5.65685387860011));
#450035=CARTESIAN_POINT('',(-6.39152331859132,23.9230384757729,-4.9216948349357));
#450036=CARTESIAN_POINT('',(-6.39146732321148,23.8019615242271,-4.92356615355223));
#450037=CARTESIAN_POINT('',(-6.39065394077646,26.,-4.92305381642377));
#450038=CARTESIAN_POINT('Ctrl Pts',(-6.39146732321148,23.8019615242271,
-4.92356615355223));
#450039=CARTESIAN_POINT('Ctrl Pts',(-6.44404636753914,23.7968727736498,
-4.97518123721477));
#450040=CARTESIAN_POINT('Ctrl Pts',(-6.49097569651667,23.7917840230725,
-5.03225965778749));
#450041=CARTESIAN_POINT('Ctrl Pts',(-6.53072214720976,23.7866952724952,
-5.09396482100832));
#450042=CARTESIAN_POINT('Ctrl Pts',(-6.71683190058211,23.7628675822638,
-5.38289458727869));
#450043=CARTESIAN_POINT('Ctrl Pts',(-6.74545633697037,23.7390398920324,
-5.77326614382955));
#450044=CARTESIAN_POINT('Ctrl Pts',(-6.60348277515141,23.715212201801,-6.08625298439034));
#450045=CARTESIAN_POINT('Ctrl Pts',(-6.46150921333244,23.6913845115696,
-6.39923982495114));
#450046=CARTESIAN_POINT('Ctrl Pts',(-6.14893765330626,23.6675568213382,
-6.63484194952187));
#450047=CARTESIAN_POINT('Ctrl Pts',(-5.80895502137128,23.6437291311068,
-6.68513161677842));
#450048=CARTESIAN_POINT('Ctrl Pts',(-5.4689723894363,23.6199014408755,-6.73542128403497));
#450049=CARTESIAN_POINT('Ctrl Pts',(-5.10157868559252,23.5960737506441,
-6.60039849397735));
#450050=CARTESIAN_POINT('Ctrl Pts',(-4.87507434314934,23.5722460604127,
-6.34191631672375));
#450051=CARTESIAN_POINT('Ctrl Pts',(-4.64857000070616,23.5484183701813,
-6.08343413947014));
#450052=CARTESIAN_POINT('Ctrl Pts',(-4.56295501966359,23.5245906799499,
-5.70149257502055));
#450053=CARTESIAN_POINT('Ctrl Pts',(-4.65744921450722,23.5007629897185,
-5.37105630657982));
#450054=CARTESIAN_POINT('Ctrl Pts',(-4.75194340935084,23.4769352994871,
-5.04062003813909));
#450055=CARTESIAN_POINT('Ctrl Pts',(-5.02654678008065,23.4531076092557,
-4.76168906570723));
#450056=CARTESIAN_POINT('Ctrl Pts',(-5.35546505814245,23.4292799190243,
-4.66203997694959));
#450057=CARTESIAN_POINT('Ctrl Pts',(-5.68438333620426,23.4054522287929,
-4.56239088819195));
#450058=CARTESIAN_POINT('Ctrl Pts',(-6.06761652159808,23.3816245385615,
-4.64202368310855));
#450059=CARTESIAN_POINT('Ctrl Pts',(-6.32960882821811,23.3577968483301,
-4.86445867565572));
#450060=CARTESIAN_POINT('Ctrl Pts',(-6.350995850443,23.3558517402958,-4.88261654521522));
#450061=CARTESIAN_POINT('Ctrl Pts',(-6.37157494470416,23.3539066322614,
-4.90172602358781));
#450062=CARTESIAN_POINT('Ctrl Pts',(-6.3913110357232,23.3519615242271,-4.92169609601798));
#450063=CARTESIAN_POINT('Ctrl Pts',(-6.38935290488262,23.4730384757729,
-4.92330089590042));
#450064=CARTESIAN_POINT('Ctrl Pts',(-6.30414930262286,23.4813898257499,
-4.83695933636888));
#450065=CARTESIAN_POINT('Ctrl Pts',(-6.20464951053553,23.4897411757268,
-4.76527121936352));
#450066=CARTESIAN_POINT('Ctrl Pts',(-6.09544017298549,23.4980925257038,
-4.71444637045848));
#450067=CARTESIAN_POINT('Ctrl Pts',(-5.78384908020389,23.5219202159352,
-4.56943523344352));
#450068=CARTESIAN_POINT('Ctrl Pts',(-5.39321753403732,23.5457479061666,
-4.59426131240047));
#450069=CARTESIAN_POINT('Ctrl Pts',(-5.10249121190879,23.569575596398,-4.77755195197114));
#450070=CARTESIAN_POINT('Ctrl Pts',(-4.81176488978025,23.5934032866293,
-4.9608425915418));
#450071=CARTESIAN_POINT('Ctrl Pts',(-4.62094379168974,23.6172309768607,
-5.30259779172617));
#450072=CARTESIAN_POINT('Ctrl Pts',(-4.61744171997954,23.6410586670921,
-5.64626184853499));
#450073=CARTESIAN_POINT('Ctrl Pts',(-4.61393964826935,23.6648863573235,
-5.98992590534381));
#450074=CARTESIAN_POINT('Ctrl Pts',(-4.79775660293947,23.6887140475549,
-6.33549881877709));
#450075=CARTESIAN_POINT('Ctrl Pts',(-5.08468731748426,23.7125417377863,
-6.52467601704459));
#450076=CARTESIAN_POINT('Ctrl Pts',(-5.37161803202905,23.7363694280177,
-6.71385321531209));
#450077=CARTESIAN_POINT('Ctrl Pts',(-5.76166250644852,23.7601971182491,
-6.74663469841383));
#450078=CARTESIAN_POINT('Ctrl Pts',(-6.07614404554655,23.7840248084805,
-6.60800349462427));
#450079=CARTESIAN_POINT('Ctrl Pts',(-6.39062558464459,23.8078524987119,
-6.46937229083472));
#450080=CARTESIAN_POINT('Ctrl Pts',(-6.6295441884212,23.8316801889433,-6.15932840015388));
#450081=CARTESIAN_POINT('Ctrl Pts',(-6.6834528935629,23.8555078791747,-5.81990079386588));
#450082=CARTESIAN_POINT('Ctrl Pts',(-6.73438085433327,23.8780180780408,
-5.49924097144978));
#450083=CARTESIAN_POINT('Ctrl Pts',(-6.62019259508593,23.9005282769068,
-5.15235699515365));
#450084=CARTESIAN_POINT('Ctrl Pts',(-6.39152331859132,23.9230384757729,
-4.9216948349357));
#450085=CARTESIAN_POINT('Origin',(-5.65685387860012,26.,-5.65685387860011));
#450086=CARTESIAN_POINT('',(-6.39128196913613,24.3730384757729,-4.92377157353715));
#450087=CARTESIAN_POINT('',(-6.38942086037359,24.2519615242271,-4.92421628016771));
#450088=CARTESIAN_POINT('',(-6.39065394077646,26.,-4.92305381642377));
#450089=CARTESIAN_POINT('Ctrl Pts',(-6.38942086037359,24.2519615242271,
-4.92421628016771));
#450090=CARTESIAN_POINT('Ctrl Pts',(-6.51405309196749,24.2398389150381,
-5.04895543667044));
#450091=CARTESIAN_POINT('Ctrl Pts',(-6.60860369693141,24.2277163058492,
-5.20382475542584));
#450092=CARTESIAN_POINT('Ctrl Pts',(-6.65652287894995,24.2155936966603,
-5.37198243345446));
#450093=CARTESIAN_POINT('Ctrl Pts',(-6.75071080561528,24.1917660064289,
-5.70250608555364));
#450094=CARTESIAN_POINT('Ctrl Pts',(-6.66474206054895,24.1679383161975,
-6.08436822205294));
#450095=CARTESIAN_POINT('Ctrl Pts',(-6.4379983333991,24.1441106259661,-6.34264042812557));
#450096=CARTESIAN_POINT('Ctrl Pts',(-6.21125460624925,24.1202829357347,
-6.60091263419821));
#450097=CARTESIAN_POINT('Ctrl Pts',(-5.84373589701587,24.0964552455033,
-6.73559490984418));
#450098=CARTESIAN_POINT('Ctrl Pts',(-5.5037999963824,24.0726275552719,-6.68499023152592));
#450099=CARTESIAN_POINT('Ctrl Pts',(-5.16386409574893,24.0487998650405,
-6.63438555320766));
#450100=CARTESIAN_POINT('Ctrl Pts',(-4.85151100371537,24.0249721748091,
-6.39849392092517));
#450101=CARTESIAN_POINT('Ctrl Pts',(-4.70982751913656,24.0011444845777,
-6.08537566804496));
#450102=CARTESIAN_POINT('Ctrl Pts',(-4.56814403455775,23.9773167943464,
-5.77225741516475));
#450103=CARTESIAN_POINT('Ctrl Pts',(-4.59713015743369,23.9534891041149,
-5.38191254168682));
#450104=CARTESIAN_POINT('Ctrl Pts',(-4.78350754767415,23.9296614138835,
-5.09315534403941));
#450105=CARTESIAN_POINT('Ctrl Pts',(-4.96988493791459,23.9058337236522,
-4.804398146392));
#450106=CARTESIAN_POINT('Ctrl Pts',(-5.31365359551954,23.8820060334208,
-4.61722862457511));
#450107=CARTESIAN_POINT('Ctrl Pts',(-5.65733545950024,23.8581783431894,
-4.6173878516616));
#450108=CARTESIAN_POINT('Ctrl Pts',(-5.92761905169082,23.8394394035353,
-4.61751307348277));
#450109=CARTESIAN_POINT('Ctrl Pts',(-6.19784896370209,23.8207004638812,
-4.73349750638545));
#450110=CARTESIAN_POINT('Ctrl Pts',(-6.39146732321148,23.8019615242271,
-4.92356615355223));
#450111=CARTESIAN_POINT('Ctrl Pts',(-6.39152331859132,23.9230384757729,
-4.9216948349357));
#450112=CARTESIAN_POINT('Ctrl Pts',(-6.37813961642664,23.9243559671382,
-4.90819449199352));
#450113=CARTESIAN_POINT('Ctrl Pts',(-6.3643637478711,23.9256734585035,-4.895092278726));
#450114=CARTESIAN_POINT('Ctrl Pts',(-6.35020586507153,23.9269909498688,
-4.88241675495565));
#450115=CARTESIAN_POINT('Ctrl Pts',(-6.0941513249317,23.9508186401002,-4.65317164422858));
#450116=CARTESIAN_POINT('Ctrl Pts',(-5.71314343814525,23.9746463303316,
-4.56349274466962));
#450117=CARTESIAN_POINT('Ctrl Pts',(-5.38171929489582,23.998474020563,-4.6544613426263));
#450118=CARTESIAN_POINT('Ctrl Pts',(-5.0502951516464,24.0223017107944,-4.74542994058297));
#450119=CARTESIAN_POINT('Ctrl Pts',(-4.76845475193401,24.0461294010258,
-5.01704603605528));
#450120=CARTESIAN_POINT('Ctrl Pts',(-4.6653072414873,24.0699570912572,-5.34488416612327));
#450121=CARTESIAN_POINT('Ctrl Pts',(-4.56215973104059,24.0937847814886,
-5.67272229619127));
#450122=CARTESIAN_POINT('Ctrl Pts',(-4.63770510985959,24.11761247172,-6.05678246085496));
#450123=CARTESIAN_POINT('Ctrl Pts',(-4.8573365604447,24.1414401619514,-6.32112934350159));
#450124=CARTESIAN_POINT('Ctrl Pts',(-5.07696801102981,24.1652678521828,
-6.58547622614821));
#450125=CARTESIAN_POINT('Ctrl Pts',(-5.44068553338104,24.1890955424141,
-6.73010982677778));
#450126=CARTESIAN_POINT('Ctrl Pts',(-5.78187263496817,24.2129232326455,
-6.68877448884911));
#450127=CARTESIAN_POINT('Ctrl Pts',(-6.12305973655531,24.2367509228769,
-6.64743915092045));
#450128=CARTESIAN_POINT('Ctrl Pts',(-6.44171641737836,24.2605786131083,
-6.42013487443355));
#450129=CARTESIAN_POINT('Ctrl Pts',(-6.59186824658804,24.2844063033397,
-6.11098818332588));
#450130=CARTESIAN_POINT('Ctrl Pts',(-6.74202007579772,24.3082339935711,
-5.80184149221821));
#450131=CARTESIAN_POINT('Ctrl Pts',(-6.72366705339403,24.3320616838025,
-5.41085238648977));
#450132=CARTESIAN_POINT('Ctrl Pts',(-6.54521657215205,24.3558893740339,
-5.11713028264445));
#450133=CARTESIAN_POINT('Ctrl Pts',(-6.50240552012982,24.3616057412803,
-5.04666506349635));
#450134=CARTESIAN_POINT('Ctrl Pts',(-6.45038020112141,24.3673221085266,
-4.98179796021342));
#450135=CARTESIAN_POINT('Ctrl Pts',(-6.39128196913613,24.3730384757729,
-4.92377157353715));
#450136=CARTESIAN_POINT('Origin',(-5.65685387860012,26.,-5.65685387860011));
#450137=CARTESIAN_POINT('',(-6.38933869113556,24.8230384757729,-4.92408802232565));
#450138=CARTESIAN_POINT('',(-6.39028821611916,24.7019615242271,-4.92212745780798));
#450139=CARTESIAN_POINT('',(-6.39065394077646,26.,-4.92305381642377));
#450140=CARTESIAN_POINT('Ctrl Pts',(-6.39028821611916,24.7019615242271,
-4.92212745780798));
#450141=CARTESIAN_POINT('Ctrl Pts',(-6.5845155347103,24.6828050564265,-5.11995795053563));
#450142=CARTESIAN_POINT('Ctrl Pts',(-6.70087353526984,24.6636485886259,
-5.39828521249021));
#450143=CARTESIAN_POINT('Ctrl Pts',(-6.69616935490973,24.6444921208254,
-5.67455106061111));
#450144=CARTESIAN_POINT('Ctrl Pts',(-6.69031808036474,24.620664430594,-6.01818314973456));
#450145=CARTESIAN_POINT('Ctrl Pts',(-6.49716519325234,24.5968367403626,
-6.35862591802897));
#450146=CARTESIAN_POINT('Ctrl Pts',(-6.20519269912468,24.5730090501312,
-6.53992487743045));
#450147=CARTESIAN_POINT('Ctrl Pts',(-5.91322020499702,24.5491813598998,
-6.72122383683193));
#450148=CARTESIAN_POINT('Ctrl Pts',(-5.52242810385412,24.5253536696684,
-6.74337898734047));
#450149=CARTESIAN_POINT('Ctrl Pts',(-5.21183556708661,24.501525979437,-6.59624120723028));
#450150=CARTESIAN_POINT('Ctrl Pts',(-4.9012430303191,24.4776982892056,-6.44910342712008));
#450151=CARTESIAN_POINT('Ctrl Pts',(-4.670850057927,24.4538705989742,-6.13267271639114));
#450152=CARTESIAN_POINT('Ctrl Pts',(-4.62619808347199,24.4300429087428,
-5.7919038045113));
#450153=CARTESIAN_POINT('Ctrl Pts',(-4.58154610901698,24.4062152185114,
-5.45113489263147));
#450154=CARTESIAN_POINT('Ctrl Pts',(-4.72263513249906,24.38238752828,-5.08602777960075));
#450155=CARTESIAN_POINT('Ctrl Pts',(-4.98483324415836,24.3585598380486,
-4.86383551964991));
#450156=CARTESIAN_POINT('Ctrl Pts',(-5.24703135581765,24.3347321478172,
-4.64164325969907));
#450157=CARTESIAN_POINT('Ctrl Pts',(-5.63033855565415,24.3109044575858,
-4.56236585282811));
#450158=CARTESIAN_POINT('Ctrl Pts',(-5.9591644547709,24.2870767673545,-4.66231973324216));
#450159=CARTESIAN_POINT('Ctrl Pts',(-6.12069642705377,24.275371686312,-4.71142093690032));
#450160=CARTESIAN_POINT('Ctrl Pts',(-6.26908122485669,24.2636666052695,
-4.80377340246064));
#450161=CARTESIAN_POINT('Ctrl Pts',(-6.38942086037359,24.2519615242271,
-4.92421628016771));
#450162=CARTESIAN_POINT('Ctrl Pts',(-6.39128196913613,24.3730384757729,
-4.92377157353715));
#450163=CARTESIAN_POINT('Ctrl Pts',(-6.20403942134221,24.391149798758,-4.7399249826062));
#450164=CARTESIAN_POINT('Ctrl Pts',(-5.94579686164739,24.4092611217431,
-4.62474754709557));
#450165=CARTESIAN_POINT('Ctrl Pts',(-5.68465923264326,24.4273724447281,
-4.61775970678069));
#450166=CARTESIAN_POINT('Ctrl Pts',(-5.34110031445674,24.4512001349595,
-4.60856633672445));
#450167=CARTESIAN_POINT('Ctrl Pts',(-4.99253041816396,24.4750278251909,
-4.78663469857419));
#450168=CARTESIAN_POINT('Ctrl Pts',(-4.79862701145602,24.4988555154223,
-5.07039290068915));
#450169=CARTESIAN_POINT('Ctrl Pts',(-4.60472360474809,24.5226832056536,
-5.35415110280411));
#450170=CARTESIAN_POINT('Ctrl Pts',(-4.565486687625,24.546510895885,-5.7435991451843));
#450171=CARTESIAN_POINT('Ctrl Pts',(-4.69889042440694,24.5703385861164,
-6.06033356407531));
#450172=CARTESIAN_POINT('Ctrl Pts',(-4.83229416118888,24.5941662763478,
-6.37706798296632));
#450173=CARTESIAN_POINT('Ctrl Pts',(-5.13833855187585,24.6179939665792,
-6.62108877836816));
#450174=CARTESIAN_POINT('Ctrl Pts',(-5.47682676316715,24.6418216568106,
-6.68061169925027));
#450175=CARTESIAN_POINT('Ctrl Pts',(-5.81531497445846,24.665649347042,-6.74013462013239));
#450176=CARTESIAN_POINT('Ctrl Pts',(-6.18624700635411,24.6894770372734,
-6.61515966649478));
#450177=CARTESIAN_POINT('Ctrl Pts',(-6.41970146010492,24.7133047275048,
-6.36293701391879));
#450178=CARTESIAN_POINT('Ctrl Pts',(-6.65315591385573,24.7371324177362,
-6.1107143613428));
#450179=CARTESIAN_POINT('Ctrl Pts',(-6.74913278946171,24.7609601079676,
-5.73124400982843));
#450180=CARTESIAN_POINT('Ctrl Pts',(-6.6636657201663,24.784787798199,-5.39835869474429));
#450181=CARTESIAN_POINT('Ctrl Pts',(-6.61793218802978,24.797538024057,-5.22023136007979));
#450182=CARTESIAN_POINT('Ctrl Pts',(-6.5202452116208,24.8102882499149,-5.05544287282308));
#450183=CARTESIAN_POINT('Ctrl Pts',(-6.38933869113556,24.8230384757729,
-4.92408802232565));
#450184=CARTESIAN_POINT('Origin',(-5.65685387860012,26.,-5.65685387860011));
#450185=CARTESIAN_POINT('',(-6.39051881327128,25.2730384757729,-4.92197603118329));
#450186=CARTESIAN_POINT('',(-6.39198798715976,25.1519615242271,-4.92254817630007));
#450187=CARTESIAN_POINT('',(-6.39065394077646,26.,-4.92305381642377));
#450188=CARTESIAN_POINT('Ctrl Pts',(-6.39198798715976,25.1519615242271,
-4.92254817630007));
#450189=CARTESIAN_POINT('Ctrl Pts',(-6.41627314991444,25.1495988880462,
-4.94650751599249));
#450190=CARTESIAN_POINT('Ctrl Pts',(-6.43929566708609,25.1472362518654,
-4.97169983154625));
#450191=CARTESIAN_POINT('Ctrl Pts',(-6.46089355482011,25.1448736156846,
-4.99805942366946));
#450192=CARTESIAN_POINT('Ctrl Pts',(-6.67871286308055,25.1210459254532,
-5.26390153716753));
#450193=CARTESIAN_POINT('Ctrl Pts',(-6.75163093056004,25.0972182352218,
-5.64846913729549));
#450194=CARTESIAN_POINT('Ctrl Pts',(-6.64624470558553,25.0733905449904,
-5.97559449046916));
#450195=CARTESIAN_POINT('Ctrl Pts',(-6.54085848061101,25.049562854759,-6.30271984364283));
#450196=CARTESIAN_POINT('Ctrl Pts',(-6.25716796318249,25.0257351645276,
-6.57240294986222));
#450197=CARTESIAN_POINT('Ctrl Pts',(-5.92512971718013,25.0019074742962,
-6.66110381706144));
#450198=CARTESIAN_POINT('Ctrl Pts',(-5.59309147117778,24.9780797840648,
-6.74980468426065));
#450199=CARTESIAN_POINT('Ctrl Pts',(-5.21270549660159,24.9542520938335,
-6.65752331243968));
#450200=CARTESIAN_POINT('Ctrl Pts',(-4.95822404429259,24.9304244036021,
-6.42653317184816));
#450201=CARTESIAN_POINT('Ctrl Pts',(-4.70374259198359,24.9065967133707,
-6.19554303125664));
#450202=CARTESIAN_POINT('Ctrl Pts',(-4.57516566194178,24.8827690231393,
-5.82584412189456));
#450203=CARTESIAN_POINT('Ctrl Pts',(-4.63139343216518,24.8589413329079,
-5.48679296352304));
#450204=CARTESIAN_POINT('Ctrl Pts',(-4.68762120238858,24.8351136426765,
-5.14774180515151));
#450205=CARTESIAN_POINT('Ctrl Pts',(-4.9286536728772,24.8112859524451,-4.83933839777055));
#450206=CARTESIAN_POINT('Ctrl Pts',(-5.24407554312886,24.7874582622137,
-4.70286022094558));
#450207=CARTESIAN_POINT('Ctrl Pts',(-5.55949741338051,24.7636305719823,
-4.56638204412062));
#450208=CARTESIAN_POINT('Ctrl Pts',(-5.94930868339519,24.7398028817509,
-4.60182909785165));
#450209=CARTESIAN_POINT('Ctrl Pts',(-6.23493948741374,24.7159751915195,
-4.79296332969341));
#450210=CARTESIAN_POINT('Ctrl Pts',(-6.29093505415592,24.7113039690887,
-4.83043362171106));
#450211=CARTESIAN_POINT('Ctrl Pts',(-6.34292671833547,24.7066327466579,
-4.87388734148021));
#450212=CARTESIAN_POINT('Ctrl Pts',(-6.39028821611916,24.7019615242271,
-4.92212745780798));
#450213=CARTESIAN_POINT('Ctrl Pts',(-6.38933869113556,24.8230384757729,
-4.92408802232565));
#450214=CARTESIAN_POINT('Ctrl Pts',(-6.27560640646284,24.8341159401463,
-4.80996622614209));
#450215=CARTESIAN_POINT('Ctrl Pts',(-6.13679925493306,24.8451934045197,
-4.72108089883846));
#450216=CARTESIAN_POINT('Ctrl Pts',(-5.98520281626299,24.8562708688931,
-4.67061008310121));
#450217=CARTESIAN_POINT('Ctrl Pts',(-5.65911799585187,24.8800985591245,
-4.56204706519615));
#450218=CARTESIAN_POINT('Ctrl Pts',(-5.27385936922642,24.9039262493559,
-4.63122130803993));
#450219=CARTESIAN_POINT('Ctrl Pts',(-5.00591117956891,24.9277539395873,
-4.84644449237099));
#450220=CARTESIAN_POINT('Ctrl Pts',(-4.7379629899114,24.9515816298187,-5.06166767670205));
#450221=CARTESIAN_POINT('Ctrl Pts',(-4.58732523722183,24.9754093200501,
-5.42293980252039));
#450222=CARTESIAN_POINT('Ctrl Pts',(-4.62300419682159,24.9992370102815,
-5.76476474386039));
#450223=CARTESIAN_POINT('Ctrl Pts',(-4.65868315642135,25.0230647005129,
-6.10658968520039));
#450224=CARTESIAN_POINT('Ctrl Pts',(-4.88067882831045,25.0468923907443,
-6.42896744206204));
#450225=CARTESIAN_POINT('Ctrl Pts',(-5.18729621377842,25.0707200809757,
-6.58421869570625));
#450226=CARTESIAN_POINT('Ctrl Pts',(-5.4939135992464,25.0945477712071,-6.73946994935045));
#450227=CARTESIAN_POINT('Ctrl Pts',(-5.88515269829325,25.1183754614385,
-6.72759469977719));
#450228=CARTESIAN_POINT('Ctrl Pts',(-6.18179018209155,25.1422031516699,
-6.5540334824637));
#450229=CARTESIAN_POINT('Ctrl Pts',(-6.47842766588984,25.1660308419013,
-6.38047226515022));
#450230=CARTESIAN_POINT('Ctrl Pts',(-6.68046353443956,25.1898585321326,
-6.04522508009649));
#450231=CARTESIAN_POINT('Ctrl Pts',(-6.69534535485933,25.213686222364,-5.70186524531576));
#450232=CARTESIAN_POINT('Ctrl Pts',(-6.70770170116849,25.2334703068337,
-5.41677424787487));
#450233=CARTESIAN_POINT('Ctrl Pts',(-6.59103501365993,25.2532543913033,
-5.12609043162756));
#450234=CARTESIAN_POINT('Ctrl Pts',(-6.39051881327128,25.2730384757729,
-4.92197603118329));
#450235=CARTESIAN_POINT('Origin',(-5.65685387860012,26.,-5.65685387860011));
#450236=CARTESIAN_POINT('',(-6.39190058798136,25.7230384757729,-4.92276701974739));
#450237=CARTESIAN_POINT('',(-6.39006796800885,25.6019615242271,-4.92443355077908));
#450238=CARTESIAN_POINT('',(-6.39065394077646,26.,-4.92305381642377));
#450239=CARTESIAN_POINT('',(-5.59475217632209,26.,-6.69274404704181));
#450240=CARTESIAN_POINT('Ctrl Pts',(-6.39190058798136,25.7230384757729,
-4.92276701974739));
#450241=CARTESIAN_POINT('Ctrl Pts',(-6.17742942344334,25.7438759131544,
-4.71160994855805));
#450242=CARTESIAN_POINT('Ctrl Pts',(-5.86562000134797,25.764713350536,-4.59523934827088));
#450243=CARTESIAN_POINT('Ctrl Pts',(-5.56615422141077,25.7855507879175,
-4.62142687258513));
#450244=CARTESIAN_POINT('Ctrl Pts',(-5.22371394391399,25.8093784781489,
-4.65137240791476));
#450245=CARTESIAN_POINT('Ctrl Pts',(-4.8974142264151,25.8332061683802,-4.86772710302321));
#450246=CARTESIAN_POINT('Ctrl Pts',(-4.7372531902219,25.8570338586116,-5.17187737628347));
#450247=CARTESIAN_POINT('Ctrl Pts',(-4.57709215402869,25.880861548843,-5.47602764954372));
#450248=CARTESIAN_POINT('Ctrl Pts',(-4.58306979914119,25.9046892390744,
-5.86797350095578));
#450249=CARTESIAN_POINT('Ctrl Pts',(-4.75132533448083,25.9285169293058,
-6.16698733288025));
#450250=CARTESIAN_POINT('Ctrl Pts',(-4.91958086982048,25.9523446195372,
-6.46600116480472));
#450251=CARTESIAN_POINT('Ctrl Pts',(-5.25011429538726,25.9761723097686,
-6.67208297724159));
#450252=CARTESIAN_POINT('Ctrl Pts',(-5.59475217632212,26.,-6.69274404704181));
#450253=CARTESIAN_POINT('',(-6.69457727933146,26.,-5.59444809180803));
#450254=CARTESIAN_POINT('Origin',(-5.65685387860012,26.,-5.65685387860011));
#450255=CARTESIAN_POINT('Ctrl Pts',(-6.69458228414866,26.,-5.59444726164187));
#450256=CARTESIAN_POINT('Ctrl Pts',(-6.71351646533255,25.9770624644402,
-5.92484673178863));
#450257=CARTESIAN_POINT('Ctrl Pts',(-6.56158375468957,25.9541249288804,
-6.26627937525033));
#450258=CARTESIAN_POINT('Ctrl Pts',(-6.30214239804398,25.9311873933205,
-6.47167795527827));
#450259=CARTESIAN_POINT('Ctrl Pts',(-6.03263270014108,25.9073597030892,
-6.68504759676004));
#450260=CARTESIAN_POINT('Ctrl Pts',(-5.64710810132191,25.8835320128578,
-6.75161994353754));
#450261=CARTESIAN_POINT('Ctrl Pts',(-5.32182159136528,25.8597043226264,
-6.64083855948586));
#450262=CARTESIAN_POINT('Ctrl Pts',(-4.99653508140864,25.835876632395,-6.53005717543418));
#450263=CARTESIAN_POINT('Ctrl Pts',(-4.73148666031454,25.8120489421636,
-6.24192206055332));
#450264=CARTESIAN_POINT('Ctrl Pts',(-4.64827248224482,25.7882212519322,
-5.90845611919746));
#450265=CARTESIAN_POINT('Ctrl Pts',(-4.56505830417509,25.7643935617008,
-5.5749901778416));
#450266=CARTESIAN_POINT('Ctrl Pts',(-4.66367836912974,25.7405658714694,
-5.19619341001074));
#450267=CARTESIAN_POINT('Ctrl Pts',(-4.89886414913017,25.716738181238,-4.94557465216384));
#450268=CARTESIAN_POINT('Ctrl Pts',(-5.13404992913059,25.6929104910066,
-4.69495589431694));
#450269=CARTESIAN_POINT('Ctrl Pts',(-5.50580142417678,25.6690828007752,
-4.572515146454));
#450270=CARTESIAN_POINT('Ctrl Pts',(-5.84386841174159,25.6452551105439,
-4.63434949773116));
#450271=CARTESIAN_POINT('Ctrl Pts',(-6.04861804217652,25.6308239151049,
-4.67179935541582));
#450272=CARTESIAN_POINT('Ctrl Pts',(-6.24101187097706,25.616392719666,-4.7768430935332));
#450273=CARTESIAN_POINT('Ctrl Pts',(-6.39006796800885,25.6019615242271,
-4.92443355077908));
#450274=CARTESIAN_POINT('Origin',(-5.65685387860012,26.993675081176,-5.65685387860011));
#450275=CARTESIAN_POINT('',(-6.5673434103921,22.756324918824,-4.74524035180399));
#450276=CARTESIAN_POINT('',(-6.57057146528766,22.718675081176,-4.74364038176038));
#450277=CARTESIAN_POINT('',(-6.56902162633079,26.993675081176,-4.74468613086949));
#450278=CARTESIAN_POINT('',(-4.8286920333622,22.5,-6.64591806159944));
#450279=CARTESIAN_POINT('Ctrl Pts',(-6.57057146528766,22.718675081176,-4.74364038176038));
#450280=CARTESIAN_POINT('Ctrl Pts',(-6.58852418981576,22.7172664581449,
-4.76142457130848));
#450281=CARTESIAN_POINT('Ctrl Pts',(-6.9000556810006,22.6920301448823,-5.09000197050781));
#450282=CARTESIAN_POINT('Ctrl Pts',(-7.12689194633153,22.6429661413884,
-6.06611679986992));
#450283=CARTESIAN_POINT('Ctrl Pts',(-6.10694434613243,22.5714830706942,
-7.11331947438321));
#450284=CARTESIAN_POINT('Ctrl Pts',(-5.15775103452081,22.5238276902314,
-6.92144528650133));
#450285=CARTESIAN_POINT('Ctrl Pts',(-4.8286920333622,22.5,-6.64591806159944));
#450286=CARTESIAN_POINT('',(-4.44194770692244,22.5,-6.09734856608926));
#450287=CARTESIAN_POINT('Origin',(-5.65685387860012,22.5,-5.65685387860011));
#450288=CARTESIAN_POINT('Ctrl Pts',(-6.5673434103921,22.756324918824,-4.74524035180399));
#450289=CARTESIAN_POINT('Ctrl Pts',(-6.75594870135602,22.7414761952386,
-4.93595953019022));
#450290=CARTESIAN_POINT('Ctrl Pts',(-7.1012121014615,22.7027997814218,-5.58182921801751));
#450291=CARTESIAN_POINT('Ctrl Pts',(-6.68055232418451,22.6402956773736,
-6.78713386963136));
#450292=CARTESIAN_POINT('Ctrl Pts',(-5.27997950888059,22.5697027613511,
-7.12528591239125));
#450293=CARTESIAN_POINT('Ctrl Pts',(-4.58325719964658,22.5229375355598,
-6.48370144903282));
#450294=CARTESIAN_POINT('Ctrl Pts',(-4.44194158662797,22.5,-6.09735008669021));
#450295=CARTESIAN_POINT('Origin',(-5.65685387860012,26.993675081176,-5.65685387860011));
#450296=CARTESIAN_POINT('',(-6.56983844394705,23.206324918824,-4.74299838399068));
#450297=CARTESIAN_POINT('',(-6.56867439792569,23.168675081176,-4.74631652959707));
#450298=CARTESIAN_POINT('',(-6.56902162633079,26.993675081176,-4.74468613086949));
#450299=CARTESIAN_POINT('Ctrl Pts',(-6.56867439792569,23.168675081176,-4.74631652959707));
#450300=CARTESIAN_POINT('Ctrl Pts',(-6.67716702479821,23.1602325995332,
-4.853408844765));
#450301=CARTESIAN_POINT('Ctrl Pts',(-7.02077633180239,23.127962427659,-5.33214451040114));
#450302=CARTESIAN_POINT('Ctrl Pts',(-6.94377741359719,23.0718645655535,
-6.47507582842176));
#450303=CARTESIAN_POINT('Ctrl Pts',(-5.66653874837813,23.0003814948592,
-7.18181942856023));
#450304=CARTESIAN_POINT('Ctrl Pts',(-4.38054591235379,22.9288984241651,
-6.49141154940691));
#450305=CARTESIAN_POINT('Ctrl Pts',(-4.26365553420012,22.8574153534709,
-5.03639155729104));
#450306=CARTESIAN_POINT('Ctrl Pts',(-5.40079341912851,22.7873409058079,
-4.16730445086878));
#450307=CARTESIAN_POINT('Ctrl Pts',(-6.28484325502835,22.7410941483762,
-4.46059450521194));
#450308=CARTESIAN_POINT('Ctrl Pts',(-6.57057146528766,22.718675081176,-4.74364038176038));
#450309=CARTESIAN_POINT('Ctrl Pts',(-6.56983844394705,23.206324918824,-4.74299838399068));
#450310=CARTESIAN_POINT('Ctrl Pts',(-6.84584090104065,23.184442336627,-5.02227299078827));
#450311=CARTESIAN_POINT('Ctrl Pts',(-7.14533371342118,23.1387320641985,
-5.8884730690954));
#450312=CARTESIAN_POINT('Ctrl Pts',(-6.3084575374563,23.0691941015387,-7.03563221165043));
#450313=CARTESIAN_POINT('Ctrl Pts',(-4.85119529970874,22.9977110308445,
-6.95165327175697));
#450314=CARTESIAN_POINT('Ctrl Pts',(-4.13204038713624,22.9262279601503,
-5.68141376558385));
#450315=CARTESIAN_POINT('Ctrl Pts',(-4.80994952176022,22.8547448894562,
-4.38863987327371));
#450316=CARTESIAN_POINT('Ctrl Pts',(-5.9617065202947,22.7981105423474,-4.28501879514302));
#450317=CARTESIAN_POINT('Ctrl Pts',(-6.45329450867432,22.76530388547,-4.62991319040622));
#450318=CARTESIAN_POINT('Ctrl Pts',(-6.5673434103921,22.756324918824,-4.74524035180399));
#450319=CARTESIAN_POINT('Origin',(-5.65685387860012,26.993675081176,-5.65685387860011));
#450320=CARTESIAN_POINT('',(-6.57003272085371,23.656324918824,-4.74532300381163));
#450321=CARTESIAN_POINT('',(-6.56740434249263,23.618675081176,-4.74499326893249));
#450322=CARTESIAN_POINT('',(-6.56902162633079,26.993675081176,-4.74468613086949));
#450323=CARTESIAN_POINT('Ctrl Pts',(-6.56740434249263,23.618675081176,-4.74499326893249));
#450324=CARTESIAN_POINT('Ctrl Pts',(-6.76368003125862,23.6031987409216,
-4.94389036502613));
#450325=CARTESIAN_POINT('Ctrl Pts',(-7.10715379447205,23.5638947104357,
-5.60787864620878));
#450326=CARTESIAN_POINT('Ctrl Pts',(-6.65070324968042,23.5007629897185,
-6.81352117024561));
#450327=CARTESIAN_POINT('Ctrl Pts',(-5.22331918686542,23.4292799190243,
-7.11892889768229));
#450328=CARTESIAN_POINT('Ctrl Pts',(-4.19313572939823,23.3577968483302,
-6.08480364614364));
#450329=CARTESIAN_POINT('Ctrl Pts',(-4.50398657889369,23.2863137776359,
-4.65859667867589));
#450330=CARTESIAN_POINT('Ctrl Pts',(-5.70962577012502,23.2232731885846,
-4.20740365817457));
#450331=CARTESIAN_POINT('Ctrl Pts',(-6.37096218895919,23.1840602897646,
-4.55115618731808));
#450332=CARTESIAN_POINT('Ctrl Pts',(-6.56867439792569,23.168675081176,-4.74631652959707));
#450333=CARTESIAN_POINT('Ctrl Pts',(-6.57003272085371,23.656324918824,-4.74532300381163));
#450334=CARTESIAN_POINT('Ctrl Pts',(-6.63539236159828,23.6512361682467,
-4.80948437015677));
#450335=CARTESIAN_POINT('Ctrl Pts',(-6.9668858368575,23.622319727438,-5.21266771861286));
#450336=CARTESIAN_POINT('Ctrl Pts',(-7.04564953674368,23.569575596398,-6.28682364983267));
#450337=CARTESIAN_POINT('Ctrl Pts',(-5.88000083782647,23.4980925257038,
-7.16543624640093));
#450338=CARTESIAN_POINT('Ctrl Pts',(-4.50990820099157,23.4266094550096,
-6.66190630419616));
#450339=CARTESIAN_POINT('Ctrl Pts',(-4.19063094092434,23.3551263843154,
-5.23756146736659));
#450340=CARTESIAN_POINT('Ctrl Pts',(-5.21468783779197,23.2836433136212,
-4.19736598356861));
#450341=CARTESIAN_POINT('Ctrl Pts',(-6.20635078283889,23.2340428251241,
-4.40342562281452));
#450342=CARTESIAN_POINT('Ctrl Pts',(-6.54530502316694,23.2082700268584,
-4.71817410701172));
#450343=CARTESIAN_POINT('Ctrl Pts',(-6.56983844394705,23.206324918824,-4.74299838399068));
#450344=CARTESIAN_POINT('Origin',(-5.65685387860012,26.993675081176,-5.65685387860011));
#450345=CARTESIAN_POINT('',(-6.56748881619374,24.106324918824,-4.74613115927677));
#450346=CARTESIAN_POINT('',(-6.57010232725217,24.068675081176,-4.74299681637215));
#450347=CARTESIAN_POINT('',(-6.56902162633079,26.993675081176,-4.74468613086949));
#450348=CARTESIAN_POINT('Ctrl Pts',(-6.57010232725218,24.068675081176,-4.74299681637215));
#450349=CARTESIAN_POINT('Ctrl Pts',(-6.85435514987614,24.0461648823099,
-5.02972694085412));
#450350=CARTESIAN_POINT('Ctrl Pts',(-7.14655186859909,23.9998269932124,
-5.91736950865738));
#450351=CARTESIAN_POINT('Ctrl Pts',(-6.27199288310558,23.9296614138836,
-7.0522818436793));
#450352=CARTESIAN_POINT('Ctrl Pts',(-4.81743049717126,23.8581783431894,
-6.93003241982605));
#450353=CARTESIAN_POINT('Ctrl Pts',(-4.13193628895796,23.7866952724952,
-5.64131435190337));
#450354=CARTESIAN_POINT('Ctrl Pts',(-4.84355050202496,23.715212201801,-4.3668333837381));
#450355=CARTESIAN_POINT('Ctrl Pts',(-5.98491025846012,23.6592054713613,
-4.29429575151248));
#450356=CARTESIAN_POINT('Ctrl Pts',(-6.4614899633887,23.627026431153,-4.63766432477859));
#450357=CARTESIAN_POINT('Ctrl Pts',(-6.56740434249263,23.618675081176,-4.74499326893249));
#450358=CARTESIAN_POINT('Ctrl Pts',(-6.56748881619374,24.106324918824,-4.74613115927677));
#450359=CARTESIAN_POINT('Ctrl Pts',(-6.72241589762581,24.0942023096351,
-4.90119115627847));
#450360=CARTESIAN_POINT('Ctrl Pts',(-7.07096798466868,24.0582520102147,
-5.47210261995127));
#450361=CARTESIAN_POINT('Ctrl Pts',(-6.80286792203874,23.998474020563,-6.662968703113));
#450362=CARTESIAN_POINT('Ctrl Pts',(-5.43230911237055,23.9269909498688,
-7.16522879152533));
#450363=CARTESIAN_POINT('Ctrl Pts',(-4.26747512907024,23.8555078791747,
-6.2855365564656));
#450364=CARTESIAN_POINT('Ctrl Pts',(-4.37557081254884,23.7840248084805,
-4.82985391579145));
#450365=CARTESIAN_POINT('Ctrl Pts',(-5.56629788826614,23.7176304883636,
-4.18154636230721));
#450366=CARTESIAN_POINT('Ctrl Pts',(-6.32935078034096,23.6750638584781,
-4.50905361827065));
#450367=CARTESIAN_POINT('Ctrl Pts',(-6.57003272085371,23.656324918824,-4.74532300381163));
#450368=CARTESIAN_POINT('Origin',(-5.65685387860012,26.993675081176,-5.65685387860011));
#450369=CARTESIAN_POINT('',(-6.56856700353347,24.556324918824,-4.74353459859835));
#450370=CARTESIAN_POINT('',(-6.56980231202958,24.518675081176,-4.74557835604531));
#450371=CARTESIAN_POINT('',(-6.56902162633079,26.993675081176,-4.74468613086949));
#450372=CARTESIAN_POINT('Ctrl Pts',(-6.56980231202958,24.518675081176,-4.74557835604531));
#450373=CARTESIAN_POINT('Ctrl Pts',(-6.64326578517921,24.5129587139297,
-4.81770944620421));
#450374=CARTESIAN_POINT('Ctrl Pts',(-6.97750833641272,24.4834146564519,
-5.23445549419879));
#450375=CARTESIAN_POINT('Ctrl Pts',(-7.02860988272989,24.4300429087428,
-6.32311258055821));
#450376=CARTESIAN_POINT('Ctrl Pts',(-5.84026841822957,24.3585598380486,
-7.17078066054311));
#450377=CARTESIAN_POINT('Ctrl Pts',(-4.4838850778304,24.2870767673545,-6.63140987332417));
#450378=CARTESIAN_POINT('Ctrl Pts',(-4.2021595986403,24.2155936966603,-5.19916430623342));
#450379=CARTESIAN_POINT('Ctrl Pts',(-5.25320498229437,24.1441106259661,
-4.18624762160045));
#450380=CARTESIAN_POINT('Ctrl Pts',(-6.22663461042285,24.095137754138,-4.41536649518845));
#450381=CARTESIAN_POINT('Ctrl Pts',(-6.55346539562853,24.0699925725413,
-4.72621489163553));
#450382=CARTESIAN_POINT('Ctrl Pts',(-6.57010232725218,24.068675081176,-4.74299681637215));
#450383=CARTESIAN_POINT('Ctrl Pts',(-6.56856700353346,24.556324918824,-4.74353459859835));
#450384=CARTESIAN_POINT('Ctrl Pts',(-6.81000592522228,24.5371684510234,
-4.98945253222269));
#450385=CARTESIAN_POINT('Ctrl Pts',(-7.13455935910424,24.4941842929915,
-5.76578134653658));
#450386=CARTESIAN_POINT('Ctrl Pts',(-6.46131966662841,24.4273724447281,
-6.95240396480877));
#450387=CARTESIAN_POINT('Ctrl Pts',(-5.00396921476326,24.3558893740339,
-7.03502543671246));
#450388=CARTESIAN_POINT('Ctrl Pts',(-4.14478270244581,24.2844063033397,
-5.85498510857852));
#450389=CARTESIAN_POINT('Ctrl Pts',(-4.67093497503137,24.2129232326456,
-4.49341967622111));
#450390=CARTESIAN_POINT('Ctrl Pts',(-5.85795834238072,24.1535627711403,
-4.24791389261248));
#450391=CARTESIAN_POINT('Ctrl Pts',(-6.41789774915756,24.1180299998665,
-4.5964117545626));
#450392=CARTESIAN_POINT('Ctrl Pts',(-6.56748881619374,24.106324918824,-4.74613115927677));
#450393=CARTESIAN_POINT('Origin',(-5.65685387860012,26.993675081176,-5.65685387860011));
#450394=CARTESIAN_POINT('',(-6.57067994464874,25.006324918824,-4.74405758279953));
#450395=CARTESIAN_POINT('',(-6.56738667375376,24.968675081176,-4.74597172529335));
#450396=CARTESIAN_POINT('',(-6.56902162633079,26.993675081176,-4.74468613086949));
#450397=CARTESIAN_POINT('Ctrl Pts',(-6.56738667375376,24.968675081176,-4.74597172529335));
#450398=CARTESIAN_POINT('Ctrl Pts',(-6.73011316031215,24.955924855318,-4.90925551921452));
#450399=CARTESIAN_POINT('Ctrl Pts',(-7.0784783223036,24.9193469392286,-5.49691387622178));
#450400=CARTESIAN_POINT('Ctrl Pts',(-6.77602463836695,24.8589413329079,
-6.69274573713214));
#450401=CARTESIAN_POINT('Ctrl Pts',(-5.39273679116276,24.7874582622137,
-7.15880506797054));
#450402=CARTESIAN_POINT('Ctrl Pts',(-4.25142935492228,24.7159751915195,
-6.24879737998679));
#450403=CARTESIAN_POINT('Ctrl Pts',(-4.39775252453572,24.6444921208253,
-4.79645922145989));
#450404=CARTESIAN_POINT('Ctrl Pts',(-5.59369688000734,24.5787254173775,
-4.18550614000559));
#450405=CARTESIAN_POINT('Ctrl Pts',(-6.33704597702196,24.5367864041611,
-4.51704344657683));
#450406=CARTESIAN_POINT('Ctrl Pts',(-6.56980231202958,24.518675081176,-4.74557835604531));
#450407=CARTESIAN_POINT('Ctrl Pts',(-6.57067994464874,25.006324918824,-4.74405758279953));
#450408=CARTESIAN_POINT('Ctrl Pts',(-6.60086819803687,25.0039622826432,
-4.77384081402403));
#450409=CARTESIAN_POINT('Ctrl Pts',(-6.91811250300101,24.9777719562309,
-5.12098437694123));
#450410=CARTESIAN_POINT('Ctrl Pts',(-7.10838527255516,24.9277539395874,
-6.12447699388038));
#450411=CARTESIAN_POINT('Ctrl Pts',(-6.05044038944422,24.8562708688931,
-7.13018513270865));
#450412=CARTESIAN_POINT('Ctrl Pts',(-4.63189669239788,24.784787798199,-6.78604742232836));
#450413=CARTESIAN_POINT('Ctrl Pts',(-4.15240479236239,24.7133047275048,
-5.40735816264999));
#450414=CARTESIAN_POINT('Ctrl Pts',(-5.0512683537124,24.6418216568106,-4.25725342975252));
#450415=CARTESIAN_POINT('Ctrl Pts',(-6.11539165852711,24.589495053917,-4.35401829743014));
#450416=CARTESIAN_POINT('Ctrl Pts',(-6.50969315902277,24.5609961412548,
-4.68356856625642));
#450417=CARTESIAN_POINT('Ctrl Pts',(-6.56856700353346,24.556324918824,-4.74353459859835));
#450418=CARTESIAN_POINT('Origin',(-5.65685387860012,26.993675081176,-5.65685387860011));
#450419=CARTESIAN_POINT('',(-6.56829321884323,25.456324918824,-4.74640124271564));
#450420=CARTESIAN_POINT('',(-6.56885365284802,25.418675081176,-4.74334636410459));
#450421=CARTESIAN_POINT('',(-6.56902162633079,26.993675081176,-4.74468613086949));
#450422=CARTESIAN_POINT('Ctrl Pts',(-6.56885365284802,25.418675081176,-4.74334636410459));
#450423=CARTESIAN_POINT('Ctrl Pts',(-6.81811011972481,25.3988909967064,
-4.99707565976646));
#450424=CARTESIAN_POINT('Ctrl Pts',(-7.13780202337966,25.3552792220053,
-5.79361205385018));
#450425=CARTESIAN_POINT('Ctrl Pts',(-6.42698533143036,25.287839757073,-6.97310209577086));
#450426=CARTESIAN_POINT('Ctrl Pts',(-4.96796792520408,25.2163566863788,
-7.01738753624157));
#450427=CARTESIAN_POINT('Ctrl Pts',(-4.14009680960707,25.1448736156846,
-5.81516935358236));
#450428=CARTESIAN_POINT('Ctrl Pts',(-4.70185841202445,25.0733905449904,
-4.46790543942481));
#450429=CARTESIAN_POINT('Ctrl Pts',(-5.88231068328694,25.0146577001542,
-4.25595199715398));
#450430=CARTESIAN_POINT('Ctrl Pts',(-6.4260090324839,24.9797525455494,-4.604109892408));
#450431=CARTESIAN_POINT('Ctrl Pts',(-6.56738667375376,24.968675081176,-4.74597172529335));
#450432=CARTESIAN_POINT('Ctrl Pts',(-6.56829321884323,25.456324918824,-4.74640124271564));
#450433=CARTESIAN_POINT('Ctrl Pts',(-6.68893848409318,25.4469284240315,
-4.86586022639608));
#450434=CARTESIAN_POINT('Ctrl Pts',(-7.03476003379299,25.4137042390077,
-5.36752678600608));
#450435=CARTESIAN_POINT('Ctrl Pts',(-6.9100356033464,25.3566523637524,-6.5258341885166));
#450436=CARTESIAN_POINT('Ctrl Pts',(-5.60564496305001,25.2851692930582,
-7.18099123031483));
#450437=CARTESIAN_POINT('Ctrl Pts',(-4.34815567114858,25.213686222364,-6.43975200870338));
#450438=CARTESIAN_POINT('Ctrl Pts',(-4.2896855842815,25.1422031516699,-4.98123363545819));
#450439=CARTESIAN_POINT('Ctrl Pts',(-5.44432497425889,25.0730827171565,
-4.16945626611646));
#450440=CARTESIAN_POINT('Ctrl Pts',(-6.29641321838457,25.0277899728745,
-4.47347056935133));
#450441=CARTESIAN_POINT('Ctrl Pts',(-6.57067994464874,25.006324918824,-4.74405758279953));
#450442=CARTESIAN_POINT('Origin',(-5.65685387860012,26.993675081176,-5.65685387860011));
#450443=CARTESIAN_POINT('',(-6.56704169373441,25.906324918824,-4.74450601134849));
#450444=CARTESIAN_POINT('',(-6.57057130100612,25.868675081176,-4.74432962138981));
#450445=CARTESIAN_POINT('',(-6.56902162633079,26.993675081176,-4.74468613086949));
#450446=CARTESIAN_POINT('',(-5.01302286563433,26.,-4.53900700771688));
#450447=CARTESIAN_POINT('Ctrl Pts',(-5.01302286563431,26.,-4.53900700771688));
#450448=CARTESIAN_POINT('Ctrl Pts',(-5.38492752167559,25.9761723097686,
-4.32480615636363));
#450449=CARTESIAN_POINT('Ctrl Pts',(-6.01924597306242,25.9449472827099,
-4.30899334914827));
#450450=CARTESIAN_POINT('Ctrl Pts',(-6.47338425157137,25.9137222556513,
-4.64940368207851));
#450451=CARTESIAN_POINT('Ctrl Pts',(-6.56704169373441,25.906324918824,-4.74450601134849));
#450452=CARTESIAN_POINT('',(-4.53689596693371,26.,-5.01208503488091));
#450453=CARTESIAN_POINT('Origin',(-5.65685387860012,26.,-5.65685387860011));
#450454=CARTESIAN_POINT('Ctrl Pts',(-4.5368902045627,26.,-5.01208247494518));
#450455=CARTESIAN_POINT('Ctrl Pts',(-4.74314812622022,25.9770624644402,
-4.65613984562121));
#450456=CARTESIAN_POINT('Ctrl Pts',(-5.48969900651177,25.9332874914989,
-4.17795197796789));
#450457=CARTESIAN_POINT('Ctrl Pts',(-6.3039677816093,25.8895125185575,-4.48184576512937));
#450458=CARTESIAN_POINT('Ctrl Pts',(-6.57057130100612,25.868675081176,-4.74432962138981));
#450459=CARTESIAN_POINT('Origin',(-5.65685387860011,26.,5.65685387860011));
#450460=CARTESIAN_POINT('',(-4.9222125558517,22.573038475773,6.39190072013885));
#450461=CARTESIAN_POINT('',(-4.92305381642377,22.5,6.39065394077645));
#450462=CARTESIAN_POINT('',(-4.92305381642377,26.,6.39065394077645));
#450463=CARTESIAN_POINT('',(-5.8978925564917,22.5,6.66622270032004));
#450464=CARTESIAN_POINT('Origin',(-5.65685387860011,22.5,5.65685387860011));
#450465=CARTESIAN_POINT('Ctrl Pts',(-5.89851203167784,22.5,6.66798006829997));
#450466=CARTESIAN_POINT('Ctrl Pts',(-5.57641995134461,22.5229375355598,
6.7439998684947));
#450467=CARTESIAN_POINT('Ctrl Pts',(-5.21379162224851,22.5458750711197,
6.65366449057419));
#450468=CARTESIAN_POINT('Ctrl Pts',(-4.96646199655034,22.5688126066795,
6.43383171727969));
#450469=CARTESIAN_POINT('Ctrl Pts',(-4.95127317183385,22.5702212297106,
6.42033150900062));
#450470=CARTESIAN_POINT('Ctrl Pts',(-4.93651917810251,22.5716298527418,
6.40634292159547));
#450471=CARTESIAN_POINT('Ctrl Pts',(-4.9222125558517,22.573038475773,6.39190072013885));
#450472=CARTESIAN_POINT('Origin',(-5.65685387860011,26.,5.65685387860011));
#450473=CARTESIAN_POINT('',(-4.92436540268704,23.0230384757729,6.39037461032892));
#450474=CARTESIAN_POINT('',(-4.92349966353597,22.9019615242271,6.38930388760559));
#450475=CARTESIAN_POINT('',(-4.92305381642377,26.,6.39065394077645));
#450476=CARTESIAN_POINT('',(-4.62591736201901,22.5,5.77557608073439));
#450477=CARTESIAN_POINT('Ctrl Pts',(-4.92349966353597,22.9019615242271,
6.38930388760559));
#450478=CARTESIAN_POINT('Ctrl Pts',(-5.07692511110986,22.8871128006417,
6.54102880287524));
#450479=CARTESIAN_POINT('Ctrl Pts',(-5.27640120658105,22.8722640770563,
6.64766299899898));
#450480=CARTESIAN_POINT('Ctrl Pts',(-5.48772889025785,22.8574153534709,
6.68249361011691));
#450481=CARTESIAN_POINT('Ctrl Pts',(-5.82684562005692,22.8335876632395,
6.73838615923167));
#450482=CARTESIAN_POINT('Ctrl Pts',(-6.19648078060475,22.8097599730081,
6.60938089562333));
#450483=CARTESIAN_POINT('Ctrl Pts',(-6.42720821100082,22.7859322827767,
6.35472685290066));
#450484=CARTESIAN_POINT('Ctrl Pts',(-6.65793564139689,22.7621045925453,
6.10007281017799));
#450485=CARTESIAN_POINT('Ctrl Pts',(-6.74975534164119,22.7382769023139,
5.71976998834099));
#450486=CARTESIAN_POINT('Ctrl Pts',(-6.66080060824128,22.7144492120825,
5.38773213421059));
#450487=CARTESIAN_POINT('Ctrl Pts',(-6.57184587484137,22.6906215218511,
5.05569428008018));
#450488=CARTESIAN_POINT('Ctrl Pts',(-6.30211670779724,22.6667938316197,
4.77192139365638));
#450489=CARTESIAN_POINT('Ctrl Pts',(-5.97477550103877,22.6429661413884,
4.66700870222797));
#450490=CARTESIAN_POINT('Ctrl Pts',(-5.6474342942803,22.619138451157,4.56209601079956));
#450491=CARTESIAN_POINT('Ctrl Pts',(-5.26248104780748,22.5953107609256,
4.63604351436656));
#450492=CARTESIAN_POINT('Ctrl Pts',(-4.99722717517853,22.5714830706942,
4.85366607828882));
#450493=CARTESIAN_POINT('Ctrl Pts',(-4.73197330254959,22.5476553804628,
5.07128864221107));
#450494=CARTESIAN_POINT('Ctrl Pts',(-4.58641880376449,22.5238276902314,
5.43258626648858));
#450495=CARTESIAN_POINT('Ctrl Pts',(-4.625917362019,22.5,5.77557608073438));
#450496=CARTESIAN_POINT('Origin',(-5.65685387860011,22.5,5.65685387860011));
#450497=CARTESIAN_POINT('Ctrl Pts',(-4.9222125558517,22.573038475773,6.39190072013885));
#450498=CARTESIAN_POINT('Ctrl Pts',(-4.69451421601594,22.5954575429732,
6.16204455719575));
#450499=CARTESIAN_POINT('Ctrl Pts',(-4.58013776446743,22.6178766101734,
5.81728522517979));
#450500=CARTESIAN_POINT('Ctrl Pts',(-4.62964039434809,22.6402956773736,
5.49777863793003));
#450501=CARTESIAN_POINT('Ctrl Pts',(-4.68225334741615,22.664123367605,5.15819698094666));
#450502=CARTESIAN_POINT('Ctrl Pts',(-4.91998587117151,22.6879510578364,
4.84714109570319));
#450503=CARTESIAN_POINT('Ctrl Pts',(-5.23393572436938,22.7117787480678,
4.70728537400252));
#450504=CARTESIAN_POINT('Ctrl Pts',(-5.54788557756724,22.7356064382992,
4.56742965230184));
#450505=CARTESIAN_POINT('Ctrl Pts',(-5.93805276020761,22.7594341285306,
4.59877409414395));
#450506=CARTESIAN_POINT('Ctrl Pts',(-6.22570363532513,22.783261818762,4.78686738296995));
#450507=CARTESIAN_POINT('Ctrl Pts',(-6.51335451044265,22.8070895089934,
4.97496067179595));
#450508=CARTESIAN_POINT('Ctrl Pts',(-6.69848907803731,22.8309171992248,
5.31980280760584));
#450509=CARTESIAN_POINT('Ctrl Pts',(-6.69629884619592,22.8547448894562,
5.66347121722023));
#450510=CARTESIAN_POINT('Ctrl Pts',(-6.69410861435454,22.8785725796876,
6.00713962683461));
#450511=CARTESIAN_POINT('Ctrl Pts',(-6.5045935830771,22.902400269919,6.34963431025349));
#450512=CARTESIAN_POINT('Ctrl Pts',(-6.21456908983246,22.9262279601503,
6.53403672593788));
#450513=CARTESIAN_POINT('Ctrl Pts',(-5.92454459658782,22.9500556503817,
6.71843914162228));
#450514=CARTESIAN_POINT('Ctrl Pts',(-5.53401064137597,22.9738833406131,
6.7447492895722));
#450515=CARTESIAN_POINT('Ctrl Pts',(-5.22186823831327,22.9977110308445,
6.60092695407667));
#450516=CARTESIAN_POINT('Ctrl Pts',(-5.11127184889382,23.0061535124873,
6.54996870275417));
#450517=CARTESIAN_POINT('Ctrl Pts',(-5.01051660428821,23.0145959941301,
6.47765230299322));
#450518=CARTESIAN_POINT('Ctrl Pts',(-4.92436540268704,23.0230384757729,
6.39037461032892));
#450519=CARTESIAN_POINT('Origin',(-5.65685387860011,26.,5.65685387860011));
#450520=CARTESIAN_POINT('',(-4.92330089590042,23.4730384757729,6.38935290488262));
#450521=CARTESIAN_POINT('',(-4.92169609601798,23.3519615242271,6.39131103572319));
#450522=CARTESIAN_POINT('',(-4.92305381642377,26.,6.39065394077645));
#450523=CARTESIAN_POINT('Ctrl Pts',(-4.92169609601798,23.3519615242271,
6.39131103572319));
#450524=CARTESIAN_POINT('Ctrl Pts',(-5.14636061012976,23.33007894203,6.61334324490838));
#450525=CARTESIAN_POINT('Ctrl Pts',(-5.47994522249351,23.308196359833,6.72868171719176));
#450526=CARTESIAN_POINT('Ctrl Pts',(-5.79285848911254,23.286313777636,6.68738448495221));
#450527=CARTESIAN_POINT('Ctrl Pts',(-6.13358611984441,23.2624860874046,
6.64241640721998));
#450528=CARTESIAN_POINT('Ctrl Pts',(-6.44980419113038,23.2386583971732,
6.41172882390928));
#450529=CARTESIAN_POINT('Ctrl Pts',(-6.59665364733223,23.2148307069418,
6.10100080909856));
#450530=CARTESIAN_POINT('Ctrl Pts',(-6.74350310353408,23.1910030167104,
5.79027279428784));
#450531=CARTESIAN_POINT('Ctrl Pts',(-6.7209839446518,23.167175326479,5.39950434797711));
#450532=CARTESIAN_POINT('Ctrl Pts',(-6.539415444341,23.1433476362476,5.1076985472349));
#450533=CARTESIAN_POINT('Ctrl Pts',(-6.3578469440302,23.1195199460162,4.8158927464927));
#450534=CARTESIAN_POINT('Ctrl Pts',(-6.01722910229088,23.0956922557848,
4.62304959131903));
#450535=CARTESIAN_POINT('Ctrl Pts',(-5.67358993507176,23.0718645655534,
4.61751951301592));
#450536=CARTESIAN_POINT('Ctrl Pts',(-5.32995076785264,23.048036875322,4.61198943471281));
#450537=CARTESIAN_POINT('Ctrl Pts',(-4.98329027515371,23.0242091850907,
4.79377243328025));
#450538=CARTESIAN_POINT('Ctrl Pts',(-4.7924243254548,23.0003814948593,5.07957475014376));
#450539=CARTESIAN_POINT('Ctrl Pts',(-4.60155837575589,22.9765538046279,
5.36537706700727));
#450540=CARTESIAN_POINT('Ctrl Pts',(-4.566486969057,22.9527261143965,5.75519870216683));
#450541=CARTESIAN_POINT('Ctrl Pts',(-4.70325041523272,22.9288984241651,
6.07050470066555));
#450542=CARTESIAN_POINT('Ctrl Pts',(-4.75478685916324,22.9199194575191,
6.18932117076025));
#450543=CARTESIAN_POINT('Ctrl Pts',(-4.83072387924101,22.9109404908731,
6.29755640872372));
#450544=CARTESIAN_POINT('Ctrl Pts',(-4.92349966353597,22.9019615242271,
6.38930388760559));
#450545=CARTESIAN_POINT('Ctrl Pts',(-4.92436540268704,23.0230384757729,
6.39037461032892));
#450546=CARTESIAN_POINT('Ctrl Pts',(-4.76736722811336,23.0384236843615,
6.23132356780567));
#450547=CARTESIAN_POINT('Ctrl Pts',(-4.65886881811934,23.0538088929501,
6.02258634020352));
#450548=CARTESIAN_POINT('Ctrl Pts',(-4.62769529041208,23.0691941015387,
5.80287677492702));
#450549=CARTESIAN_POINT('Ctrl Pts',(-4.57941559648715,23.0930217917701,
5.46260375021388));
#450550=CARTESIAN_POINT('Ctrl Pts',(-4.71660705955086,23.1168494820015,
5.09601251972856));
#450551=CARTESIAN_POINT('Ctrl Pts',(-4.97642324075838,23.1406771722329,
4.87103919530453));
#450552=CARTESIAN_POINT('Ctrl Pts',(-5.2362394219659,23.1645048624643,4.64606587088049));
#450553=CARTESIAN_POINT('Ctrl Pts',(-5.61868032131723,23.1883325526957,
4.56271045251773));
#450554=CARTESIAN_POINT('Ctrl Pts',(-5.94855238336812,23.2121602429271,
4.65915585483332));
#450555=CARTESIAN_POINT('Ctrl Pts',(-6.278424445419,23.2359879331585,4.75560125714891));
#450556=CARTESIAN_POINT('Ctrl Pts',(-6.55572767016945,23.2598156233899,
5.03184748014285));
#450557=CARTESIAN_POINT('Ctrl Pts',(-6.65343136663416,23.2836433136212,
5.36134886181892));
#450558=CARTESIAN_POINT('Ctrl Pts',(-6.75113506309886,23.3074710038526,
5.690850243495));
#450559=CARTESIAN_POINT('Ctrl Pts',(-6.66923923127783,23.331298694084,6.07360678385322));
#450560=CARTESIAN_POINT('Ctrl Pts',(-6.44525978436571,23.3551263843154,
6.33427992409048));
#450561=CARTESIAN_POINT('Ctrl Pts',(-6.22128033745359,23.3789540745468,
6.59495306432775));
#450562=CARTESIAN_POINT('Ctrl Pts',(-5.85521727545038,23.4027817647782,
6.73354280444407));
#450563=CARTESIAN_POINT('Ctrl Pts',(-5.51476156795534,23.4266094550096,
6.6865623548039));
#450564=CARTESIAN_POINT('Ctrl Pts',(-5.29363193601897,23.442085795264,6.65604804910002));
#450565=CARTESIAN_POINT('Ctrl Pts',(-5.08330512959901,23.4575621355185,
6.54724832815155));
#450566=CARTESIAN_POINT('Ctrl Pts',(-4.92330089590042,23.4730384757729,
6.38935290488262));
#450567=CARTESIAN_POINT('Origin',(-5.65685387860011,26.,5.65685387860011));
#450568=CARTESIAN_POINT('',(-4.92169483493571,23.9230384757729,6.39152331859132));
#450569=CARTESIAN_POINT('',(-4.92356615355223,23.8019615242271,6.39146732321148));
#450570=CARTESIAN_POINT('',(-4.92305381642377,26.,6.39065394077645));
#450571=CARTESIAN_POINT('Ctrl Pts',(-4.92356615355223,23.8019615242271,
6.39146732321148));
#450572=CARTESIAN_POINT('Ctrl Pts',(-4.97518123721477,23.7968727736498,
6.44404636753914));
#450573=CARTESIAN_POINT('Ctrl Pts',(-5.03225965778749,23.7917840230725,
6.49097569651667));
#450574=CARTESIAN_POINT('Ctrl Pts',(-5.09396482100832,23.7866952724952,
6.53072214720976));
#450575=CARTESIAN_POINT('Ctrl Pts',(-5.38289458727869,23.7628675822638,
6.71683190058211));
#450576=CARTESIAN_POINT('Ctrl Pts',(-5.77326614382955,23.7390398920324,
6.74545633697037));
#450577=CARTESIAN_POINT('Ctrl Pts',(-6.08625298439034,23.715212201801,6.60348277515141));
#450578=CARTESIAN_POINT('Ctrl Pts',(-6.39923982495114,23.6913845115696,
6.46150921333244));
#450579=CARTESIAN_POINT('Ctrl Pts',(-6.63484194952187,23.6675568213382,
6.14893765330626));
#450580=CARTESIAN_POINT('Ctrl Pts',(-6.68513161677842,23.6437291311068,
5.80895502137128));
#450581=CARTESIAN_POINT('Ctrl Pts',(-6.73542128403497,23.6199014408755,
5.4689723894363));
#450582=CARTESIAN_POINT('Ctrl Pts',(-6.60039849397735,23.5960737506441,
5.10157868559252));
#450583=CARTESIAN_POINT('Ctrl Pts',(-6.34191631672375,23.5722460604127,
4.87507434314934));
#450584=CARTESIAN_POINT('Ctrl Pts',(-6.08343413947014,23.5484183701813,
4.64857000070617));
#450585=CARTESIAN_POINT('Ctrl Pts',(-5.70149257502055,23.5245906799499,
4.56295501966359));
#450586=CARTESIAN_POINT('Ctrl Pts',(-5.37105630657982,23.5007629897185,
4.65744921450721));
#450587=CARTESIAN_POINT('Ctrl Pts',(-5.04062003813909,23.4769352994871,
4.75194340935083));
#450588=CARTESIAN_POINT('Ctrl Pts',(-4.76168906570723,23.4531076092557,
5.02654678008064));
#450589=CARTESIAN_POINT('Ctrl Pts',(-4.66203997694959,23.4292799190243,
5.35546505814245));
#450590=CARTESIAN_POINT('Ctrl Pts',(-4.56239088819196,23.4054522287929,
5.68438333620426));
#450591=CARTESIAN_POINT('Ctrl Pts',(-4.64202368310855,23.3816245385615,
6.06761652159808));
#450592=CARTESIAN_POINT('Ctrl Pts',(-4.86445867565572,23.3577968483301,
6.32960882821811));
#450593=CARTESIAN_POINT('Ctrl Pts',(-4.88261654521522,23.3558517402958,
6.350995850443));
#450594=CARTESIAN_POINT('Ctrl Pts',(-4.90172602358781,23.3539066322614,
6.37157494470415));
#450595=CARTESIAN_POINT('Ctrl Pts',(-4.92169609601798,23.3519615242271,
6.39131103572319));
#450596=CARTESIAN_POINT('Ctrl Pts',(-4.92330089590042,23.4730384757729,
6.38935290488262));
#450597=CARTESIAN_POINT('Ctrl Pts',(-4.83695933636888,23.4813898257499,
6.30414930262285));
#450598=CARTESIAN_POINT('Ctrl Pts',(-4.76527121936352,23.4897411757268,
6.20464951053553));
#450599=CARTESIAN_POINT('Ctrl Pts',(-4.71444637045848,23.4980925257038,
6.09544017298549));
#450600=CARTESIAN_POINT('Ctrl Pts',(-4.56943523344352,23.5219202159352,
5.78384908020389));
#450601=CARTESIAN_POINT('Ctrl Pts',(-4.59426131240048,23.5457479061666,
5.39321753403733));
#450602=CARTESIAN_POINT('Ctrl Pts',(-4.77755195197114,23.569575596398,5.10249121190879));
#450603=CARTESIAN_POINT('Ctrl Pts',(-4.9608425915418,23.5934032866293,4.81176488978025));
#450604=CARTESIAN_POINT('Ctrl Pts',(-5.30259779172617,23.6172309768607,
4.62094379168974));
#450605=CARTESIAN_POINT('Ctrl Pts',(-5.64626184853499,23.6410586670921,
4.61744171997954));
#450606=CARTESIAN_POINT('Ctrl Pts',(-5.98992590534381,23.6648863573235,
4.61393964826934));
#450607=CARTESIAN_POINT('Ctrl Pts',(-6.33549881877709,23.6887140475549,
4.79775660293946));
#450608=CARTESIAN_POINT('Ctrl Pts',(-6.52467601704459,23.7125417377863,
5.08468731748426));
#450609=CARTESIAN_POINT('Ctrl Pts',(-6.71385321531209,23.7363694280177,
5.37161803202905));
#450610=CARTESIAN_POINT('Ctrl Pts',(-6.74663469841383,23.7601971182491,
5.76166250644851));
#450611=CARTESIAN_POINT('Ctrl Pts',(-6.60800349462427,23.7840248084805,
6.07614404554655));
#450612=CARTESIAN_POINT('Ctrl Pts',(-6.46937229083472,23.8078524987119,
6.39062558464459));
#450613=CARTESIAN_POINT('Ctrl Pts',(-6.15932840015388,23.8316801889433,
6.6295441884212));
#450614=CARTESIAN_POINT('Ctrl Pts',(-5.81990079386588,23.8555078791747,
6.6834528935629));
#450615=CARTESIAN_POINT('Ctrl Pts',(-5.49924097144978,23.8780180780408,
6.73438085433327));
#450616=CARTESIAN_POINT('Ctrl Pts',(-5.15235699515366,23.9005282769068,
6.62019259508592));
#450617=CARTESIAN_POINT('Ctrl Pts',(-4.92169483493571,23.9230384757729,
6.39152331859132));
#450618=CARTESIAN_POINT('Origin',(-5.65685387860011,26.,5.65685387860011));
#450619=CARTESIAN_POINT('',(-4.92377157353716,24.3730384757729,6.39128196913613));
#450620=CARTESIAN_POINT('',(-4.92421628016771,24.2519615242271,6.38942086037359));
#450621=CARTESIAN_POINT('',(-4.92305381642377,26.,6.39065394077645));
#450622=CARTESIAN_POINT('Ctrl Pts',(-4.92421628016771,24.2519615242271,
6.38942086037359));
#450623=CARTESIAN_POINT('Ctrl Pts',(-5.04895543667043,24.2398389150381,
6.51405309196749));
#450624=CARTESIAN_POINT('Ctrl Pts',(-5.20382475542584,24.2277163058492,
6.60860369693141));
#450625=CARTESIAN_POINT('Ctrl Pts',(-5.37198243345446,24.2155936966603,
6.65652287894995));
#450626=CARTESIAN_POINT('Ctrl Pts',(-5.70250608555364,24.1917660064289,
6.75071080561528));
#450627=CARTESIAN_POINT('Ctrl Pts',(-6.08436822205294,24.1679383161975,
6.66474206054895));
#450628=CARTESIAN_POINT('Ctrl Pts',(-6.34264042812557,24.1441106259661,
6.4379983333991));
#450629=CARTESIAN_POINT('Ctrl Pts',(-6.60091263419821,24.1202829357347,
6.21125460624925));
#450630=CARTESIAN_POINT('Ctrl Pts',(-6.73559490984418,24.0964552455033,
5.84373589701588));
#450631=CARTESIAN_POINT('Ctrl Pts',(-6.68499023152592,24.0726275552719,
5.50379999638241));
#450632=CARTESIAN_POINT('Ctrl Pts',(-6.63438555320766,24.0487998650405,
5.16386409574894));
#450633=CARTESIAN_POINT('Ctrl Pts',(-6.39849392092517,24.0249721748091,
4.85151100371537));
#450634=CARTESIAN_POINT('Ctrl Pts',(-6.08537566804496,24.0011444845777,
4.70982751913656));
#450635=CARTESIAN_POINT('Ctrl Pts',(-5.77225741516475,23.9773167943463,
4.56814403455774));
#450636=CARTESIAN_POINT('Ctrl Pts',(-5.38191254168682,23.953489104115,4.59713015743369));
#450637=CARTESIAN_POINT('Ctrl Pts',(-5.09315534403941,23.9296614138836,
4.78350754767415));
#450638=CARTESIAN_POINT('Ctrl Pts',(-4.804398146392,23.9058337236522,4.96988493791459));
#450639=CARTESIAN_POINT('Ctrl Pts',(-4.61722862457511,23.8820060334208,
5.31365359551954));
#450640=CARTESIAN_POINT('Ctrl Pts',(-4.6173878516616,23.8581783431894,5.65733545950024));
#450641=CARTESIAN_POINT('Ctrl Pts',(-4.61751307348277,23.8394394035353,
5.92761905169082));
#450642=CARTESIAN_POINT('Ctrl Pts',(-4.73349750638545,23.8207004638812,
6.19784896370208));
#450643=CARTESIAN_POINT('Ctrl Pts',(-4.92356615355223,23.8019615242271,
6.39146732321148));
#450644=CARTESIAN_POINT('Ctrl Pts',(-4.92169483493571,23.9230384757729,
6.39152331859132));
#450645=CARTESIAN_POINT('Ctrl Pts',(-4.90819449199352,23.9243559671382,
6.37813961642664));
#450646=CARTESIAN_POINT('Ctrl Pts',(-4.895092278726,23.9256734585035,6.3643637478711));
#450647=CARTESIAN_POINT('Ctrl Pts',(-4.88241675495565,23.9269909498688,
6.35020586507153));
#450648=CARTESIAN_POINT('Ctrl Pts',(-4.65317164422858,23.9508186401002,
6.09415132493169));
#450649=CARTESIAN_POINT('Ctrl Pts',(-4.56349274466962,23.9746463303316,
5.71314343814525));
#450650=CARTESIAN_POINT('Ctrl Pts',(-4.6544613426263,23.998474020563,5.38171929489583));
#450651=CARTESIAN_POINT('Ctrl Pts',(-4.74542994058297,24.0223017107944,
5.05029515164641));
#450652=CARTESIAN_POINT('Ctrl Pts',(-5.01704603605528,24.0461294010258,
4.768454751934));
#450653=CARTESIAN_POINT('Ctrl Pts',(-5.34488416612327,24.0699570912572,
4.6653072414873));
#450654=CARTESIAN_POINT('Ctrl Pts',(-5.67272229619127,24.0937847814886,
4.56215973104059));
#450655=CARTESIAN_POINT('Ctrl Pts',(-6.05678246085496,24.11761247172,4.63770510985958));
#450656=CARTESIAN_POINT('Ctrl Pts',(-6.32112934350159,24.1414401619514,
4.8573365604447));
#450657=CARTESIAN_POINT('Ctrl Pts',(-6.58547622614821,24.1652678521828,
5.07696801102981));
#450658=CARTESIAN_POINT('Ctrl Pts',(-6.73010982677778,24.1890955424141,
5.44068553338104));
#450659=CARTESIAN_POINT('Ctrl Pts',(-6.68877448884912,24.2129232326455,
5.78187263496817));
#450660=CARTESIAN_POINT('Ctrl Pts',(-6.64743915092045,24.2367509228769,
6.12305973655531));
#450661=CARTESIAN_POINT('Ctrl Pts',(-6.42013487443355,24.2605786131083,
6.44171641737836));
#450662=CARTESIAN_POINT('Ctrl Pts',(-6.11098818332588,24.2844063033397,
6.59186824658804));
#450663=CARTESIAN_POINT('Ctrl Pts',(-5.80184149221821,24.3082339935711,
6.74202007579772));
#450664=CARTESIAN_POINT('Ctrl Pts',(-5.41085238648978,24.3320616838025,
6.72366705339403));
#450665=CARTESIAN_POINT('Ctrl Pts',(-5.11713028264445,24.3558893740339,
6.54521657215205));
#450666=CARTESIAN_POINT('Ctrl Pts',(-5.04666506349635,24.3616057412803,
6.50240552012982));
#450667=CARTESIAN_POINT('Ctrl Pts',(-4.98179796021343,24.3673221085266,
6.45038020112141));
#450668=CARTESIAN_POINT('Ctrl Pts',(-4.92377157353716,24.3730384757729,
6.39128196913613));
#450669=CARTESIAN_POINT('Origin',(-5.65685387860011,26.,5.65685387860011));
#450670=CARTESIAN_POINT('',(-4.92408802232565,24.8230384757729,6.38933869113556));
#450671=CARTESIAN_POINT('',(-4.92212745780799,24.7019615242271,6.39028821611916));
#450672=CARTESIAN_POINT('',(-4.92305381642377,26.,6.39065394077645));
#450673=CARTESIAN_POINT('Ctrl Pts',(-4.92212745780799,24.7019615242271,
6.39028821611916));
#450674=CARTESIAN_POINT('Ctrl Pts',(-5.11995795053564,24.6828050564265,
6.5845155347103));
#450675=CARTESIAN_POINT('Ctrl Pts',(-5.39828521249021,24.6636485886259,
6.70087353526984));
#450676=CARTESIAN_POINT('Ctrl Pts',(-5.67455106061111,24.6444921208253,
6.69616935490973));
#450677=CARTESIAN_POINT('Ctrl Pts',(-6.01818314973456,24.620664430594,6.69031808036474));
#450678=CARTESIAN_POINT('Ctrl Pts',(-6.35862591802898,24.5968367403626,
6.49716519325233));
#450679=CARTESIAN_POINT('Ctrl Pts',(-6.53992487743046,24.5730090501312,
6.20519269912468));
#450680=CARTESIAN_POINT('Ctrl Pts',(-6.72122383683194,24.5491813598998,
5.91322020499702));
#450681=CARTESIAN_POINT('Ctrl Pts',(-6.74337898734048,24.5253536696684,
5.52242810385412));
#450682=CARTESIAN_POINT('Ctrl Pts',(-6.59624120723028,24.501525979437,5.21183556708661));
#450683=CARTESIAN_POINT('Ctrl Pts',(-6.44910342712008,24.4776982892056,
4.9012430303191));
#450684=CARTESIAN_POINT('Ctrl Pts',(-6.13267271639113,24.4538705989742,
4.670850057927));
#450685=CARTESIAN_POINT('Ctrl Pts',(-5.7919038045113,24.4300429087428,4.62619808347199));
#450686=CARTESIAN_POINT('Ctrl Pts',(-5.45113489263147,24.4062152185114,
4.58154610901698));
#450687=CARTESIAN_POINT('Ctrl Pts',(-5.08602777960075,24.38238752828,4.72263513249907));
#450688=CARTESIAN_POINT('Ctrl Pts',(-4.86383551964991,24.3585598380486,
4.98483324415836));
#450689=CARTESIAN_POINT('Ctrl Pts',(-4.64164325969907,24.3347321478172,
5.24703135581765));
#450690=CARTESIAN_POINT('Ctrl Pts',(-4.56236585282811,24.3109044575858,
5.63033855565415));
#450691=CARTESIAN_POINT('Ctrl Pts',(-4.66231973324216,24.2870767673544,
5.9591644547709));
#450692=CARTESIAN_POINT('Ctrl Pts',(-4.71142093690032,24.275371686312,6.12069642705376));
#450693=CARTESIAN_POINT('Ctrl Pts',(-4.80377340246064,24.2636666052695,
6.26908122485669));
#450694=CARTESIAN_POINT('Ctrl Pts',(-4.92421628016771,24.2519615242271,
6.38942086037359));
#450695=CARTESIAN_POINT('Ctrl Pts',(-4.92377157353716,24.3730384757729,
6.39128196913613));
#450696=CARTESIAN_POINT('Ctrl Pts',(-4.7399249826062,24.391149798758,6.20403942134221));
#450697=CARTESIAN_POINT('Ctrl Pts',(-4.62474754709557,24.4092611217431,
5.94579686164739));
#450698=CARTESIAN_POINT('Ctrl Pts',(-4.61775970678068,24.4273724447281,
5.68465923264326));
#450699=CARTESIAN_POINT('Ctrl Pts',(-4.60856633672445,24.4512001349595,
5.34110031445673));
#450700=CARTESIAN_POINT('Ctrl Pts',(-4.7866346985742,24.4750278251909,4.99253041816395));
#450701=CARTESIAN_POINT('Ctrl Pts',(-5.07039290068915,24.4988555154223,
4.79862701145602));
#450702=CARTESIAN_POINT('Ctrl Pts',(-5.35415110280411,24.5226832056536,
4.60472360474809));
#450703=CARTESIAN_POINT('Ctrl Pts',(-5.7435991451843,24.546510895885,4.565486687625));
#450704=CARTESIAN_POINT('Ctrl Pts',(-6.06033356407531,24.5703385861164,
4.69889042440694));
#450705=CARTESIAN_POINT('Ctrl Pts',(-6.37706798296632,24.5941662763478,
4.83229416118888));
#450706=CARTESIAN_POINT('Ctrl Pts',(-6.62108877836816,24.6179939665792,
5.13833855187584));
#450707=CARTESIAN_POINT('Ctrl Pts',(-6.68061169925028,24.6418216568106,
5.47682676316715));
#450708=CARTESIAN_POINT('Ctrl Pts',(-6.74013462013239,24.665649347042,5.81531497445846));
#450709=CARTESIAN_POINT('Ctrl Pts',(-6.61515966649478,24.6894770372734,
6.18624700635411));
#450710=CARTESIAN_POINT('Ctrl Pts',(-6.36293701391879,24.7133047275048,
6.41970146010492));
#450711=CARTESIAN_POINT('Ctrl Pts',(-6.1107143613428,24.7371324177362,6.65315591385573));
#450712=CARTESIAN_POINT('Ctrl Pts',(-5.73124400982843,24.7609601079676,
6.7491327894617));
#450713=CARTESIAN_POINT('Ctrl Pts',(-5.3983586947443,24.784787798199,6.6636657201663));
#450714=CARTESIAN_POINT('Ctrl Pts',(-5.22023136007979,24.797538024057,6.61793218802977));
#450715=CARTESIAN_POINT('Ctrl Pts',(-5.05544287282308,24.8102882499149,
6.5202452116208));
#450716=CARTESIAN_POINT('Ctrl Pts',(-4.92408802232565,24.8230384757729,
6.38933869113556));
#450717=CARTESIAN_POINT('Origin',(-5.65685387860011,26.,5.65685387860011));
#450718=CARTESIAN_POINT('',(-4.92197603118329,25.2730384757729,6.39051881327128));
#450719=CARTESIAN_POINT('',(-4.92254817630007,25.1519615242271,6.39198798715976));
#450720=CARTESIAN_POINT('',(-4.92305381642377,26.,6.39065394077645));
#450721=CARTESIAN_POINT('Ctrl Pts',(-4.92254817630007,25.1519615242271,
6.39198798715976));
#450722=CARTESIAN_POINT('Ctrl Pts',(-4.94650751599249,25.1495988880462,
6.41627314991443));
#450723=CARTESIAN_POINT('Ctrl Pts',(-4.97169983154625,25.1472362518654,
6.43929566708609));
#450724=CARTESIAN_POINT('Ctrl Pts',(-4.99805942366946,25.1448736156846,
6.46089355482011));
#450725=CARTESIAN_POINT('Ctrl Pts',(-5.26390153716754,25.1210459254532,
6.67871286308055));
#450726=CARTESIAN_POINT('Ctrl Pts',(-5.64846913729549,25.0972182352218,
6.75163093056004));
#450727=CARTESIAN_POINT('Ctrl Pts',(-5.97559449046916,25.0733905449904,
6.64624470558553));
#450728=CARTESIAN_POINT('Ctrl Pts',(-6.30271984364283,25.049562854759,6.54085848061101));
#450729=CARTESIAN_POINT('Ctrl Pts',(-6.57240294986222,25.0257351645276,
6.25716796318249));
#450730=CARTESIAN_POINT('Ctrl Pts',(-6.66110381706144,25.0019074742962,
5.92512971718013));
#450731=CARTESIAN_POINT('Ctrl Pts',(-6.74980468426065,24.9780797840648,
5.59309147117778));
#450732=CARTESIAN_POINT('Ctrl Pts',(-6.65752331243968,24.9542520938335,
5.2127054966016));
#450733=CARTESIAN_POINT('Ctrl Pts',(-6.42653317184816,24.9304244036021,
4.95822404429259));
#450734=CARTESIAN_POINT('Ctrl Pts',(-6.19554303125664,24.9065967133707,
4.70374259198359));
#450735=CARTESIAN_POINT('Ctrl Pts',(-5.82584412189456,24.8827690231393,
4.57516566194178));
#450736=CARTESIAN_POINT('Ctrl Pts',(-5.48679296352304,24.8589413329079,
4.63139343216518));
#450737=CARTESIAN_POINT('Ctrl Pts',(-5.14774180515151,24.8351136426765,
4.68762120238858));
#450738=CARTESIAN_POINT('Ctrl Pts',(-4.83933839777055,24.8112859524451,
4.9286536728772));
#450739=CARTESIAN_POINT('Ctrl Pts',(-4.70286022094558,24.7874582622137,
5.24407554312885));
#450740=CARTESIAN_POINT('Ctrl Pts',(-4.56638204412061,24.7636305719823,
5.55949741338051));
#450741=CARTESIAN_POINT('Ctrl Pts',(-4.60182909785165,24.7398028817509,
5.94930868339519));
#450742=CARTESIAN_POINT('Ctrl Pts',(-4.79296332969342,24.7159751915195,
6.23493948741375));
#450743=CARTESIAN_POINT('Ctrl Pts',(-4.83043362171106,24.7113039690887,
6.29093505415592));
#450744=CARTESIAN_POINT('Ctrl Pts',(-4.87388734148021,24.7066327466579,
6.34292671833547));
#450745=CARTESIAN_POINT('Ctrl Pts',(-4.92212745780799,24.7019615242271,
6.39028821611916));
#450746=CARTESIAN_POINT('Ctrl Pts',(-4.92408802232565,24.8230384757729,
6.38933869113556));
#450747=CARTESIAN_POINT('Ctrl Pts',(-4.80996622614209,24.8341159401463,
6.27560640646284));
#450748=CARTESIAN_POINT('Ctrl Pts',(-4.72108089883846,24.8451934045197,
6.13679925493306));
#450749=CARTESIAN_POINT('Ctrl Pts',(-4.67061008310121,24.8562708688931,
5.98520281626299));
#450750=CARTESIAN_POINT('Ctrl Pts',(-4.56204706519615,24.8800985591245,
5.65911799585187));
#450751=CARTESIAN_POINT('Ctrl Pts',(-4.63122130803993,24.9039262493559,
5.27385936922642));
#450752=CARTESIAN_POINT('Ctrl Pts',(-4.84644449237099,24.9277539395873,
5.00591117956891));
#450753=CARTESIAN_POINT('Ctrl Pts',(-5.06166767670205,24.9515816298187,
4.7379629899114));
#450754=CARTESIAN_POINT('Ctrl Pts',(-5.42293980252039,24.9754093200501,
4.58732523722183));
#450755=CARTESIAN_POINT('Ctrl Pts',(-5.7647647438604,24.9992370102815,4.62300419682159));
#450756=CARTESIAN_POINT('Ctrl Pts',(-6.10658968520039,25.0230647005129,
4.65868315642135));
#450757=CARTESIAN_POINT('Ctrl Pts',(-6.42896744206205,25.0468923907443,
4.88067882831044));
#450758=CARTESIAN_POINT('Ctrl Pts',(-6.58421869570625,25.0707200809757,
5.18729621377842));
#450759=CARTESIAN_POINT('Ctrl Pts',(-6.73946994935045,25.0945477712071,
5.49391359924639));
#450760=CARTESIAN_POINT('Ctrl Pts',(-6.72759469977719,25.1183754614385,
5.88515269829325));
#450761=CARTESIAN_POINT('Ctrl Pts',(-6.5540334824637,25.1422031516699,6.18179018209155));
#450762=CARTESIAN_POINT('Ctrl Pts',(-6.38047226515022,25.1660308419013,
6.47842766588984));
#450763=CARTESIAN_POINT('Ctrl Pts',(-6.0452250800965,25.1898585321326,6.68046353443956));
#450764=CARTESIAN_POINT('Ctrl Pts',(-5.70186524531576,25.213686222364,6.69534535485932));
#450765=CARTESIAN_POINT('Ctrl Pts',(-5.41677424787487,25.2334703068337,
6.70770170116848));
#450766=CARTESIAN_POINT('Ctrl Pts',(-5.12609043162756,25.2532543913033,
6.59103501365993));
#450767=CARTESIAN_POINT('Ctrl Pts',(-4.92197603118329,25.2730384757729,
6.39051881327128));
#450768=CARTESIAN_POINT('Origin',(-5.65685387860011,26.,5.65685387860011));
#450769=CARTESIAN_POINT('',(-4.92276701974739,25.7230384757729,6.39190058798136));
#450770=CARTESIAN_POINT('',(-4.92443355077908,25.6019615242271,6.39006796800886));
#450771=CARTESIAN_POINT('',(-4.92305381642377,26.,6.39065394077645));
#450772=CARTESIAN_POINT('',(-6.69274404704181,26.,5.59475217632209));
#450773=CARTESIAN_POINT('Ctrl Pts',(-4.92276701974739,25.7230384757729,
6.39190058798136));
#450774=CARTESIAN_POINT('Ctrl Pts',(-4.71160994855805,25.7438759131544,
6.17742942344334));
#450775=CARTESIAN_POINT('Ctrl Pts',(-4.59523934827088,25.764713350536,5.86562000134797));
#450776=CARTESIAN_POINT('Ctrl Pts',(-4.62142687258513,25.7855507879175,
5.56615422141076));
#450777=CARTESIAN_POINT('Ctrl Pts',(-4.65137240791476,25.8093784781489,
5.22371394391399));
#450778=CARTESIAN_POINT('Ctrl Pts',(-4.86772710302321,25.8332061683802,
4.89741422641509));
#450779=CARTESIAN_POINT('Ctrl Pts',(-5.17187737628347,25.8570338586116,
4.73725319022189));
#450780=CARTESIAN_POINT('Ctrl Pts',(-5.47602764954372,25.880861548843,4.57709215402869));
#450781=CARTESIAN_POINT('Ctrl Pts',(-5.86797350095578,25.9046892390744,
4.58306979914119));
#450782=CARTESIAN_POINT('Ctrl Pts',(-6.16698733288025,25.9285169293058,
4.75132533448083));
#450783=CARTESIAN_POINT('Ctrl Pts',(-6.46600116480472,25.9523446195372,
4.91958086982048));
#450784=CARTESIAN_POINT('Ctrl Pts',(-6.67208297724159,25.9761723097686,
5.25011429538726));
#450785=CARTESIAN_POINT('Ctrl Pts',(-6.69274404704181,26.,5.59475217632212));
#450786=CARTESIAN_POINT('',(-5.59444809180803,26.,6.69457727933146));
#450787=CARTESIAN_POINT('Origin',(-5.65685387860011,26.,5.65685387860011));
#450788=CARTESIAN_POINT('Ctrl Pts',(-5.59444726164187,26.,6.69458228414866));
#450789=CARTESIAN_POINT('Ctrl Pts',(-5.92484673178863,25.9770624644402,
6.71351646533254));
#450790=CARTESIAN_POINT('Ctrl Pts',(-6.26627937525033,25.9541249288804,
6.56158375468957));
#450791=CARTESIAN_POINT('Ctrl Pts',(-6.47167795527827,25.9311873933205,
6.30214239804397));
#450792=CARTESIAN_POINT('Ctrl Pts',(-6.68504759676004,25.9073597030892,
6.03263270014108));
#450793=CARTESIAN_POINT('Ctrl Pts',(-6.75161994353754,25.8835320128578,
5.64710810132191));
#450794=CARTESIAN_POINT('Ctrl Pts',(-6.64083855948586,25.8597043226264,
5.32182159136527));
#450795=CARTESIAN_POINT('Ctrl Pts',(-6.53005717543418,25.835876632395,4.99653508140864));
#450796=CARTESIAN_POINT('Ctrl Pts',(-6.24192206055333,25.8120489421636,
4.73148666031454));
#450797=CARTESIAN_POINT('Ctrl Pts',(-5.90845611919747,25.7882212519322,
4.64827248224482));
#450798=CARTESIAN_POINT('Ctrl Pts',(-5.57499017784161,25.7643935617008,
4.56505830417509));
#450799=CARTESIAN_POINT('Ctrl Pts',(-5.19619341001074,25.7405658714694,
4.66367836912974));
#450800=CARTESIAN_POINT('Ctrl Pts',(-4.94557465216384,25.716738181238,4.89886414913016));
#450801=CARTESIAN_POINT('Ctrl Pts',(-4.69495589431694,25.6929104910066,
5.13404992913058));
#450802=CARTESIAN_POINT('Ctrl Pts',(-4.572515146454,25.6690828007752,5.50580142417677));
#450803=CARTESIAN_POINT('Ctrl Pts',(-4.63434949773116,25.6452551105439,
5.84386841174159));
#450804=CARTESIAN_POINT('Ctrl Pts',(-4.67179935541582,25.6308239151049,
6.04861804217652));
#450805=CARTESIAN_POINT('Ctrl Pts',(-4.7768430935332,25.616392719666,6.24101187097706));
#450806=CARTESIAN_POINT('Ctrl Pts',(-4.92443355077908,25.6019615242271,
6.39006796800886));
#450807=CARTESIAN_POINT('Origin',(-5.65685387860011,26.993675081176,5.65685387860011));
#450808=CARTESIAN_POINT('',(-4.74524035180399,22.756324918824,6.5673434103921));
#450809=CARTESIAN_POINT('',(-4.74364038176039,22.718675081176,6.57057146528765));
#450810=CARTESIAN_POINT('',(-4.74468613086949,26.993675081176,6.56902162633079));
#450811=CARTESIAN_POINT('',(-6.64591806159944,22.5,4.8286920333622));
#450812=CARTESIAN_POINT('Ctrl Pts',(-4.74364038176039,22.718675081176,6.57057146528766));
#450813=CARTESIAN_POINT('Ctrl Pts',(-4.76142457130848,22.7172664581449,
6.58852418981576));
#450814=CARTESIAN_POINT('Ctrl Pts',(-5.09000197050781,22.6920301448823,
6.9000556810006));
#450815=CARTESIAN_POINT('Ctrl Pts',(-6.06611679986992,22.6429661413884,
7.12689194633153));
#450816=CARTESIAN_POINT('Ctrl Pts',(-7.11331947438321,22.5714830706942,
6.10694434613243));
#450817=CARTESIAN_POINT('Ctrl Pts',(-6.92144528650133,22.5238276902314,
5.15775103452081));
#450818=CARTESIAN_POINT('Ctrl Pts',(-6.64591806159944,22.5,4.8286920333622));
#450819=CARTESIAN_POINT('',(-6.09734856608926,22.5,4.44194770692244));
#450820=CARTESIAN_POINT('Origin',(-5.65685387860011,22.5,5.65685387860011));
#450821=CARTESIAN_POINT('Ctrl Pts',(-4.74524035180399,22.756324918824,6.5673434103921));
#450822=CARTESIAN_POINT('Ctrl Pts',(-4.93595953019022,22.7414761952386,
6.75594870135602));
#450823=CARTESIAN_POINT('Ctrl Pts',(-5.58182921801751,22.7027997814218,
7.10121210146151));
#450824=CARTESIAN_POINT('Ctrl Pts',(-6.78713386963137,22.6402956773736,
6.6805523241845));
#450825=CARTESIAN_POINT('Ctrl Pts',(-7.12528591239125,22.569702761351,5.27997950888059));
#450826=CARTESIAN_POINT('Ctrl Pts',(-6.48370144903283,22.5229375355598,
4.58325719964657));
#450827=CARTESIAN_POINT('Ctrl Pts',(-6.09735008669021,22.5,4.44194158662797));
#450828=CARTESIAN_POINT('Origin',(-5.65685387860011,26.993675081176,5.65685387860011));
#450829=CARTESIAN_POINT('',(-4.74299838399068,23.206324918824,6.56983844394705));
#450830=CARTESIAN_POINT('',(-4.74631652959707,23.168675081176,6.56867439792569));
#450831=CARTESIAN_POINT('',(-4.74468613086949,26.993675081176,6.56902162633079));
#450832=CARTESIAN_POINT('Ctrl Pts',(-4.74631652959707,23.168675081176,6.56867439792569));
#450833=CARTESIAN_POINT('Ctrl Pts',(-4.853408844765,23.1602325995332,6.67716702479821));
#450834=CARTESIAN_POINT('Ctrl Pts',(-5.33214451040115,23.127962427659,7.02077633180239));
#450835=CARTESIAN_POINT('Ctrl Pts',(-6.47507582842176,23.0718645655535,
6.94377741359718));
#450836=CARTESIAN_POINT('Ctrl Pts',(-7.18181942856023,23.0003814948592,
5.66653874837814));
#450837=CARTESIAN_POINT('Ctrl Pts',(-6.49141154940691,22.9288984241651,
4.38054591235378));
#450838=CARTESIAN_POINT('Ctrl Pts',(-5.03639155729104,22.8574153534709,
4.26365553420012));
#450839=CARTESIAN_POINT('Ctrl Pts',(-4.16730445086878,22.7873409058079,
5.40079341912851));
#450840=CARTESIAN_POINT('Ctrl Pts',(-4.46059450521194,22.7410941483762,
6.28484325502835));
#450841=CARTESIAN_POINT('Ctrl Pts',(-4.74364038176039,22.718675081176,6.57057146528766));
#450842=CARTESIAN_POINT('Ctrl Pts',(-4.74299838399068,23.206324918824,6.56983844394705));
#450843=CARTESIAN_POINT('Ctrl Pts',(-5.02227299078827,23.184442336627,6.84584090104065));
#450844=CARTESIAN_POINT('Ctrl Pts',(-5.88847306909541,23.1387320641985,
7.14533371342118));
#450845=CARTESIAN_POINT('Ctrl Pts',(-7.03563221165043,23.0691941015387,
6.3084575374563));
#450846=CARTESIAN_POINT('Ctrl Pts',(-6.95165327175697,22.9977110308445,
4.85119529970875));
#450847=CARTESIAN_POINT('Ctrl Pts',(-5.68141376558384,22.9262279601503,
4.13204038713623));
#450848=CARTESIAN_POINT('Ctrl Pts',(-4.38863987327371,22.8547448894562,
4.80994952176022));
#450849=CARTESIAN_POINT('Ctrl Pts',(-4.28501879514303,22.7981105423474,
5.9617065202947));
#450850=CARTESIAN_POINT('Ctrl Pts',(-4.62991319040622,22.76530388547,6.45329450867431));
#450851=CARTESIAN_POINT('Ctrl Pts',(-4.74524035180399,22.756324918824,6.5673434103921));
#450852=CARTESIAN_POINT('Origin',(-5.65685387860011,26.993675081176,5.65685387860011));
#450853=CARTESIAN_POINT('',(-4.74532300381163,23.656324918824,6.57003272085371));
#450854=CARTESIAN_POINT('',(-4.74499326893249,23.618675081176,6.56740434249263));
#450855=CARTESIAN_POINT('',(-4.74468613086949,26.993675081176,6.56902162633079));
#450856=CARTESIAN_POINT('Ctrl Pts',(-4.74499326893249,23.618675081176,6.56740434249263));
#450857=CARTESIAN_POINT('Ctrl Pts',(-4.94389036502613,23.6031987409216,
6.76368003125862));
#450858=CARTESIAN_POINT('Ctrl Pts',(-5.60787864620878,23.5638947104357,
7.10715379447204));
#450859=CARTESIAN_POINT('Ctrl Pts',(-6.81352117024561,23.5007629897185,
6.65070324968042));
#450860=CARTESIAN_POINT('Ctrl Pts',(-7.11892889768229,23.4292799190243,
5.22331918686542));
#450861=CARTESIAN_POINT('Ctrl Pts',(-6.08480364614363,23.3577968483302,
4.19313572939823));
#450862=CARTESIAN_POINT('Ctrl Pts',(-4.65859667867589,23.2863137776359,
4.50398657889369));
#450863=CARTESIAN_POINT('Ctrl Pts',(-4.20740365817457,23.2232731885846,
5.70962577012502));
#450864=CARTESIAN_POINT('Ctrl Pts',(-4.55115618731809,23.1840602897646,
6.37096218895919));
#450865=CARTESIAN_POINT('Ctrl Pts',(-4.74631652959707,23.168675081176,6.56867439792569));
#450866=CARTESIAN_POINT('Ctrl Pts',(-4.74532300381163,23.656324918824,6.57003272085371));
#450867=CARTESIAN_POINT('Ctrl Pts',(-4.80948437015677,23.6512361682467,
6.63539236159828));
#450868=CARTESIAN_POINT('Ctrl Pts',(-5.21266771861287,23.622319727438,6.9668858368575));
#450869=CARTESIAN_POINT('Ctrl Pts',(-6.28682364983266,23.569575596398,7.04564953674368));
#450870=CARTESIAN_POINT('Ctrl Pts',(-7.16543624640093,23.4980925257038,
5.88000083782648));
#450871=CARTESIAN_POINT('Ctrl Pts',(-6.66190630419616,23.4266094550096,
4.50990820099156));
#450872=CARTESIAN_POINT('Ctrl Pts',(-5.23756146736659,23.3551263843154,
4.19063094092434));
#450873=CARTESIAN_POINT('Ctrl Pts',(-4.19736598356862,23.2836433136212,
5.21468783779196));
#450874=CARTESIAN_POINT('Ctrl Pts',(-4.40342562281452,23.2340428251241,
6.20635078283889));
#450875=CARTESIAN_POINT('Ctrl Pts',(-4.71817410701172,23.2082700268584,
6.54530502316694));
#450876=CARTESIAN_POINT('Ctrl Pts',(-4.74299838399068,23.206324918824,6.56983844394705));
#450877=CARTESIAN_POINT('Origin',(-5.65685387860011,26.993675081176,5.65685387860011));
#450878=CARTESIAN_POINT('',(-4.74613115927677,24.106324918824,6.56748881619374));
#450879=CARTESIAN_POINT('',(-4.74299681637215,24.068675081176,6.57010232725217));
#450880=CARTESIAN_POINT('',(-4.74468613086949,26.993675081176,6.56902162633079));
#450881=CARTESIAN_POINT('Ctrl Pts',(-4.74299681637215,24.068675081176,6.57010232725217));
#450882=CARTESIAN_POINT('Ctrl Pts',(-5.02972694085412,24.0461648823099,
6.85435514987614));
#450883=CARTESIAN_POINT('Ctrl Pts',(-5.91736950865738,23.9998269932124,
7.14655186859909));
#450884=CARTESIAN_POINT('Ctrl Pts',(-7.0522818436793,23.9296614138836,6.27199288310558));
#450885=CARTESIAN_POINT('Ctrl Pts',(-6.93003241982605,23.8581783431894,
4.81743049717126));
#450886=CARTESIAN_POINT('Ctrl Pts',(-5.64131435190337,23.7866952724952,
4.13193628895796));
#450887=CARTESIAN_POINT('Ctrl Pts',(-4.3668333837381,23.715212201801,4.84355050202496));
#450888=CARTESIAN_POINT('Ctrl Pts',(-4.29429575151249,23.6592054713613,
5.98491025846011));
#450889=CARTESIAN_POINT('Ctrl Pts',(-4.63766432477859,23.627026431153,6.4614899633887));
#450890=CARTESIAN_POINT('Ctrl Pts',(-4.74499326893249,23.618675081176,6.56740434249263));
#450891=CARTESIAN_POINT('Ctrl Pts',(-4.74613115927677,24.106324918824,6.56748881619374));
#450892=CARTESIAN_POINT('Ctrl Pts',(-4.90119115627847,24.0942023096351,
6.72241589762581));
#450893=CARTESIAN_POINT('Ctrl Pts',(-5.47210261995128,24.0582520102147,
7.07096798466868));
#450894=CARTESIAN_POINT('Ctrl Pts',(-6.662968703113,23.998474020563,6.80286792203874));
#450895=CARTESIAN_POINT('Ctrl Pts',(-7.16522879152533,23.9269909498688,
5.43230911237055));
#450896=CARTESIAN_POINT('Ctrl Pts',(-6.2855365564656,23.8555078791747,4.26747512907024));
#450897=CARTESIAN_POINT('Ctrl Pts',(-4.82985391579145,23.7840248084805,
4.37557081254884));
#450898=CARTESIAN_POINT('Ctrl Pts',(-4.18154636230721,23.7176304883636,
5.56629788826614));
#450899=CARTESIAN_POINT('Ctrl Pts',(-4.50905361827065,23.6750638584781,
6.32935078034095));
#450900=CARTESIAN_POINT('Ctrl Pts',(-4.74532300381163,23.656324918824,6.57003272085371));
#450901=CARTESIAN_POINT('Origin',(-5.65685387860011,26.993675081176,5.65685387860011));
#450902=CARTESIAN_POINT('',(-4.74353459859835,24.556324918824,6.56856700353347));
#450903=CARTESIAN_POINT('',(-4.74557835604531,24.518675081176,6.56980231202958));
#450904=CARTESIAN_POINT('',(-4.74468613086949,26.993675081176,6.56902162633079));
#450905=CARTESIAN_POINT('Ctrl Pts',(-4.74557835604531,24.518675081176,6.56980231202958));
#450906=CARTESIAN_POINT('Ctrl Pts',(-4.81770944620421,24.5129587139297,
6.64326578517921));
#450907=CARTESIAN_POINT('Ctrl Pts',(-5.23445549419879,24.4834146564519,
6.97750833641272));
#450908=CARTESIAN_POINT('Ctrl Pts',(-6.32311258055822,24.4300429087428,
7.0286098827299));
#450909=CARTESIAN_POINT('Ctrl Pts',(-7.17078066054311,24.3585598380486,
5.84026841822956));
#450910=CARTESIAN_POINT('Ctrl Pts',(-6.63140987332417,24.2870767673545,
4.4838850778304));
#450911=CARTESIAN_POINT('Ctrl Pts',(-5.19916430623342,24.2155936966603,
4.2021595986403));
#450912=CARTESIAN_POINT('Ctrl Pts',(-4.18624762160046,24.1441106259661,
5.25320498229437));
#450913=CARTESIAN_POINT('Ctrl Pts',(-4.41536649518845,24.095137754138,6.22663461042285));
#450914=CARTESIAN_POINT('Ctrl Pts',(-4.72621489163553,24.0699925725413,
6.55346539562852));
#450915=CARTESIAN_POINT('Ctrl Pts',(-4.74299681637215,24.068675081176,6.57010232725217));
#450916=CARTESIAN_POINT('Ctrl Pts',(-4.74353459859835,24.556324918824,6.56856700353347));
#450917=CARTESIAN_POINT('Ctrl Pts',(-4.9894525322227,24.5371684510234,6.81000592522228));
#450918=CARTESIAN_POINT('Ctrl Pts',(-5.76578134653658,24.4941842929915,
7.13455935910424));
#450919=CARTESIAN_POINT('Ctrl Pts',(-6.95240396480877,24.4273724447281,
6.4613196666284));
#450920=CARTESIAN_POINT('Ctrl Pts',(-7.03502543671246,24.3558893740339,
5.00396921476326));
#450921=CARTESIAN_POINT('Ctrl Pts',(-5.85498510857851,24.2844063033397,
4.14478270244581));
#450922=CARTESIAN_POINT('Ctrl Pts',(-4.49341967622111,24.2129232326456,
4.67093497503136));
#450923=CARTESIAN_POINT('Ctrl Pts',(-4.24791389261248,24.1535627711403,
5.85795834238072));
#450924=CARTESIAN_POINT('Ctrl Pts',(-4.59641175456261,24.1180299998664,
6.41789774915756));
#450925=CARTESIAN_POINT('Ctrl Pts',(-4.74613115927677,24.106324918824,6.56748881619374));
#450926=CARTESIAN_POINT('Origin',(-5.65685387860011,26.993675081176,5.65685387860011));
#450927=CARTESIAN_POINT('',(-4.74405758279954,25.006324918824,6.57067994464873));
#450928=CARTESIAN_POINT('',(-4.74597172529335,24.968675081176,6.56738667375376));
#450929=CARTESIAN_POINT('',(-4.74468613086949,26.993675081176,6.56902162633079));
#450930=CARTESIAN_POINT('Ctrl Pts',(-4.74597172529336,24.968675081176,6.56738667375376));
#450931=CARTESIAN_POINT('Ctrl Pts',(-4.90925551921452,24.955924855318,6.73011316031215));
#450932=CARTESIAN_POINT('Ctrl Pts',(-5.49691387622178,24.9193469392286,
7.07847832230359));
#450933=CARTESIAN_POINT('Ctrl Pts',(-6.69274573713214,24.8589413329079,
6.77602463836695));
#450934=CARTESIAN_POINT('Ctrl Pts',(-7.15880506797054,24.7874582622137,
5.39273679116275));
#450935=CARTESIAN_POINT('Ctrl Pts',(-6.24879737998678,24.7159751915195,
4.25142935492228));
#450936=CARTESIAN_POINT('Ctrl Pts',(-4.79645922145989,24.6444921208253,
4.39775252453571));
#450937=CARTESIAN_POINT('Ctrl Pts',(-4.18550614000559,24.5787254173775,
5.59369688000734));
#450938=CARTESIAN_POINT('Ctrl Pts',(-4.51704344657683,24.5367864041611,
6.33704597702196));
#450939=CARTESIAN_POINT('Ctrl Pts',(-4.74557835604531,24.518675081176,6.56980231202958));
#450940=CARTESIAN_POINT('Ctrl Pts',(-4.74405758279954,25.006324918824,6.57067994464873));
#450941=CARTESIAN_POINT('Ctrl Pts',(-4.77384081402403,25.0039622826432,
6.60086819803686));
#450942=CARTESIAN_POINT('Ctrl Pts',(-5.12098437694123,24.9777719562309,
6.91811250300101));
#450943=CARTESIAN_POINT('Ctrl Pts',(-6.12447699388038,24.9277539395873,
7.10838527255516));
#450944=CARTESIAN_POINT('Ctrl Pts',(-7.13018513270865,24.8562708688931,
6.05044038944422));
#450945=CARTESIAN_POINT('Ctrl Pts',(-6.78604742232836,24.784787798199,4.63189669239788));
#450946=CARTESIAN_POINT('Ctrl Pts',(-5.40735816264999,24.7133047275048,
4.15240479236238));
#450947=CARTESIAN_POINT('Ctrl Pts',(-4.25725342975252,24.6418216568106,
5.05126835371239));
#450948=CARTESIAN_POINT('Ctrl Pts',(-4.35401829743014,24.589495053917,6.11539165852711));
#450949=CARTESIAN_POINT('Ctrl Pts',(-4.68356856625642,24.5609961412548,
6.50969315902277));
#450950=CARTESIAN_POINT('Ctrl Pts',(-4.74353459859835,24.556324918824,6.56856700353347));
#450951=CARTESIAN_POINT('Origin',(-5.65685387860011,26.993675081176,5.65685387860011));
#450952=CARTESIAN_POINT('',(-4.74640124271564,25.456324918824,6.56829321884323));
#450953=CARTESIAN_POINT('',(-4.74334636410459,25.418675081176,6.56885365284802));
#450954=CARTESIAN_POINT('',(-4.74468613086949,26.993675081176,6.56902162633079));
#450955=CARTESIAN_POINT('Ctrl Pts',(-4.74334636410459,25.418675081176,6.56885365284802));
#450956=CARTESIAN_POINT('Ctrl Pts',(-4.99707565976646,25.3988909967064,
6.81811011972481));
#450957=CARTESIAN_POINT('Ctrl Pts',(-5.79361205385018,25.3552792220053,
7.13780202337966));
#450958=CARTESIAN_POINT('Ctrl Pts',(-6.97310209577086,25.287839757073,6.42698533143036));
#450959=CARTESIAN_POINT('Ctrl Pts',(-7.01738753624157,25.2163566863788,
4.96796792520407));
#450960=CARTESIAN_POINT('Ctrl Pts',(-5.81516935358237,25.1448736156846,
4.14009680960707));
#450961=CARTESIAN_POINT('Ctrl Pts',(-4.4679054394248,25.0733905449904,4.70185841202445));
#450962=CARTESIAN_POINT('Ctrl Pts',(-4.25595199715398,25.0146577001542,
5.88231068328695));
#450963=CARTESIAN_POINT('Ctrl Pts',(-4.604109892408,24.9797525455494,6.4260090324839));
#450964=CARTESIAN_POINT('Ctrl Pts',(-4.74597172529336,24.968675081176,6.56738667375376));
#450965=CARTESIAN_POINT('Ctrl Pts',(-4.74640124271564,25.456324918824,6.56829321884323));
#450966=CARTESIAN_POINT('Ctrl Pts',(-4.86586022639608,25.4469284240315,
6.68893848409317));
#450967=CARTESIAN_POINT('Ctrl Pts',(-5.36752678600608,25.4137042390077,
7.03476003379299));
#450968=CARTESIAN_POINT('Ctrl Pts',(-6.5258341885166,25.3566523637524,6.91003560334641));
#450969=CARTESIAN_POINT('Ctrl Pts',(-7.18099123031483,25.2851692930582,
5.60564496305));
#450970=CARTESIAN_POINT('Ctrl Pts',(-6.43975200870338,25.213686222364,4.34815567114859));
#450971=CARTESIAN_POINT('Ctrl Pts',(-4.98123363545819,25.1422031516699,
4.28968558428151));
#450972=CARTESIAN_POINT('Ctrl Pts',(-4.16945626611646,25.0730827171565,
5.44432497425889));
#450973=CARTESIAN_POINT('Ctrl Pts',(-4.47347056935133,25.0277899728746,
6.29641321838457));
#450974=CARTESIAN_POINT('Ctrl Pts',(-4.74405758279954,25.006324918824,6.57067994464873));
#450975=CARTESIAN_POINT('Origin',(-5.65685387860011,26.993675081176,5.65685387860011));
#450976=CARTESIAN_POINT('',(-4.7445060113485,25.906324918824,6.56704169373441));
#450977=CARTESIAN_POINT('',(-4.74432962138981,25.868675081176,6.57057130100612));
#450978=CARTESIAN_POINT('',(-4.74468613086949,26.993675081176,6.56902162633079));
#450979=CARTESIAN_POINT('',(-4.53900700771688,26.,5.01302286563433));
#450980=CARTESIAN_POINT('Ctrl Pts',(-4.53900700771688,26.,5.01302286563431));
#450981=CARTESIAN_POINT('Ctrl Pts',(-4.32480615636363,25.9761723097686,
5.38492752167559));
#450982=CARTESIAN_POINT('Ctrl Pts',(-4.30899334914827,25.9449472827099,
6.01924597306242));
#450983=CARTESIAN_POINT('Ctrl Pts',(-4.64940368207851,25.9137222556513,
6.47338425157138));
#450984=CARTESIAN_POINT('Ctrl Pts',(-4.7445060113485,25.906324918824,6.56704169373441));
#450985=CARTESIAN_POINT('',(-5.01208503488091,26.,4.53689596693371));
#450986=CARTESIAN_POINT('Origin',(-5.65685387860011,26.,5.65685387860011));
#450987=CARTESIAN_POINT('Ctrl Pts',(-5.01208247494518,26.,4.5368902045627));
#450988=CARTESIAN_POINT('Ctrl Pts',(-4.65613984562121,25.9770624644402,
4.74314812622022));
#450989=CARTESIAN_POINT('Ctrl Pts',(-4.17795197796788,25.9332874914989,
5.48969900651177));
#450990=CARTESIAN_POINT('Ctrl Pts',(-4.48184576512937,25.8895125185575,
6.3039677816093));
#450991=CARTESIAN_POINT('Ctrl Pts',(-4.74432962138981,25.868675081176,6.57057130100612));
#450992=CARTESIAN_POINT('Origin',(5.65685387860011,26.,5.65685387860011));
#450993=CARTESIAN_POINT('',(6.39190072013885,22.573038475773,4.9222125558517));
#450994=CARTESIAN_POINT('',(6.39065394077645,22.5,4.92305381642377));
#450995=CARTESIAN_POINT('',(6.39065394077645,26.,4.92305381642377));
#450996=CARTESIAN_POINT('',(6.66622270032004,22.5,5.8978925564917));
#450997=CARTESIAN_POINT('Origin',(5.65685387860011,22.5,5.65685387860011));
#450998=CARTESIAN_POINT('Ctrl Pts',(6.66798006829997,22.5,5.89851203167784));
#450999=CARTESIAN_POINT('Ctrl Pts',(6.7439998684947,22.5229375355598,5.57641995134461));
#451000=CARTESIAN_POINT('Ctrl Pts',(6.65366449057419,22.5458750711197,5.21379162224851));
#451001=CARTESIAN_POINT('Ctrl Pts',(6.43383171727969,22.5688126066795,4.96646199655034));
#451002=CARTESIAN_POINT('Ctrl Pts',(6.42033150900062,22.5702212297106,4.95127317183385));
#451003=CARTESIAN_POINT('Ctrl Pts',(6.40634292159547,22.5716298527418,4.93651917810251));
#451004=CARTESIAN_POINT('Ctrl Pts',(6.39190072013885,22.573038475773,4.9222125558517));
#451005=CARTESIAN_POINT('Origin',(5.65685387860011,26.,5.65685387860011));
#451006=CARTESIAN_POINT('',(6.39037461032892,23.0230384757729,4.92436540268704));
#451007=CARTESIAN_POINT('',(6.38930388760559,22.9019615242271,4.92349966353597));
#451008=CARTESIAN_POINT('',(6.39065394077645,26.,4.92305381642377));
#451009=CARTESIAN_POINT('',(5.77557608073439,22.5,4.62591736201901));
#451010=CARTESIAN_POINT('Ctrl Pts',(6.38930388760559,22.9019615242271,4.92349966353597));
#451011=CARTESIAN_POINT('Ctrl Pts',(6.54102880287524,22.8871128006417,5.07692511110986));
#451012=CARTESIAN_POINT('Ctrl Pts',(6.64766299899898,22.8722640770563,5.27640120658105));
#451013=CARTESIAN_POINT('Ctrl Pts',(6.68249361011691,22.8574153534709,5.48772889025785));
#451014=CARTESIAN_POINT('Ctrl Pts',(6.73838615923167,22.8335876632395,5.82684562005692));
#451015=CARTESIAN_POINT('Ctrl Pts',(6.60938089562333,22.8097599730081,6.19648078060475));
#451016=CARTESIAN_POINT('Ctrl Pts',(6.35472685290066,22.7859322827767,6.42720821100082));
#451017=CARTESIAN_POINT('Ctrl Pts',(6.10007281017799,22.7621045925453,6.65793564139689));
#451018=CARTESIAN_POINT('Ctrl Pts',(5.71976998834099,22.7382769023139,6.74975534164119));
#451019=CARTESIAN_POINT('Ctrl Pts',(5.38773213421059,22.7144492120825,6.66080060824128));
#451020=CARTESIAN_POINT('Ctrl Pts',(5.05569428008018,22.6906215218511,6.57184587484137));
#451021=CARTESIAN_POINT('Ctrl Pts',(4.77192139365638,22.6667938316197,6.30211670779724));
#451022=CARTESIAN_POINT('Ctrl Pts',(4.66700870222797,22.6429661413884,5.97477550103877));
#451023=CARTESIAN_POINT('Ctrl Pts',(4.56209601079956,22.619138451157,5.6474342942803));
#451024=CARTESIAN_POINT('Ctrl Pts',(4.63604351436656,22.5953107609256,5.26248104780748));
#451025=CARTESIAN_POINT('Ctrl Pts',(4.85366607828882,22.5714830706942,4.99722717517853));
#451026=CARTESIAN_POINT('Ctrl Pts',(5.07128864221107,22.5476553804628,4.73197330254958));
#451027=CARTESIAN_POINT('Ctrl Pts',(5.43258626648858,22.5238276902314,4.58641880376449));
#451028=CARTESIAN_POINT('Ctrl Pts',(5.77557608073438,22.5,4.625917362019));
#451029=CARTESIAN_POINT('Origin',(5.65685387860011,22.5,5.65685387860011));
#451030=CARTESIAN_POINT('Ctrl Pts',(6.39190072013885,22.573038475773,4.9222125558517));
#451031=CARTESIAN_POINT('Ctrl Pts',(6.16204455719575,22.5954575429732,4.69451421601594));
#451032=CARTESIAN_POINT('Ctrl Pts',(5.81728522517979,22.6178766101734,4.58013776446743));
#451033=CARTESIAN_POINT('Ctrl Pts',(5.49777863793003,22.6402956773736,4.62964039434809));
#451034=CARTESIAN_POINT('Ctrl Pts',(5.15819698094666,22.664123367605,4.68225334741615));
#451035=CARTESIAN_POINT('Ctrl Pts',(4.84714109570319,22.6879510578364,4.91998587117151));
#451036=CARTESIAN_POINT('Ctrl Pts',(4.70728537400252,22.7117787480678,5.23393572436938));
#451037=CARTESIAN_POINT('Ctrl Pts',(4.56742965230184,22.7356064382992,5.54788557756724));
#451038=CARTESIAN_POINT('Ctrl Pts',(4.59877409414395,22.7594341285306,5.93805276020761));
#451039=CARTESIAN_POINT('Ctrl Pts',(4.78686738296995,22.783261818762,6.22570363532513));
#451040=CARTESIAN_POINT('Ctrl Pts',(4.97496067179595,22.8070895089934,6.51335451044265));
#451041=CARTESIAN_POINT('Ctrl Pts',(5.31980280760584,22.8309171992248,6.69848907803731));
#451042=CARTESIAN_POINT('Ctrl Pts',(5.66347121722023,22.8547448894562,6.69629884619592));
#451043=CARTESIAN_POINT('Ctrl Pts',(6.00713962683461,22.8785725796876,6.69410861435454));
#451044=CARTESIAN_POINT('Ctrl Pts',(6.34963431025349,22.902400269919,6.5045935830771));
#451045=CARTESIAN_POINT('Ctrl Pts',(6.53403672593788,22.9262279601503,6.21456908983246));
#451046=CARTESIAN_POINT('Ctrl Pts',(6.71843914162228,22.9500556503817,5.92454459658782));
#451047=CARTESIAN_POINT('Ctrl Pts',(6.7447492895722,22.9738833406131,5.53401064137597));
#451048=CARTESIAN_POINT('Ctrl Pts',(6.60092695407667,22.9977110308445,5.22186823831327));
#451049=CARTESIAN_POINT('Ctrl Pts',(6.54996870275417,23.0061535124873,5.11127184889382));
#451050=CARTESIAN_POINT('Ctrl Pts',(6.47765230299322,23.0145959941301,5.01051660428821));
#451051=CARTESIAN_POINT('Ctrl Pts',(6.39037461032892,23.0230384757729,4.92436540268704));
#451052=CARTESIAN_POINT('Origin',(5.65685387860011,26.,5.65685387860011));
#451053=CARTESIAN_POINT('',(6.38935290488262,23.4730384757729,4.92330089590042));
#451054=CARTESIAN_POINT('',(6.39131103572319,23.3519615242271,4.92169609601798));
#451055=CARTESIAN_POINT('',(6.39065394077645,26.,4.92305381642377));
#451056=CARTESIAN_POINT('Ctrl Pts',(6.39131103572319,23.3519615242271,4.92169609601798));
#451057=CARTESIAN_POINT('Ctrl Pts',(6.61334324490838,23.33007894203,5.14636061012976));
#451058=CARTESIAN_POINT('Ctrl Pts',(6.72868171719176,23.308196359833,5.47994522249351));
#451059=CARTESIAN_POINT('Ctrl Pts',(6.6873844849522,23.286313777636,5.79285848911253));
#451060=CARTESIAN_POINT('Ctrl Pts',(6.64241640721998,23.2624860874046,6.1335861198444));
#451061=CARTESIAN_POINT('Ctrl Pts',(6.41172882390928,23.2386583971732,6.44980419113038));
#451062=CARTESIAN_POINT('Ctrl Pts',(6.10100080909856,23.2148307069418,6.59665364733223));
#451063=CARTESIAN_POINT('Ctrl Pts',(5.79027279428784,23.1910030167104,6.74350310353408));
#451064=CARTESIAN_POINT('Ctrl Pts',(5.39950434797711,23.167175326479,6.7209839446518));
#451065=CARTESIAN_POINT('Ctrl Pts',(5.10769854723491,23.1433476362476,6.539415444341));
#451066=CARTESIAN_POINT('Ctrl Pts',(4.8158927464927,23.1195199460162,6.3578469440302));
#451067=CARTESIAN_POINT('Ctrl Pts',(4.62304959131903,23.0956922557848,6.01722910229088));
#451068=CARTESIAN_POINT('Ctrl Pts',(4.61751951301592,23.0718645655534,5.67358993507176));
#451069=CARTESIAN_POINT('Ctrl Pts',(4.61198943471281,23.048036875322,5.32995076785264));
#451070=CARTESIAN_POINT('Ctrl Pts',(4.79377243328026,23.0242091850907,4.98329027515371));
#451071=CARTESIAN_POINT('Ctrl Pts',(5.07957475014376,23.0003814948593,4.7924243254548));
#451072=CARTESIAN_POINT('Ctrl Pts',(5.36537706700727,22.9765538046279,4.60155837575589));
#451073=CARTESIAN_POINT('Ctrl Pts',(5.75519870216683,22.9527261143965,4.566486969057));
#451074=CARTESIAN_POINT('Ctrl Pts',(6.07050470066555,22.9288984241651,4.70325041523272));
#451075=CARTESIAN_POINT('Ctrl Pts',(6.18932117076025,22.9199194575191,4.75478685916323));
#451076=CARTESIAN_POINT('Ctrl Pts',(6.29755640872372,22.9109404908731,4.83072387924101));
#451077=CARTESIAN_POINT('Ctrl Pts',(6.38930388760559,22.9019615242271,4.92349966353597));
#451078=CARTESIAN_POINT('Ctrl Pts',(6.39037461032892,23.0230384757729,4.92436540268704));
#451079=CARTESIAN_POINT('Ctrl Pts',(6.23132356780567,23.0384236843615,4.76736722811336));
#451080=CARTESIAN_POINT('Ctrl Pts',(6.02258634020352,23.0538088929501,4.65886881811934));
#451081=CARTESIAN_POINT('Ctrl Pts',(5.80287677492702,23.0691941015387,4.62769529041208));
#451082=CARTESIAN_POINT('Ctrl Pts',(5.46260375021388,23.0930217917701,4.57941559648715));
#451083=CARTESIAN_POINT('Ctrl Pts',(5.09601251972856,23.1168494820015,4.71660705955086));
#451084=CARTESIAN_POINT('Ctrl Pts',(4.87103919530453,23.1406771722329,4.97642324075838));
#451085=CARTESIAN_POINT('Ctrl Pts',(4.64606587088049,23.1645048624643,5.2362394219659));
#451086=CARTESIAN_POINT('Ctrl Pts',(4.56271045251773,23.1883325526957,5.61868032131723));
#451087=CARTESIAN_POINT('Ctrl Pts',(4.65915585483332,23.2121602429271,5.94855238336812));
#451088=CARTESIAN_POINT('Ctrl Pts',(4.75560125714891,23.2359879331585,6.278424445419));
#451089=CARTESIAN_POINT('Ctrl Pts',(5.03184748014285,23.2598156233899,6.55572767016945));
#451090=CARTESIAN_POINT('Ctrl Pts',(5.36134886181892,23.2836433136212,6.65343136663416));
#451091=CARTESIAN_POINT('Ctrl Pts',(5.690850243495,23.3074710038526,6.75113506309886));
#451092=CARTESIAN_POINT('Ctrl Pts',(6.07360678385322,23.331298694084,6.66923923127783));
#451093=CARTESIAN_POINT('Ctrl Pts',(6.33427992409048,23.3551263843154,6.44525978436571));
#451094=CARTESIAN_POINT('Ctrl Pts',(6.59495306432775,23.3789540745468,6.22128033745359));
#451095=CARTESIAN_POINT('Ctrl Pts',(6.73354280444407,23.4027817647782,5.85521727545038));
#451096=CARTESIAN_POINT('Ctrl Pts',(6.6865623548039,23.4266094550096,5.51476156795534));
#451097=CARTESIAN_POINT('Ctrl Pts',(6.65604804910002,23.442085795264,5.29363193601897));
#451098=CARTESIAN_POINT('Ctrl Pts',(6.54724832815155,23.4575621355185,5.08330512959901));
#451099=CARTESIAN_POINT('Ctrl Pts',(6.38935290488262,23.4730384757729,4.92330089590042));
#451100=CARTESIAN_POINT('Origin',(5.65685387860011,26.,5.65685387860011));
#451101=CARTESIAN_POINT('',(6.39152331859132,23.9230384757729,4.92169483493571));
#451102=CARTESIAN_POINT('',(6.39146732321148,23.8019615242271,4.92356615355223));
#451103=CARTESIAN_POINT('',(6.39065394077645,26.,4.92305381642377));
#451104=CARTESIAN_POINT('Ctrl Pts',(6.39146732321148,23.8019615242271,4.92356615355223));
#451105=CARTESIAN_POINT('Ctrl Pts',(6.44404636753914,23.7968727736498,4.97518123721477));
#451106=CARTESIAN_POINT('Ctrl Pts',(6.49097569651667,23.7917840230725,5.03225965778749));
#451107=CARTESIAN_POINT('Ctrl Pts',(6.53072214720976,23.7866952724952,5.09396482100832));
#451108=CARTESIAN_POINT('Ctrl Pts',(6.71683190058211,23.7628675822638,5.38289458727869));
#451109=CARTESIAN_POINT('Ctrl Pts',(6.74545633697037,23.7390398920324,5.77326614382955));
#451110=CARTESIAN_POINT('Ctrl Pts',(6.60348277515141,23.715212201801,6.08625298439034));
#451111=CARTESIAN_POINT('Ctrl Pts',(6.46150921333244,23.6913845115696,6.39923982495114));
#451112=CARTESIAN_POINT('Ctrl Pts',(6.14893765330626,23.6675568213382,6.63484194952187));
#451113=CARTESIAN_POINT('Ctrl Pts',(5.80895502137127,23.6437291311068,6.68513161677842));
#451114=CARTESIAN_POINT('Ctrl Pts',(5.4689723894363,23.6199014408755,6.73542128403497));
#451115=CARTESIAN_POINT('Ctrl Pts',(5.10157868559252,23.5960737506441,6.60039849397735));
#451116=CARTESIAN_POINT('Ctrl Pts',(4.87507434314934,23.5722460604127,6.34191631672375));
#451117=CARTESIAN_POINT('Ctrl Pts',(4.64857000070616,23.5484183701813,6.08343413947014));
#451118=CARTESIAN_POINT('Ctrl Pts',(4.56295501966359,23.5245906799499,5.70149257502055));
#451119=CARTESIAN_POINT('Ctrl Pts',(4.65744921450722,23.5007629897185,5.37105630657982));
#451120=CARTESIAN_POINT('Ctrl Pts',(4.75194340935084,23.4769352994871,5.0406200381391));
#451121=CARTESIAN_POINT('Ctrl Pts',(5.02654678008064,23.4531076092557,4.76168906570723));
#451122=CARTESIAN_POINT('Ctrl Pts',(5.35546505814245,23.4292799190243,4.66203997694959));
#451123=CARTESIAN_POINT('Ctrl Pts',(5.68438333620426,23.4054522287929,4.56239088819196));
#451124=CARTESIAN_POINT('Ctrl Pts',(6.06761652159808,23.3816245385615,4.64202368310855));
#451125=CARTESIAN_POINT('Ctrl Pts',(6.32960882821811,23.3577968483301,4.86445867565572));
#451126=CARTESIAN_POINT('Ctrl Pts',(6.350995850443,23.3558517402958,4.88261654521522));
#451127=CARTESIAN_POINT('Ctrl Pts',(6.37157494470415,23.3539066322614,4.90172602358781));
#451128=CARTESIAN_POINT('Ctrl Pts',(6.39131103572319,23.3519615242271,4.92169609601798));
#451129=CARTESIAN_POINT('Ctrl Pts',(6.38935290488262,23.4730384757729,4.92330089590042));
#451130=CARTESIAN_POINT('Ctrl Pts',(6.30414930262285,23.4813898257499,4.83695933636888));
#451131=CARTESIAN_POINT('Ctrl Pts',(6.20464951053553,23.4897411757268,4.76527121936352));
#451132=CARTESIAN_POINT('Ctrl Pts',(6.09544017298549,23.4980925257038,4.71444637045848));
#451133=CARTESIAN_POINT('Ctrl Pts',(5.78384908020389,23.5219202159352,4.56943523344352));
#451134=CARTESIAN_POINT('Ctrl Pts',(5.39321753403733,23.5457479061666,4.59426131240048));
#451135=CARTESIAN_POINT('Ctrl Pts',(5.10249121190879,23.569575596398,4.77755195197114));
#451136=CARTESIAN_POINT('Ctrl Pts',(4.81176488978025,23.5934032866293,4.9608425915418));
#451137=CARTESIAN_POINT('Ctrl Pts',(4.62094379168974,23.6172309768607,5.30259779172617));
#451138=CARTESIAN_POINT('Ctrl Pts',(4.61744171997954,23.6410586670921,5.64626184853499));
#451139=CARTESIAN_POINT('Ctrl Pts',(4.61393964826934,23.6648863573235,5.98992590534381));
#451140=CARTESIAN_POINT('Ctrl Pts',(4.79775660293946,23.6887140475549,6.33549881877709));
#451141=CARTESIAN_POINT('Ctrl Pts',(5.08468731748426,23.7125417377863,6.52467601704459));
#451142=CARTESIAN_POINT('Ctrl Pts',(5.37161803202905,23.7363694280177,6.71385321531209));
#451143=CARTESIAN_POINT('Ctrl Pts',(5.76166250644851,23.7601971182491,6.74663469841383));
#451144=CARTESIAN_POINT('Ctrl Pts',(6.07614404554655,23.7840248084805,6.60800349462427));
#451145=CARTESIAN_POINT('Ctrl Pts',(6.39062558464459,23.8078524987119,6.46937229083472));
#451146=CARTESIAN_POINT('Ctrl Pts',(6.6295441884212,23.8316801889433,6.15932840015388));
#451147=CARTESIAN_POINT('Ctrl Pts',(6.6834528935629,23.8555078791747,5.81990079386588));
#451148=CARTESIAN_POINT('Ctrl Pts',(6.73438085433327,23.8780180780408,5.49924097144978));
#451149=CARTESIAN_POINT('Ctrl Pts',(6.62019259508592,23.9005282769068,5.15235699515366));
#451150=CARTESIAN_POINT('Ctrl Pts',(6.39152331859132,23.9230384757729,4.92169483493571));
#451151=CARTESIAN_POINT('Origin',(5.65685387860011,26.,5.65685387860011));
#451152=CARTESIAN_POINT('',(6.39128196913613,24.3730384757729,4.92377157353716));
#451153=CARTESIAN_POINT('',(6.38942086037359,24.2519615242271,4.92421628016771));
#451154=CARTESIAN_POINT('',(6.39065394077645,26.,4.92305381642377));
#451155=CARTESIAN_POINT('Ctrl Pts',(6.38942086037359,24.2519615242271,4.92421628016771));
#451156=CARTESIAN_POINT('Ctrl Pts',(6.51405309196749,24.2398389150381,5.04895543667044));
#451157=CARTESIAN_POINT('Ctrl Pts',(6.60860369693141,24.2277163058492,5.20382475542584));
#451158=CARTESIAN_POINT('Ctrl Pts',(6.65652287894995,24.2155936966603,5.37198243345446));
#451159=CARTESIAN_POINT('Ctrl Pts',(6.75071080561528,24.1917660064289,5.70250608555364));
#451160=CARTESIAN_POINT('Ctrl Pts',(6.66474206054895,24.1679383161975,6.08436822205294));
#451161=CARTESIAN_POINT('Ctrl Pts',(6.4379983333991,24.1441106259661,6.34264042812557));
#451162=CARTESIAN_POINT('Ctrl Pts',(6.21125460624925,24.1202829357347,6.60091263419821));
#451163=CARTESIAN_POINT('Ctrl Pts',(5.84373589701588,24.0964552455033,6.73559490984418));
#451164=CARTESIAN_POINT('Ctrl Pts',(5.50379999638241,24.0726275552719,6.68499023152592));
#451165=CARTESIAN_POINT('Ctrl Pts',(5.16386409574894,24.0487998650405,6.63438555320766));
#451166=CARTESIAN_POINT('Ctrl Pts',(4.85151100371537,24.0249721748091,6.39849392092517));
#451167=CARTESIAN_POINT('Ctrl Pts',(4.70982751913656,24.0011444845777,6.08537566804496));
#451168=CARTESIAN_POINT('Ctrl Pts',(4.56814403455774,23.9773167943464,5.77225741516475));
#451169=CARTESIAN_POINT('Ctrl Pts',(4.59713015743369,23.9534891041149,5.38191254168682));
#451170=CARTESIAN_POINT('Ctrl Pts',(4.78350754767415,23.9296614138835,5.09315534403941));
#451171=CARTESIAN_POINT('Ctrl Pts',(4.96988493791459,23.9058337236522,4.804398146392));
#451172=CARTESIAN_POINT('Ctrl Pts',(5.31365359551954,23.8820060334208,4.61722862457511));
#451173=CARTESIAN_POINT('Ctrl Pts',(5.65733545950024,23.8581783431894,4.6173878516616));
#451174=CARTESIAN_POINT('Ctrl Pts',(5.92761905169082,23.8394394035353,4.61751307348277));
#451175=CARTESIAN_POINT('Ctrl Pts',(6.19784896370209,23.8207004638812,4.73349750638545));
#451176=CARTESIAN_POINT('Ctrl Pts',(6.39146732321148,23.8019615242271,4.92356615355223));
#451177=CARTESIAN_POINT('Ctrl Pts',(6.39152331859132,23.9230384757729,4.92169483493571));
#451178=CARTESIAN_POINT('Ctrl Pts',(6.37813961642664,23.9243559671382,4.90819449199352));
#451179=CARTESIAN_POINT('Ctrl Pts',(6.3643637478711,23.9256734585035,4.895092278726));
#451180=CARTESIAN_POINT('Ctrl Pts',(6.35020586507153,23.9269909498688,4.88241675495565));
#451181=CARTESIAN_POINT('Ctrl Pts',(6.09415132493169,23.9508186401002,4.65317164422858));
#451182=CARTESIAN_POINT('Ctrl Pts',(5.71314343814525,23.9746463303316,4.56349274466962));
#451183=CARTESIAN_POINT('Ctrl Pts',(5.38171929489583,23.998474020563,4.6544613426263));
#451184=CARTESIAN_POINT('Ctrl Pts',(5.05029515164641,24.0223017107944,4.74542994058297));
#451185=CARTESIAN_POINT('Ctrl Pts',(4.768454751934,24.0461294010258,5.01704603605528));
#451186=CARTESIAN_POINT('Ctrl Pts',(4.6653072414873,24.0699570912572,5.34488416612327));
#451187=CARTESIAN_POINT('Ctrl Pts',(4.56215973104059,24.0937847814886,5.67272229619127));
#451188=CARTESIAN_POINT('Ctrl Pts',(4.63770510985958,24.11761247172,6.05678246085496));
#451189=CARTESIAN_POINT('Ctrl Pts',(4.8573365604447,24.1414401619514,6.32112934350159));
#451190=CARTESIAN_POINT('Ctrl Pts',(5.07696801102981,24.1652678521828,6.58547622614821));
#451191=CARTESIAN_POINT('Ctrl Pts',(5.44068553338104,24.1890955424141,6.73010982677778));
#451192=CARTESIAN_POINT('Ctrl Pts',(5.78187263496817,24.2129232326455,6.68877448884912));
#451193=CARTESIAN_POINT('Ctrl Pts',(6.12305973655531,24.2367509228769,6.64743915092045));
#451194=CARTESIAN_POINT('Ctrl Pts',(6.44171641737836,24.2605786131083,6.42013487443355));
#451195=CARTESIAN_POINT('Ctrl Pts',(6.59186824658804,24.2844063033397,6.11098818332588));
#451196=CARTESIAN_POINT('Ctrl Pts',(6.74202007579772,24.3082339935711,5.80184149221821));
#451197=CARTESIAN_POINT('Ctrl Pts',(6.72366705339403,24.3320616838025,5.41085238648978));
#451198=CARTESIAN_POINT('Ctrl Pts',(6.54521657215205,24.3558893740339,5.11713028264445));
#451199=CARTESIAN_POINT('Ctrl Pts',(6.50240552012982,24.3616057412803,5.04666506349635));
#451200=CARTESIAN_POINT('Ctrl Pts',(6.45038020112141,24.3673221085266,4.98179796021343));
#451201=CARTESIAN_POINT('Ctrl Pts',(6.39128196913613,24.3730384757729,4.92377157353716));
#451202=CARTESIAN_POINT('Origin',(5.65685387860011,26.,5.65685387860011));
#451203=CARTESIAN_POINT('',(6.38933869113556,24.8230384757729,4.92408802232565));
#451204=CARTESIAN_POINT('',(6.39028821611916,24.7019615242271,4.92212745780798));
#451205=CARTESIAN_POINT('',(6.39065394077645,26.,4.92305381642377));
#451206=CARTESIAN_POINT('Ctrl Pts',(6.39028821611916,24.7019615242271,4.92212745780798));
#451207=CARTESIAN_POINT('Ctrl Pts',(6.5845155347103,24.6828050564265,5.11995795053563));
#451208=CARTESIAN_POINT('Ctrl Pts',(6.70087353526984,24.6636485886259,5.39828521249021));
#451209=CARTESIAN_POINT('Ctrl Pts',(6.69616935490973,24.6444921208254,5.67455106061111));
#451210=CARTESIAN_POINT('Ctrl Pts',(6.69031808036474,24.620664430594,6.01818314973456));
#451211=CARTESIAN_POINT('Ctrl Pts',(6.49716519325233,24.5968367403626,6.35862591802898));
#451212=CARTESIAN_POINT('Ctrl Pts',(6.20519269912468,24.5730090501312,6.53992487743046));
#451213=CARTESIAN_POINT('Ctrl Pts',(5.91322020499702,24.5491813598998,6.72122383683194));
#451214=CARTESIAN_POINT('Ctrl Pts',(5.52242810385412,24.5253536696684,6.74337898734048));
#451215=CARTESIAN_POINT('Ctrl Pts',(5.21183556708661,24.501525979437,6.59624120723028));
#451216=CARTESIAN_POINT('Ctrl Pts',(4.90124303031911,24.4776982892056,6.44910342712008));
#451217=CARTESIAN_POINT('Ctrl Pts',(4.670850057927,24.4538705989742,6.13267271639114));
#451218=CARTESIAN_POINT('Ctrl Pts',(4.62619808347199,24.4300429087428,5.79190380451131));
#451219=CARTESIAN_POINT('Ctrl Pts',(4.58154610901698,24.4062152185114,5.45113489263147));
#451220=CARTESIAN_POINT('Ctrl Pts',(4.72263513249906,24.38238752828,5.08602777960075));
#451221=CARTESIAN_POINT('Ctrl Pts',(4.98483324415836,24.3585598380486,4.86383551964991));
#451222=CARTESIAN_POINT('Ctrl Pts',(5.24703135581765,24.3347321478172,4.64164325969907));
#451223=CARTESIAN_POINT('Ctrl Pts',(5.63033855565415,24.3109044575858,4.56236585282811));
#451224=CARTESIAN_POINT('Ctrl Pts',(5.9591644547709,24.2870767673545,4.66231973324217));
#451225=CARTESIAN_POINT('Ctrl Pts',(6.12069642705376,24.275371686312,4.71142093690032));
#451226=CARTESIAN_POINT('Ctrl Pts',(6.26908122485669,24.2636666052695,4.80377340246064));
#451227=CARTESIAN_POINT('Ctrl Pts',(6.38942086037359,24.2519615242271,4.92421628016771));
#451228=CARTESIAN_POINT('Ctrl Pts',(6.39128196913613,24.3730384757729,4.92377157353716));
#451229=CARTESIAN_POINT('Ctrl Pts',(6.20403942134221,24.391149798758,4.7399249826062));
#451230=CARTESIAN_POINT('Ctrl Pts',(5.94579686164739,24.4092611217431,4.62474754709557));
#451231=CARTESIAN_POINT('Ctrl Pts',(5.68465923264326,24.4273724447281,4.61775970678068));
#451232=CARTESIAN_POINT('Ctrl Pts',(5.34110031445673,24.4512001349595,4.60856633672445));
#451233=CARTESIAN_POINT('Ctrl Pts',(4.99253041816395,24.4750278251909,4.7866346985742));
#451234=CARTESIAN_POINT('Ctrl Pts',(4.79862701145602,24.4988555154223,5.07039290068915));
#451235=CARTESIAN_POINT('Ctrl Pts',(4.60472360474809,24.5226832056536,5.35415110280411));
#451236=CARTESIAN_POINT('Ctrl Pts',(4.565486687625,24.546510895885,5.7435991451843));
#451237=CARTESIAN_POINT('Ctrl Pts',(4.69889042440694,24.5703385861164,6.06033356407531));
#451238=CARTESIAN_POINT('Ctrl Pts',(4.83229416118888,24.5941662763478,6.37706798296632));
#451239=CARTESIAN_POINT('Ctrl Pts',(5.13833855187584,24.6179939665792,6.62108877836816));
#451240=CARTESIAN_POINT('Ctrl Pts',(5.47682676316715,24.6418216568106,6.68061169925028));
#451241=CARTESIAN_POINT('Ctrl Pts',(5.81531497445846,24.665649347042,6.74013462013239));
#451242=CARTESIAN_POINT('Ctrl Pts',(6.18624700635411,24.6894770372734,6.61515966649478));
#451243=CARTESIAN_POINT('Ctrl Pts',(6.41970146010492,24.7133047275048,6.36293701391879));
#451244=CARTESIAN_POINT('Ctrl Pts',(6.65315591385573,24.7371324177362,6.1107143613428));
#451245=CARTESIAN_POINT('Ctrl Pts',(6.7491327894617,24.7609601079676,5.73124400982843));
#451246=CARTESIAN_POINT('Ctrl Pts',(6.6636657201663,24.784787798199,5.3983586947443));
#451247=CARTESIAN_POINT('Ctrl Pts',(6.61793218802977,24.797538024057,5.22023136007979));
#451248=CARTESIAN_POINT('Ctrl Pts',(6.5202452116208,24.8102882499149,5.05544287282308));
#451249=CARTESIAN_POINT('Ctrl Pts',(6.38933869113556,24.8230384757729,4.92408802232565));
#451250=CARTESIAN_POINT('Origin',(5.65685387860011,26.,5.65685387860011));
#451251=CARTESIAN_POINT('',(6.39051881327128,25.2730384757729,4.92197603118329));
#451252=CARTESIAN_POINT('',(6.39198798715975,25.151961524227,4.92254817630007));
#451253=CARTESIAN_POINT('',(6.39065394077645,26.,4.92305381642377));
#451254=CARTESIAN_POINT('Ctrl Pts',(6.39198798715975,25.151961524227,4.92254817630007));
#451255=CARTESIAN_POINT('Ctrl Pts',(6.41627314991443,25.1495988880462,4.94650751599249));
#451256=CARTESIAN_POINT('Ctrl Pts',(6.43929566708608,25.1472362518654,4.97169983154625));
#451257=CARTESIAN_POINT('Ctrl Pts',(6.46089355482011,25.1448736156846,4.99805942366946));
#451258=CARTESIAN_POINT('Ctrl Pts',(6.67871286308055,25.1210459254532,5.26390153716753));
#451259=CARTESIAN_POINT('Ctrl Pts',(6.75163093056004,25.0972182352218,5.64846913729549));
#451260=CARTESIAN_POINT('Ctrl Pts',(6.64624470558553,25.0733905449904,5.97559449046916));
#451261=CARTESIAN_POINT('Ctrl Pts',(6.54085848061101,25.049562854759,6.30271984364283));
#451262=CARTESIAN_POINT('Ctrl Pts',(6.25716796318248,25.0257351645276,6.57240294986222));
#451263=CARTESIAN_POINT('Ctrl Pts',(5.92512971718013,25.0019074742962,6.66110381706143));
#451264=CARTESIAN_POINT('Ctrl Pts',(5.59309147117778,24.9780797840648,6.74980468426065));
#451265=CARTESIAN_POINT('Ctrl Pts',(5.2127054966016,24.9542520938335,6.65752331243968));
#451266=CARTESIAN_POINT('Ctrl Pts',(4.9582240442926,24.9304244036021,6.42653317184816));
#451267=CARTESIAN_POINT('Ctrl Pts',(4.7037425919836,24.9065967133707,6.19554303125664));
#451268=CARTESIAN_POINT('Ctrl Pts',(4.57516566194178,24.8827690231393,5.82584412189456));
#451269=CARTESIAN_POINT('Ctrl Pts',(4.63139343216518,24.8589413329079,5.48679296352304));
#451270=CARTESIAN_POINT('Ctrl Pts',(4.68762120238858,24.8351136426765,5.14774180515151));
#451271=CARTESIAN_POINT('Ctrl Pts',(4.9286536728772,24.8112859524451,4.83933839777055));
#451272=CARTESIAN_POINT('Ctrl Pts',(5.24407554312886,24.7874582622137,4.70286022094558));
#451273=CARTESIAN_POINT('Ctrl Pts',(5.55949741338051,24.7636305719823,4.56638204412062));
#451274=CARTESIAN_POINT('Ctrl Pts',(5.94930868339519,24.7398028817509,4.60182909785165));
#451275=CARTESIAN_POINT('Ctrl Pts',(6.23493948741374,24.7159751915195,4.79296332969341));
#451276=CARTESIAN_POINT('Ctrl Pts',(6.29093505415592,24.7113039690887,4.83043362171106));
#451277=CARTESIAN_POINT('Ctrl Pts',(6.34292671833546,24.7066327466579,4.87388734148021));
#451278=CARTESIAN_POINT('Ctrl Pts',(6.39028821611916,24.7019615242271,4.92212745780798));
#451279=CARTESIAN_POINT('Ctrl Pts',(6.38933869113556,24.8230384757729,4.92408802232565));
#451280=CARTESIAN_POINT('Ctrl Pts',(6.27560640646284,24.8341159401463,4.80996622614209));
#451281=CARTESIAN_POINT('Ctrl Pts',(6.13679925493306,24.8451934045197,4.72108089883846));
#451282=CARTESIAN_POINT('Ctrl Pts',(5.98520281626299,24.8562708688931,4.67061008310121));
#451283=CARTESIAN_POINT('Ctrl Pts',(5.65911799585187,24.8800985591245,4.56204706519615));
#451284=CARTESIAN_POINT('Ctrl Pts',(5.27385936922642,24.9039262493559,4.63122130803993));
#451285=CARTESIAN_POINT('Ctrl Pts',(5.00591117956891,24.9277539395873,4.84644449237099));
#451286=CARTESIAN_POINT('Ctrl Pts',(4.7379629899114,24.9515816298187,5.06166767670205));
#451287=CARTESIAN_POINT('Ctrl Pts',(4.58732523722183,24.9754093200501,5.42293980252039));
#451288=CARTESIAN_POINT('Ctrl Pts',(4.62300419682159,24.9992370102815,5.7647647438604));
#451289=CARTESIAN_POINT('Ctrl Pts',(4.65868315642135,25.0230647005129,6.10658968520039));
#451290=CARTESIAN_POINT('Ctrl Pts',(4.88067882831044,25.0468923907443,6.42896744206205));
#451291=CARTESIAN_POINT('Ctrl Pts',(5.18729621377842,25.0707200809757,6.58421869570625));
#451292=CARTESIAN_POINT('Ctrl Pts',(5.49391359924639,25.0945477712071,6.73946994935045));
#451293=CARTESIAN_POINT('Ctrl Pts',(5.88515269829325,25.1183754614385,6.72759469977719));
#451294=CARTESIAN_POINT('Ctrl Pts',(6.18179018209155,25.1422031516699,6.5540334824637));
#451295=CARTESIAN_POINT('Ctrl Pts',(6.47842766588984,25.1660308419013,6.38047226515022));
#451296=CARTESIAN_POINT('Ctrl Pts',(6.68046353443956,25.1898585321326,6.0452250800965));
#451297=CARTESIAN_POINT('Ctrl Pts',(6.69534535485932,25.213686222364,5.70186524531576));
#451298=CARTESIAN_POINT('Ctrl Pts',(6.70770170116848,25.2334703068337,5.41677424787487));
#451299=CARTESIAN_POINT('Ctrl Pts',(6.59103501365993,25.2532543913033,5.12609043162756));
#451300=CARTESIAN_POINT('Ctrl Pts',(6.39051881327128,25.2730384757729,4.92197603118329));
#451301=CARTESIAN_POINT('Origin',(5.65685387860011,26.,5.65685387860011));
#451302=CARTESIAN_POINT('',(6.39190058798136,25.7230384757729,4.92276701974739));
#451303=CARTESIAN_POINT('',(6.39006796800885,25.6019615242271,4.92443355077908));
#451304=CARTESIAN_POINT('',(6.39065394077645,26.,4.92305381642377));
#451305=CARTESIAN_POINT('',(5.59475217632209,26.,6.69274404704181));
#451306=CARTESIAN_POINT('Ctrl Pts',(6.39190058798136,25.7230384757729,4.92276701974739));
#451307=CARTESIAN_POINT('Ctrl Pts',(6.17742942344334,25.7438759131544,4.71160994855805));
#451308=CARTESIAN_POINT('Ctrl Pts',(5.86562000134797,25.764713350536,4.59523934827088));
#451309=CARTESIAN_POINT('Ctrl Pts',(5.56615422141076,25.7855507879175,4.62142687258513));
#451310=CARTESIAN_POINT('Ctrl Pts',(5.22371394391399,25.8093784781489,4.65137240791476));
#451311=CARTESIAN_POINT('Ctrl Pts',(4.89741422641509,25.8332061683802,4.86772710302321));
#451312=CARTESIAN_POINT('Ctrl Pts',(4.73725319022189,25.8570338586116,5.17187737628347));
#451313=CARTESIAN_POINT('Ctrl Pts',(4.57709215402869,25.880861548843,5.47602764954372));
#451314=CARTESIAN_POINT('Ctrl Pts',(4.58306979914119,25.9046892390744,5.86797350095578));
#451315=CARTESIAN_POINT('Ctrl Pts',(4.75132533448083,25.9285169293058,6.16698733288025));
#451316=CARTESIAN_POINT('Ctrl Pts',(4.91958086982048,25.9523446195372,6.46600116480472));
#451317=CARTESIAN_POINT('Ctrl Pts',(5.25011429538726,25.9761723097686,6.67208297724159));
#451318=CARTESIAN_POINT('Ctrl Pts',(5.59475217632212,26.,6.69274404704181));
#451319=CARTESIAN_POINT('',(6.69457727933146,26.,5.59444809180803));
#451320=CARTESIAN_POINT('Origin',(5.65685387860011,26.,5.65685387860011));
#451321=CARTESIAN_POINT('Ctrl Pts',(6.69458228414866,26.,5.59444726164187));
#451322=CARTESIAN_POINT('Ctrl Pts',(6.71351646533254,25.9770624644402,5.92484673178863));
#451323=CARTESIAN_POINT('Ctrl Pts',(6.56158375468957,25.9541249288804,6.26627937525033));
#451324=CARTESIAN_POINT('Ctrl Pts',(6.30214239804398,25.9311873933205,6.47167795527827));
#451325=CARTESIAN_POINT('Ctrl Pts',(6.03263270014108,25.9073597030892,6.68504759676004));
#451326=CARTESIAN_POINT('Ctrl Pts',(5.64710810132191,25.8835320128578,6.75161994353754));
#451327=CARTESIAN_POINT('Ctrl Pts',(5.32182159136527,25.8597043226264,6.64083855948586));
#451328=CARTESIAN_POINT('Ctrl Pts',(4.99653508140864,25.835876632395,6.53005717543419));
#451329=CARTESIAN_POINT('Ctrl Pts',(4.73148666031454,25.8120489421636,6.24192206055333));
#451330=CARTESIAN_POINT('Ctrl Pts',(4.64827248224482,25.7882212519322,5.90845611919747));
#451331=CARTESIAN_POINT('Ctrl Pts',(4.56505830417509,25.7643935617008,5.57499017784161));
#451332=CARTESIAN_POINT('Ctrl Pts',(4.66367836912974,25.7405658714694,5.19619341001074));
#451333=CARTESIAN_POINT('Ctrl Pts',(4.89886414913016,25.716738181238,4.94557465216384));
#451334=CARTESIAN_POINT('Ctrl Pts',(5.13404992913058,25.6929104910066,4.69495589431694));
#451335=CARTESIAN_POINT('Ctrl Pts',(5.50580142417677,25.6690828007752,4.572515146454));
#451336=CARTESIAN_POINT('Ctrl Pts',(5.84386841174159,25.6452551105438,4.63434949773116));
#451337=CARTESIAN_POINT('Ctrl Pts',(6.04861804217652,25.6308239151049,4.67179935541582));
#451338=CARTESIAN_POINT('Ctrl Pts',(6.24101187097706,25.616392719666,4.7768430935332));
#451339=CARTESIAN_POINT('Ctrl Pts',(6.39006796800885,25.6019615242271,4.92443355077908));
#451340=CARTESIAN_POINT('Origin',(5.65685387860011,26.993675081176,5.65685387860011));
#451341=CARTESIAN_POINT('',(6.5673434103921,22.756324918824,4.74524035180398));
#451342=CARTESIAN_POINT('',(6.57057146528765,22.718675081176,4.74364038176039));
#451343=CARTESIAN_POINT('',(6.56902162633079,26.993675081176,4.74468613086949));
#451344=CARTESIAN_POINT('',(4.8286920333622,22.5,6.64591806159944));
#451345=CARTESIAN_POINT('Ctrl Pts',(6.57057146528766,22.718675081176,4.74364038176039));
#451346=CARTESIAN_POINT('Ctrl Pts',(6.58852418981576,22.7172664581449,4.76142457130848));
#451347=CARTESIAN_POINT('Ctrl Pts',(6.9000556810006,22.6920301448823,5.09000197050781));
#451348=CARTESIAN_POINT('Ctrl Pts',(7.12689194633153,22.6429661413884,6.06611679986992));
#451349=CARTESIAN_POINT('Ctrl Pts',(6.10694434613243,22.5714830706942,7.11331947438321));
#451350=CARTESIAN_POINT('Ctrl Pts',(5.15775103452081,22.5238276902314,6.92144528650133));
#451351=CARTESIAN_POINT('Ctrl Pts',(4.8286920333622,22.5,6.64591806159944));
#451352=CARTESIAN_POINT('',(4.44194770692244,22.5,6.09734856608929));
#451353=CARTESIAN_POINT('Origin',(5.65685387860011,22.5,5.65685387860011));
#451354=CARTESIAN_POINT('Ctrl Pts',(6.5673434103921,22.756324918824,4.74524035180399));
#451355=CARTESIAN_POINT('Ctrl Pts',(6.75594870135602,22.7414761952386,4.93595953019022));
#451356=CARTESIAN_POINT('Ctrl Pts',(7.10121210146151,22.7027997814218,5.58182921801751));
#451357=CARTESIAN_POINT('Ctrl Pts',(6.68055232418451,22.6402956773736,6.78713386963137));
#451358=CARTESIAN_POINT('Ctrl Pts',(5.27997950888059,22.5697027613511,7.12528591239124));
#451359=CARTESIAN_POINT('Ctrl Pts',(4.58325719964657,22.5229375355598,6.48370144903283));
#451360=CARTESIAN_POINT('Ctrl Pts',(4.44194158662797,22.5,6.09735008669022));
#451361=CARTESIAN_POINT('Origin',(5.65685387860011,26.993675081176,5.65685387860011));
#451362=CARTESIAN_POINT('',(6.56983844394705,23.206324918824,4.74299838399068));
#451363=CARTESIAN_POINT('',(6.56867439792569,23.168675081176,4.74631652959707));
#451364=CARTESIAN_POINT('',(6.56902162633079,26.993675081176,4.74468613086949));
#451365=CARTESIAN_POINT('Ctrl Pts',(6.56867439792569,23.168675081176,4.74631652959707));
#451366=CARTESIAN_POINT('Ctrl Pts',(6.67716702479821,23.1602325995332,4.853408844765));
#451367=CARTESIAN_POINT('Ctrl Pts',(7.02077633180239,23.127962427659,5.33214451040115));
#451368=CARTESIAN_POINT('Ctrl Pts',(6.94377741359718,23.0718645655535,6.47507582842176));
#451369=CARTESIAN_POINT('Ctrl Pts',(5.66653874837814,23.0003814948592,7.18181942856023));
#451370=CARTESIAN_POINT('Ctrl Pts',(4.38054591235378,22.9288984241651,6.49141154940691));
#451371=CARTESIAN_POINT('Ctrl Pts',(4.26365553420012,22.8574153534709,5.03639155729104));
#451372=CARTESIAN_POINT('Ctrl Pts',(5.40079341912851,22.7873409058079,4.16730445086878));
#451373=CARTESIAN_POINT('Ctrl Pts',(6.28484325502835,22.7410941483762,4.46059450521194));
#451374=CARTESIAN_POINT('Ctrl Pts',(6.57057146528766,22.718675081176,4.74364038176039));
#451375=CARTESIAN_POINT('Ctrl Pts',(6.56983844394705,23.206324918824,4.74299838399068));
#451376=CARTESIAN_POINT('Ctrl Pts',(6.84584090104065,23.184442336627,5.02227299078826));
#451377=CARTESIAN_POINT('Ctrl Pts',(7.14533371342118,23.1387320641985,5.88847306909541));
#451378=CARTESIAN_POINT('Ctrl Pts',(6.30845753745629,23.0691941015387,7.03563221165043));
#451379=CARTESIAN_POINT('Ctrl Pts',(4.85119529970875,22.9977110308445,6.95165327175697));
#451380=CARTESIAN_POINT('Ctrl Pts',(4.13204038713623,22.9262279601503,5.68141376558384));
#451381=CARTESIAN_POINT('Ctrl Pts',(4.80994952176022,22.8547448894562,4.38863987327371));
#451382=CARTESIAN_POINT('Ctrl Pts',(5.9617065202947,22.7981105423474,4.28501879514303));
#451383=CARTESIAN_POINT('Ctrl Pts',(6.45329450867431,22.76530388547,4.62991319040622));
#451384=CARTESIAN_POINT('Ctrl Pts',(6.5673434103921,22.756324918824,4.74524035180399));
#451385=CARTESIAN_POINT('Origin',(5.65685387860011,26.993675081176,5.65685387860011));
#451386=CARTESIAN_POINT('',(6.57003272085371,23.656324918824,4.74532300381163));
#451387=CARTESIAN_POINT('',(6.56740434249263,23.618675081176,4.74499326893249));
#451388=CARTESIAN_POINT('',(6.56902162633079,26.993675081176,4.74468613086949));
#451389=CARTESIAN_POINT('Ctrl Pts',(6.56740434249263,23.618675081176,4.74499326893249));
#451390=CARTESIAN_POINT('Ctrl Pts',(6.76368003125862,23.6031987409216,4.94389036502613));
#451391=CARTESIAN_POINT('Ctrl Pts',(7.10715379447204,23.5638947104357,5.60787864620878));
#451392=CARTESIAN_POINT('Ctrl Pts',(6.65070324968042,23.5007629897185,6.81352117024561));
#451393=CARTESIAN_POINT('Ctrl Pts',(5.22331918686542,23.4292799190243,7.11892889768229));
#451394=CARTESIAN_POINT('Ctrl Pts',(4.19313572939823,23.3577968483302,6.08480364614363));
#451395=CARTESIAN_POINT('Ctrl Pts',(4.50398657889369,23.2863137776359,4.65859667867589));
#451396=CARTESIAN_POINT('Ctrl Pts',(5.70962577012502,23.2232731885846,4.20740365817457));
#451397=CARTESIAN_POINT('Ctrl Pts',(6.37096218895919,23.1840602897646,4.55115618731809));
#451398=CARTESIAN_POINT('Ctrl Pts',(6.56867439792569,23.168675081176,4.74631652959707));
#451399=CARTESIAN_POINT('Ctrl Pts',(6.57003272085371,23.656324918824,4.74532300381163));
#451400=CARTESIAN_POINT('Ctrl Pts',(6.63539236159828,23.6512361682467,4.80948437015677));
#451401=CARTESIAN_POINT('Ctrl Pts',(6.9668858368575,23.622319727438,5.21266771861287));
#451402=CARTESIAN_POINT('Ctrl Pts',(7.04564953674368,23.569575596398,6.28682364983267));
#451403=CARTESIAN_POINT('Ctrl Pts',(5.88000083782648,23.4980925257038,7.16543624640093));
#451404=CARTESIAN_POINT('Ctrl Pts',(4.50990820099156,23.4266094550096,6.66190630419616));
#451405=CARTESIAN_POINT('Ctrl Pts',(4.19063094092434,23.3551263843154,5.23756146736659));
#451406=CARTESIAN_POINT('Ctrl Pts',(5.21468783779196,23.2836433136212,4.19736598356862));
#451407=CARTESIAN_POINT('Ctrl Pts',(6.20635078283888,23.2340428251241,4.40342562281452));
#451408=CARTESIAN_POINT('Ctrl Pts',(6.54530502316694,23.2082700268584,4.71817410701172));
#451409=CARTESIAN_POINT('Ctrl Pts',(6.56983844394705,23.206324918824,4.74299838399068));
#451410=CARTESIAN_POINT('Origin',(5.65685387860011,26.993675081176,5.65685387860011));
#451411=CARTESIAN_POINT('',(6.56748881619374,24.106324918824,4.74613115927677));
#451412=CARTESIAN_POINT('',(6.57010232725217,24.068675081176,4.74299681637215));
#451413=CARTESIAN_POINT('',(6.56902162633079,26.993675081176,4.74468613086949));
#451414=CARTESIAN_POINT('Ctrl Pts',(6.57010232725217,24.068675081176,4.74299681637215));
#451415=CARTESIAN_POINT('Ctrl Pts',(6.85435514987614,24.0461648823099,5.02972694085412));
#451416=CARTESIAN_POINT('Ctrl Pts',(7.14655186859909,23.9998269932124,5.91736950865738));
#451417=CARTESIAN_POINT('Ctrl Pts',(6.27199288310558,23.9296614138836,7.0522818436793));
#451418=CARTESIAN_POINT('Ctrl Pts',(4.81743049717126,23.8581783431894,6.93003241982605));
#451419=CARTESIAN_POINT('Ctrl Pts',(4.13193628895796,23.7866952724952,5.64131435190337));
#451420=CARTESIAN_POINT('Ctrl Pts',(4.84355050202496,23.715212201801,4.3668333837381));
#451421=CARTESIAN_POINT('Ctrl Pts',(5.98491025846011,23.6592054713613,4.29429575151249));
#451422=CARTESIAN_POINT('Ctrl Pts',(6.4614899633887,23.627026431153,4.63766432477859));
#451423=CARTESIAN_POINT('Ctrl Pts',(6.56740434249263,23.618675081176,4.74499326893249));
#451424=CARTESIAN_POINT('Ctrl Pts',(6.56748881619374,24.106324918824,4.74613115927677));
#451425=CARTESIAN_POINT('Ctrl Pts',(6.72241589762581,24.0942023096351,4.90119115627847));
#451426=CARTESIAN_POINT('Ctrl Pts',(7.07096798466868,24.0582520102147,5.47210261995128));
#451427=CARTESIAN_POINT('Ctrl Pts',(6.80286792203874,23.998474020563,6.662968703113));
#451428=CARTESIAN_POINT('Ctrl Pts',(5.43230911237055,23.9269909498688,7.16522879152533));
#451429=CARTESIAN_POINT('Ctrl Pts',(4.26747512907024,23.8555078791747,6.2855365564656));
#451430=CARTESIAN_POINT('Ctrl Pts',(4.37557081254884,23.7840248084805,4.82985391579145));
#451431=CARTESIAN_POINT('Ctrl Pts',(5.56629788826614,23.7176304883636,4.18154636230721));
#451432=CARTESIAN_POINT('Ctrl Pts',(6.32935078034095,23.6750638584781,4.50905361827065));
#451433=CARTESIAN_POINT('Ctrl Pts',(6.57003272085371,23.656324918824,4.74532300381163));
#451434=CARTESIAN_POINT('Origin',(5.65685387860011,26.993675081176,5.65685387860011));
#451435=CARTESIAN_POINT('',(6.56856700353347,24.556324918824,4.74353459859835));
#451436=CARTESIAN_POINT('',(6.56980231202958,24.518675081176,4.74557835604531));
#451437=CARTESIAN_POINT('',(6.56902162633079,26.993675081176,4.74468613086949));
#451438=CARTESIAN_POINT('Ctrl Pts',(6.56980231202958,24.518675081176,4.74557835604531));
#451439=CARTESIAN_POINT('Ctrl Pts',(6.64326578517921,24.5129587139297,4.81770944620421));
#451440=CARTESIAN_POINT('Ctrl Pts',(6.97750833641272,24.4834146564519,5.23445549419879));
#451441=CARTESIAN_POINT('Ctrl Pts',(7.0286098827299,24.4300429087428,6.32311258055822));
#451442=CARTESIAN_POINT('Ctrl Pts',(5.84026841822956,24.3585598380486,7.17078066054311));
#451443=CARTESIAN_POINT('Ctrl Pts',(4.4838850778304,24.2870767673545,6.63140987332417));
#451444=CARTESIAN_POINT('Ctrl Pts',(4.2021595986403,24.2155936966603,5.19916430623342));
#451445=CARTESIAN_POINT('Ctrl Pts',(5.25320498229437,24.1441106259661,4.18624762160046));
#451446=CARTESIAN_POINT('Ctrl Pts',(6.22663461042285,24.095137754138,4.41536649518845));
#451447=CARTESIAN_POINT('Ctrl Pts',(6.55346539562852,24.0699925725413,4.72621489163553));
#451448=CARTESIAN_POINT('Ctrl Pts',(6.57010232725217,24.068675081176,4.74299681637215));
#451449=CARTESIAN_POINT('Ctrl Pts',(6.56856700353347,24.556324918824,4.74353459859835));
#451450=CARTESIAN_POINT('Ctrl Pts',(6.81000592522228,24.5371684510234,4.9894525322227));
#451451=CARTESIAN_POINT('Ctrl Pts',(7.13455935910424,24.4941842929914,5.76578134653658));
#451452=CARTESIAN_POINT('Ctrl Pts',(6.46131966662841,24.4273724447281,6.95240396480877));
#451453=CARTESIAN_POINT('Ctrl Pts',(5.00396921476326,24.3558893740339,7.03502543671246));
#451454=CARTESIAN_POINT('Ctrl Pts',(4.14478270244581,24.2844063033397,5.85498510857851));
#451455=CARTESIAN_POINT('Ctrl Pts',(4.67093497503136,24.2129232326456,4.49341967622111));
#451456=CARTESIAN_POINT('Ctrl Pts',(5.85795834238072,24.1535627711403,4.24791389261248));
#451457=CARTESIAN_POINT('Ctrl Pts',(6.41789774915756,24.1180299998665,4.59641175456261));
#451458=CARTESIAN_POINT('Ctrl Pts',(6.56748881619374,24.106324918824,4.74613115927677));
#451459=CARTESIAN_POINT('Origin',(5.65685387860011,26.993675081176,5.65685387860011));
#451460=CARTESIAN_POINT('',(6.57067994464873,25.006324918824,4.74405758279954));
#451461=CARTESIAN_POINT('',(6.56738667375376,24.968675081176,4.74597172529336));
#451462=CARTESIAN_POINT('',(6.56902162633079,26.993675081176,4.74468613086949));
#451463=CARTESIAN_POINT('Ctrl Pts',(6.56738667375376,24.968675081176,4.74597172529336));
#451464=CARTESIAN_POINT('Ctrl Pts',(6.73011316031215,24.955924855318,4.90925551921452));
#451465=CARTESIAN_POINT('Ctrl Pts',(7.07847832230359,24.9193469392286,5.49691387622178));
#451466=CARTESIAN_POINT('Ctrl Pts',(6.77602463836695,24.8589413329079,6.69274573713214));
#451467=CARTESIAN_POINT('Ctrl Pts',(5.39273679116275,24.7874582622137,7.15880506797054));
#451468=CARTESIAN_POINT('Ctrl Pts',(4.25142935492228,24.7159751915195,6.24879737998678));
#451469=CARTESIAN_POINT('Ctrl Pts',(4.39775252453571,24.6444921208253,4.79645922145989));
#451470=CARTESIAN_POINT('Ctrl Pts',(5.59369688000734,24.5787254173775,4.18550614000559));
#451471=CARTESIAN_POINT('Ctrl Pts',(6.33704597702196,24.5367864041611,4.51704344657683));
#451472=CARTESIAN_POINT('Ctrl Pts',(6.56980231202958,24.518675081176,4.74557835604531));
#451473=CARTESIAN_POINT('Ctrl Pts',(6.57067994464873,25.006324918824,4.74405758279954));
#451474=CARTESIAN_POINT('Ctrl Pts',(6.60086819803686,25.0039622826432,4.77384081402403));
#451475=CARTESIAN_POINT('Ctrl Pts',(6.918112503001,24.9777719562309,5.12098437694123));
#451476=CARTESIAN_POINT('Ctrl Pts',(7.10838527255517,24.9277539395874,6.12447699388039));
#451477=CARTESIAN_POINT('Ctrl Pts',(6.05044038944422,24.8562708688931,7.13018513270865));
#451478=CARTESIAN_POINT('Ctrl Pts',(4.63189669239788,24.784787798199,6.78604742232837));
#451479=CARTESIAN_POINT('Ctrl Pts',(4.15240479236238,24.7133047275048,5.40735816264999));
#451480=CARTESIAN_POINT('Ctrl Pts',(5.0512683537124,24.6418216568106,4.25725342975252));
#451481=CARTESIAN_POINT('Ctrl Pts',(6.11539165852711,24.589495053917,4.35401829743014));
#451482=CARTESIAN_POINT('Ctrl Pts',(6.50969315902277,24.5609961412548,4.68356856625642));
#451483=CARTESIAN_POINT('Ctrl Pts',(6.56856700353347,24.556324918824,4.74353459859835));
#451484=CARTESIAN_POINT('Origin',(5.65685387860011,26.993675081176,5.65685387860011));
#451485=CARTESIAN_POINT('',(6.56829321884323,25.456324918824,4.74640124271564));
#451486=CARTESIAN_POINT('',(6.56885365284802,25.418675081176,4.74334636410459));
#451487=CARTESIAN_POINT('',(6.56902162633079,26.993675081176,4.74468613086949));
#451488=CARTESIAN_POINT('Ctrl Pts',(6.56885365284802,25.418675081176,4.74334636410459));
#451489=CARTESIAN_POINT('Ctrl Pts',(6.81811011972481,25.3988909967064,4.99707565976646));
#451490=CARTESIAN_POINT('Ctrl Pts',(7.13780202337966,25.3552792220053,5.79361205385018));
#451491=CARTESIAN_POINT('Ctrl Pts',(6.42698533143036,25.287839757073,6.97310209577086));
#451492=CARTESIAN_POINT('Ctrl Pts',(4.96796792520407,25.2163566863788,7.01738753624157));
#451493=CARTESIAN_POINT('Ctrl Pts',(4.14009680960707,25.1448736156846,5.81516935358237));
#451494=CARTESIAN_POINT('Ctrl Pts',(4.70185841202445,25.0733905449904,4.4679054394248));
#451495=CARTESIAN_POINT('Ctrl Pts',(5.88231068328695,25.0146577001542,4.25595199715398));
#451496=CARTESIAN_POINT('Ctrl Pts',(6.4260090324839,24.9797525455494,4.604109892408));
#451497=CARTESIAN_POINT('Ctrl Pts',(6.56738667375376,24.968675081176,4.74597172529336));
#451498=CARTESIAN_POINT('Ctrl Pts',(6.56829321884323,25.456324918824,4.74640124271564));
#451499=CARTESIAN_POINT('Ctrl Pts',(6.68893848409317,25.4469284240315,4.86586022639608));
#451500=CARTESIAN_POINT('Ctrl Pts',(7.03476003379299,25.4137042390077,5.36752678600608));
#451501=CARTESIAN_POINT('Ctrl Pts',(6.91003560334641,25.3566523637524,6.5258341885166));
#451502=CARTESIAN_POINT('Ctrl Pts',(5.60564496305,25.2851692930582,7.18099123031483));
#451503=CARTESIAN_POINT('Ctrl Pts',(4.34815567114858,25.213686222364,6.43975200870338));
#451504=CARTESIAN_POINT('Ctrl Pts',(4.28968558428151,25.1422031516699,4.98123363545819));
#451505=CARTESIAN_POINT('Ctrl Pts',(5.44432497425889,25.0730827171565,4.16945626611646));
#451506=CARTESIAN_POINT('Ctrl Pts',(6.29641321838457,25.0277899728745,4.47347056935133));
#451507=CARTESIAN_POINT('Ctrl Pts',(6.57067994464873,25.006324918824,4.74405758279954));
#451508=CARTESIAN_POINT('Origin',(5.65685387860011,26.993675081176,5.65685387860011));
#451509=CARTESIAN_POINT('',(6.56704169373441,25.906324918824,4.7445060113485));
#451510=CARTESIAN_POINT('',(6.57057130100612,25.868675081176,4.74432962138981));
#451511=CARTESIAN_POINT('',(6.56902162633079,26.993675081176,4.74468613086949));
#451512=CARTESIAN_POINT('',(5.01302286563433,26.,4.53900700771688));
#451513=CARTESIAN_POINT('Ctrl Pts',(5.01302286563431,26.,4.53900700771688));
#451514=CARTESIAN_POINT('Ctrl Pts',(5.38492752167559,25.9761723097686,4.32480615636363));
#451515=CARTESIAN_POINT('Ctrl Pts',(6.01924597306242,25.9449472827099,4.30899334914827));
#451516=CARTESIAN_POINT('Ctrl Pts',(6.47338425157137,25.9137222556513,4.64940368207851));
#451517=CARTESIAN_POINT('Ctrl Pts',(6.56704169373441,25.906324918824,4.74450601134849));
#451518=CARTESIAN_POINT('',(4.5368959669337,26.,5.01208503488093));
#451519=CARTESIAN_POINT('Origin',(5.65685387860011,26.,5.65685387860011));
#451520=CARTESIAN_POINT('Ctrl Pts',(4.5368902045627,26.,5.01208247494518));
#451521=CARTESIAN_POINT('Ctrl Pts',(4.74314812622022,25.9770624644402,4.65613984562121));
#451522=CARTESIAN_POINT('Ctrl Pts',(5.48969900651177,25.9332874914989,4.17795197796788));
#451523=CARTESIAN_POINT('Ctrl Pts',(6.3039677816093,25.8895125185575,4.48184576512937));
#451524=CARTESIAN_POINT('Ctrl Pts',(6.57057130100612,25.868675081176,4.74432962138981));
#451525=CARTESIAN_POINT('Origin',(0.,25.85,0.));
#451526=CARTESIAN_POINT('',(-1.69705627484771,26.,-1.69705627484771));
#451527=CARTESIAN_POINT('Origin',(0.,26.,0.));
#451528=CARTESIAN_POINT('',(-1.48492424049175,25.7,-1.48492424049175));
#451529=CARTESIAN_POINT('',(-1.59099025766973,25.85,-1.59099025766973));
#451530=CARTESIAN_POINT('Origin',(0.,25.7,0.));
#451531=CARTESIAN_POINT('Origin',(0.,0.,0.));
#451532=CARTESIAN_POINT('',(-1.48492424049175,14.7,-1.48492424049175));
#451533=CARTESIAN_POINT('',(1.48492424049174,14.7,1.48492424049174));
#451534=CARTESIAN_POINT('Origin',(0.,14.7,0.));
#451535=CARTESIAN_POINT('Origin',(0.,14.7,0.));
#451536=CARTESIAN_POINT('',(-1.48492424049175,0.,-1.48492424049175));
#451537=CARTESIAN_POINT('Origin',(7.88424061023,26.,-7.88424061023001));
#451538=CARTESIAN_POINT('',(7.42462120245875,26.,7.42462120245875));
#451539=CARTESIAN_POINT('Origin',(0.,26.,0.));
#451540=CARTESIAN_POINT('Ctrl Pts',(5.01302286563431,26.,4.53900700771688));
#451541=CARTESIAN_POINT('Ctrl Pts',(5.06076150603835,26.,4.51730428611638));
#451542=CARTESIAN_POINT('Ctrl Pts',(5.10974961966388,26.,4.49883681289365));
#451543=CARTESIAN_POINT('Ctrl Pts',(5.15967019073111,26.,4.48353831525793));
#451544=CARTESIAN_POINT('Ctrl Pts',(5.21017178076232,26.,4.46806176041941));
#451545=CARTESIAN_POINT('Ctrl Pts',(5.26162887990441,26.,4.45582849042794));
#451546=CARTESIAN_POINT('Ctrl Pts',(5.31372001428672,26.,4.44682362697332));
#451547=CARTESIAN_POINT('Ctrl Pts',(5.3513943575585,26.,4.44031095795722));
#451548=CARTESIAN_POINT('Ctrl Pts',(5.38940054503647,26.,4.43548811807628));
#451549=CARTESIAN_POINT('Ctrl Pts',(5.42761365593421,26.,4.43236615256964));
#451550=CARTESIAN_POINT('Ctrl Pts',(5.44398133170966,26.,4.43102893301346));
#451551=CARTESIAN_POINT('Ctrl Pts',(5.46038690933068,26.,4.43000393185805));
#451552=CARTESIAN_POINT('Ctrl Pts',(5.47682022646822,26.,4.42929277127865));
#451553=CARTESIAN_POINT('Ctrl Pts',(5.48697840403902,26.,4.4288531707168));
#451554=CARTESIAN_POINT('Ctrl Pts',(5.49714835620506,26.,4.42853358462936));
#451555=CARTESIAN_POINT('Ctrl Pts',(5.50731025736073,26.,4.42833449334039));
#451556=CARTESIAN_POINT('Ctrl Pts',(5.55884880603531,26.,4.42732475353579));
#451557=CARTESIAN_POINT('Ctrl Pts',(5.610283939002,26.,4.42940473009374));
#451558=CARTESIAN_POINT('Ctrl Pts',(5.66131493500104,26.,4.43455229706354));
#451559=CARTESIAN_POINT('Ctrl Pts',(5.7111818931385,26.,4.43958244592831));
#451560=CARTESIAN_POINT('Ctrl Pts',(5.7606639397111,26.,4.44754223428516));
#451561=CARTESIAN_POINT('Ctrl Pts',(5.8094641568765,26.,4.45845673165193));
#451562=CARTESIAN_POINT('Ctrl Pts',(5.84341695883143,26.,4.46605050457051));
#451563=CARTESIAN_POINT('Ctrl Pts',(5.87703937804619,26.,4.47507550289033));
#451564=CARTESIAN_POINT('Ctrl Pts',(5.91022284171251,26.,4.48555225878239));
#451565=CARTESIAN_POINT('Ctrl Pts',(5.92194029467554,26.,4.48925171871836));
#451566=CARTESIAN_POINT('Ctrl Pts',(5.93360293686827,26.,4.49313228200365));
#451567=CARTESIAN_POINT('Ctrl Pts',(5.94520571051292,26.,4.49719513441307));
#451568=CARTESIAN_POINT('Ctrl Pts',(5.95377453080572,26.,4.50019561112999));
#451569=CARTESIAN_POINT('Ctrl Pts',(5.96230961480298,26.,4.50329523558675));
#451570=CARTESIAN_POINT('Ctrl Pts',(5.97079740732734,26.,4.50648983134838));
#451571=CARTESIAN_POINT('Ctrl Pts',(6.01606106262497,26.,4.52352595481099));
#451572=CARTESIAN_POINT('Ctrl Pts',(6.06007213708863,26.,4.54329052845224));
#451573=CARTESIAN_POINT('Ctrl Pts',(6.10256102519025,26.,4.56579698909369));
#451574=CARTESIAN_POINT('Ctrl Pts',(6.13297429945773,26.,4.58190696962887));
#451575=CARTESIAN_POINT('Ctrl Pts',(6.16260727981828,26.,4.59942271299404));
#451576=CARTESIAN_POINT('Ctrl Pts',(6.1913507700685,26.,4.61836202894701));
#451577=CARTESIAN_POINT('Ctrl Pts',(6.22965595338923,26.,4.64360162105055));
#451578=CARTESIAN_POINT('Ctrl Pts',(6.26638275459849,26.,4.67136946042345));
#451579=CARTESIAN_POINT('Ctrl Pts',(6.30137698491027,26.,4.70144469586272));
#451580=CARTESIAN_POINT('Ctrl Pts',(6.31060442836129,26.,4.70937507558016));
#451581=CARTESIAN_POINT('Ctrl Pts',(6.31971121578836,26.,4.71746597339334));
#451582=CARTESIAN_POINT('Ctrl Pts',(6.32869409556115,26.,4.72571349227114));
#451583=CARTESIAN_POINT('Ctrl Pts',(6.33546837134763,26.,4.73193320898177));
#451584=CARTESIAN_POINT('Ctrl Pts',(6.34217214625841,26.,4.73824213429014));
#451585=CARTESIAN_POINT('Ctrl Pts',(6.34879370706907,26.,4.74462823868481));
#451586=CARTESIAN_POINT('Ctrl Pts',(6.38351694987569,26.,4.77811675594305));
#451587=CARTESIAN_POINT('Ctrl Pts',(6.41605753628304,26.,4.81379250852091));
#451588=CARTESIAN_POINT('Ctrl Pts',(6.4462758017894,26.,4.85136909773308));
#451589=CARTESIAN_POINT('Ctrl Pts',(6.47641151646928,26.,4.88884303451155));
#451590=CARTESIAN_POINT('Ctrl Pts',(6.50423803830034,26.,4.92820865020386));
#451591=CARTESIAN_POINT('Ctrl Pts',(6.52957020070414,26.,4.96920312732197));
#451592=CARTESIAN_POINT('Ctrl Pts',(6.54313464053154,26.,4.9911541597392));
#451593=CARTESIAN_POINT('Ctrl Pts',(6.55598305842118,26.,5.0135724729987));
#451594=CARTESIAN_POINT('Ctrl Pts',(6.56808081878415,26.,5.03641841923856));
#451595=CARTESIAN_POINT('Ctrl Pts',(6.57436456839788,26.,5.04828493019204));
#451596=CARTESIAN_POINT('Ctrl Pts',(6.58044572293647,26.,5.06026681279699));
#451597=CARTESIAN_POINT('Ctrl Pts',(6.58631893168823,26.,5.07235847248556));
#451598=CARTESIAN_POINT('Ctrl Pts',(6.59081778530665,26.,5.0816206338086));
#451599=CARTESIAN_POINT('Ctrl Pts',(6.5951946526525,26.,5.09094758402314));
#451600=CARTESIAN_POINT('Ctrl Pts',(6.59944110229676,26.,5.10032287212331));
#451601=CARTESIAN_POINT('Ctrl Pts',(6.6185486795277,26.,5.14250847573184));
#451602=CARTESIAN_POINT('Ctrl Pts',(6.63505331111242,26.,5.18574009205373));
#451603=CARTESIAN_POINT('Ctrl Pts',(6.64877678422558,26.,5.22977562437019));
#451604=CARTESIAN_POINT('Ctrl Pts',(6.65803415466685,26.,5.25948043975257));
#451605=CARTESIAN_POINT('Ctrl Pts',(6.66602500922953,26.,5.28955126506286));
#451606=CARTESIAN_POINT('Ctrl Pts',(6.67268119205899,26.,5.3199128379813));
#451607=CARTESIAN_POINT('Ctrl Pts',(6.67555458049447,26.,5.33301953813398));
#451608=CARTESIAN_POINT('Ctrl Pts',(6.67817927295671,26.,5.34618251321162));
#451609=CARTESIAN_POINT('Ctrl Pts',(6.68054575323313,26.,5.35937322817315));
#451610=CARTESIAN_POINT('Ctrl Pts',(6.68833148242524,26.,5.4027707310232));
#451611=CARTESIAN_POINT('Ctrl Pts',(6.69333871127853,26.,5.44652175704576));
#451612=CARTESIAN_POINT('Ctrl Pts',(6.69538344663679,26.,5.49040691017122));
#451613=CARTESIAN_POINT('Ctrl Pts',(6.69639471249186,26.,5.51211121372355));
#451614=CARTESIAN_POINT('Ctrl Pts',(6.69668059243935,26.,5.53384821037826));
#451615=CARTESIAN_POINT('Ctrl Pts',(6.69621420261903,26.,5.55559016156262));
#451616=CARTESIAN_POINT('Ctrl Pts',(6.69593634735414,26.,5.56854309351446));
#451617=CARTESIAN_POINT('Ctrl Pts',(6.69539142062067,26.,5.58149776570054));
#451618=CARTESIAN_POINT('Ctrl Pts',(6.69458228414866,26.,5.59444726164187));
#451619=CARTESIAN_POINT('Ctrl Pts',(5.59475217632212,26.,6.69274404704181));
#451620=CARTESIAN_POINT('Ctrl Pts',(5.55137724984311,26.,6.69531021368757));
#451621=CARTESIAN_POINT('Ctrl Pts',(5.50802061877154,26.,6.69492058849835));
#451622=CARTESIAN_POINT('Ctrl Pts',(5.4649019749424,26.,6.69178524360462));
#451623=CARTESIAN_POINT('Ctrl Pts',(5.41981030827847,26.,6.6885064316043));
#451624=CARTESIAN_POINT('Ctrl Pts',(5.3749781156863,26.,6.6822250250606));
#451625=CARTESIAN_POINT('Ctrl Pts',(5.33063916085636,26.,6.67312701402814));
#451626=CARTESIAN_POINT('Ctrl Pts',(5.29648485405826,26.,6.66611881409995));
#451627=CARTESIAN_POINT('Ctrl Pts',(5.26262271564401,26.,6.657438192268));
#451628=CARTESIAN_POINT('Ctrl Pts',(5.22915790417526,26.,6.64714921184179));
#451629=CARTESIAN_POINT('Ctrl Pts',(5.2180438660871,26.,6.64373212639213));
#451630=CARTESIAN_POINT('Ctrl Pts',(5.20697366141539,26.,6.64013749916696));
#451631=CARTESIAN_POINT('Ctrl Pts',(5.19595119703594,26.,6.63636725687979));
#451632=CARTESIAN_POINT('Ctrl Pts',(5.18836217076809,26.,6.63377142469848));
#451633=CARTESIAN_POINT('Ctrl Pts',(5.18079825567733,26.,6.63109312202817));
#451634=CARTESIAN_POINT('Ctrl Pts',(5.17326885643069,26.,6.62833627003802));
#451635=CARTESIAN_POINT('Ctrl Pts',(5.1291279008345,26.,6.61217427924751));
#451636=CARTESIAN_POINT('Ctrl Pts',(5.08609247696685,26.,6.59328941999762));
#451637=CARTESIAN_POINT('Ctrl Pts',(5.04440658587507,26.,6.57188267750787));
#451638=CARTESIAN_POINT('Ctrl Pts',(5.00189276334404,26.,6.55005077161978));
#451639=CARTESIAN_POINT('Ctrl Pts',(4.96078147197193,26.,6.52559561372727));
#451640=CARTESIAN_POINT('Ctrl Pts',(4.92133403622236,26.,6.49867698438676));
#451641=CARTESIAN_POINT('Ctrl Pts',(4.89441638666335,26.,6.48030858559407));
#451642=CARTESIAN_POINT('Ctrl Pts',(4.86827351967756,26.,6.46079201260925));
#451643=CARTESIAN_POINT('Ctrl Pts',(4.84299340446309,26.,6.4401650142142));
#451644=CARTESIAN_POINT('Ctrl Pts',(4.83579340555386,26.,6.43429026385467));
#451645=CARTESIAN_POINT('Ctrl Pts',(4.82866342617017,26.,6.42832537837765));
#451646=CARTESIAN_POINT('Ctrl Pts',(4.82160559536045,26.,6.42227108527737));
#451647=CARTESIAN_POINT('Ctrl Pts',(4.81488692701488,26.,6.41650772986347));
#451648=CARTESIAN_POINT('Ctrl Pts',(4.80824066086902,26.,6.41066935775182));
#451649=CARTESIAN_POINT('Ctrl Pts',(4.80166944006503,26.,6.40475816436008));
#451650=CARTESIAN_POINT('Ctrl Pts',(4.76504957872374,26.,6.37181647988102));
#451651=CARTESIAN_POINT('Ctrl Pts',(4.73074760271325,26.,6.3366074009898));
#451652=CARTESIAN_POINT('Ctrl Pts',(4.69903040790721,26.,6.29931177973046));
#451653=CARTESIAN_POINT('Ctrl Pts',(4.67944112167677,26.,6.27627712598951));
#451654=CARTESIAN_POINT('Ctrl Pts',(4.66083800978401,26.,6.25244551905118));
#451655=CARTESIAN_POINT('Ctrl Pts',(4.64328815682614,26.,6.22785054805505));
#451656=CARTESIAN_POINT('Ctrl Pts',(4.61561379199964,26.,6.18906673591271));
#451657=CARTESIAN_POINT('Ctrl Pts',(4.59055615782454,26.,6.14838638392197));
#451658=CARTESIAN_POINT('Ctrl Pts',(4.56810357334095,26.,6.10609561292347));
#451659=CARTESIAN_POINT('Ctrl Pts',(4.56308085571068,26.,6.0966350271612));
#451660=CARTESIAN_POINT('Ctrl Pts',(4.55818866062255,26.,6.08709371894873));
#451661=CARTESIAN_POINT('Ctrl Pts',(4.55342713549933,26.,6.0774746818157));
#451662=CARTESIAN_POINT('Ctrl Pts',(4.54941744651794,26.,6.06937447312086));
#451663=CARTESIAN_POINT('Ctrl Pts',(4.54550147490651,26.,6.06122106951547));
#451664=CARTESIAN_POINT('Ctrl Pts',(4.54168378413803,26.,6.05302670560527));
#451665=CARTESIAN_POINT('Ctrl Pts',(4.52091202527781,26.,6.00844180822155));
#451666=CARTESIAN_POINT('Ctrl Pts',(4.5030051530968,26.,5.9625645247388));
#451667=CARTESIAN_POINT('Ctrl Pts',(4.48791424199878,26.,5.91572767775388));
#451668=CARTESIAN_POINT('Ctrl Pts',(4.4724457898949,26.,5.86771907710826));
#451669=CARTESIAN_POINT('Ctrl Pts',(4.45993552318701,26.,5.81870139486952));
#451670=CARTESIAN_POINT('Ctrl Pts',(4.45037293016505,26.,5.76899658983648));
#451671=CARTESIAN_POINT('Ctrl Pts',(4.44466425311952,26.,5.73932381395939));
#451672=CARTESIAN_POINT('Ctrl Pts',(4.4400069173499,26.,5.70940552486093));
#451673=CARTESIAN_POINT('Ctrl Pts',(4.43640656180746,26.,5.67930640361674));
#451674=CARTESIAN_POINT('Ctrl Pts',(4.4344238827759,26.,5.66273112491008));
#451675=CARTESIAN_POINT('Ctrl Pts',(4.4327618494722,26.,5.6461009688343));
#451676=CARTESIAN_POINT('Ctrl Pts',(4.4314222120057,26.,5.62942654610506));
#451677=CARTESIAN_POINT('Ctrl Pts',(4.4306913632861,26.,5.62032969654203));
#451678=CARTESIAN_POINT('Ctrl Pts',(4.43005669150461,26.,5.61122148290957));
#451679=CARTESIAN_POINT('Ctrl Pts',(4.42951879017363,26.,5.60211289272811));
#451680=CARTESIAN_POINT('Ctrl Pts',(4.4264158896556,26.,5.54956970763969));
#451681=CARTESIAN_POINT('Ctrl Pts',(4.42652201105729,26.,5.4969304712558));
#451682=CARTESIAN_POINT('Ctrl Pts',(4.42983270797829,26.,5.44453981443333));
#451683=CARTESIAN_POINT('Ctrl Pts',(4.43208820455334,26.,5.40884734549178));
#451684=CARTESIAN_POINT('Ctrl Pts',(4.43583203037196,26.,5.37326963814493));
#451685=CARTESIAN_POINT('Ctrl Pts',(4.44107619046014,26.,5.33791219834493));
#451686=CARTESIAN_POINT('Ctrl Pts',(4.44350332623801,26.,5.32154784147763));
#451687=CARTESIAN_POINT('Ctrl Pts',(4.44625314527356,26.,5.3052257211536));
#451688=CARTESIAN_POINT('Ctrl Pts',(4.44932134384721,26.,5.2889864307097));
#451689=CARTESIAN_POINT('Ctrl Pts',(4.45918506317858,26.,5.23677996517828));
#451690=CARTESIAN_POINT('Ctrl Pts',(4.47234120944802,26.,5.18537728352641));
#451691=CARTESIAN_POINT('Ctrl Pts',(4.48880818879318,26.,5.13511946191399));
#451692=CARTESIAN_POINT('Ctrl Pts',(4.49754364477499,26.,5.10845853162224));
#451693=CARTESIAN_POINT('Ctrl Pts',(4.50721166236008,26.,5.08211963725754));
#451694=CARTESIAN_POINT('Ctrl Pts',(4.51782098438608,26.,5.05615381819268));
#451695=CARTESIAN_POINT('Ctrl Pts',(4.52387352626206,26.,5.04134050525441));
#451696=CARTESIAN_POINT('Ctrl Pts',(4.53023250440261,26.,5.02664862375098));
#451697=CARTESIAN_POINT('Ctrl Pts',(4.53689020456271,26.,5.01208247494515));
#451698=CARTESIAN_POINT('Ctrl Pts',(-4.53900700771688,26.,5.01302286563431));
#451699=CARTESIAN_POINT('Ctrl Pts',(-4.51730428611638,26.,5.06076150603835));
#451700=CARTESIAN_POINT('Ctrl Pts',(-4.49883681289365,26.,5.10974961966389));
#451701=CARTESIAN_POINT('Ctrl Pts',(-4.48353831525793,26.,5.15967019073111));
#451702=CARTESIAN_POINT('Ctrl Pts',(-4.46806176041944,26.,5.21017178076222));
#451703=CARTESIAN_POINT('Ctrl Pts',(-4.45582849042799,26.,5.26162887990419));
#451704=CARTESIAN_POINT('Ctrl Pts',(-4.44682362697337,26.,5.3137200142864));
#451705=CARTESIAN_POINT('Ctrl Pts',(-4.44031095795727,26.,5.35139435755819));
#451706=CARTESIAN_POINT('Ctrl Pts',(-4.43548811807631,26.,5.38940054503618));
#451707=CARTESIAN_POINT('Ctrl Pts',(-4.43236615256966,26.,5.42761365593392));
#451708=CARTESIAN_POINT('Ctrl Pts',(-4.43102893301347,26.,5.4439813317094));
#451709=CARTESIAN_POINT('Ctrl Pts',(-4.43000393185806,26.,5.46038690933045));
#451710=CARTESIAN_POINT('Ctrl Pts',(-4.42929277127866,26.,5.47682022646802));
#451711=CARTESIAN_POINT('Ctrl Pts',(-4.42885317071679,26.,5.48697840403927));
#451712=CARTESIAN_POINT('Ctrl Pts',(-4.42853358462933,26.,5.49714835620576));
#451713=CARTESIAN_POINT('Ctrl Pts',(-4.42833449334036,26.,5.50731025736187));
#451714=CARTESIAN_POINT('Ctrl Pts',(-4.42732475353582,26.,5.55884880603616));
#451715=CARTESIAN_POINT('Ctrl Pts',(-4.42940473009378,26.,5.61028393900257));
#451716=CARTESIAN_POINT('Ctrl Pts',(-4.43455229706356,26.,5.66131493500133));
#451717=CARTESIAN_POINT('Ctrl Pts',(-4.43958244592836,26.,5.71118189313887));
#451718=CARTESIAN_POINT('Ctrl Pts',(-4.44754223428524,26.,5.76066393971155));
#451719=CARTESIAN_POINT('Ctrl Pts',(-4.45845673165205,26.,5.80946415687703));
#451720=CARTESIAN_POINT('Ctrl Pts',(-4.46605050457064,26.,5.84341695883192));
#451721=CARTESIAN_POINT('Ctrl Pts',(-4.47507550289046,26.,5.87703937804663));
#451722=CARTESIAN_POINT('Ctrl Pts',(-4.48555225878251,26.,5.9102228417129));
#451723=CARTESIAN_POINT('Ctrl Pts',(-4.48925171871859,26.,5.92194029467625));
#451724=CARTESIAN_POINT('Ctrl Pts',(-4.493132282004,26.,5.9336029368693));
#451725=CARTESIAN_POINT('Ctrl Pts',(-4.49719513441354,26.,5.94520571051427));
#451726=CARTESIAN_POINT('Ctrl Pts',(-4.50019561112957,26.,5.95377453080449));
#451727=CARTESIAN_POINT('Ctrl Pts',(-4.50329523558538,26.,5.96230961479921));
#451728=CARTESIAN_POINT('Ctrl Pts',(-4.50648983134602,26.,5.97079740732105));
#451729=CARTESIAN_POINT('Ctrl Pts',(-4.52352595480839,26.,6.01606106261884));
#451730=CARTESIAN_POINT('Ctrl Pts',(-4.54329052844941,26.,6.06007213708267));
#451731=CARTESIAN_POINT('Ctrl Pts',(-4.56579698909062,26.,6.10256102518446));
#451732=CARTESIAN_POINT('Ctrl Pts',(-4.58190696962665,26.,6.13297429945397));
#451733=CARTESIAN_POINT('Ctrl Pts',(-4.59942271299284,26.,6.16260727981646));
#451734=CARTESIAN_POINT('Ctrl Pts',(-4.61836202894701,26.,6.1913507700685));
#451735=CARTESIAN_POINT('Ctrl Pts',(-4.64360162105055,26.,6.22965595338923));
#451736=CARTESIAN_POINT('Ctrl Pts',(-4.67136946042345,26.,6.2663827545985));
#451737=CARTESIAN_POINT('Ctrl Pts',(-4.70144469586272,26.,6.30137698491027));
#451738=CARTESIAN_POINT('Ctrl Pts',(-4.70937507558004,26.,6.31060442836116));
#451739=CARTESIAN_POINT('Ctrl Pts',(-4.71746597339309,26.,6.31971121578808));
#451740=CARTESIAN_POINT('Ctrl Pts',(-4.72571349227076,26.,6.32869409556074));
#451741=CARTESIAN_POINT('Ctrl Pts',(-4.7319332089771,26.,6.33546837134255));
#451742=CARTESIAN_POINT('Ctrl Pts',(-4.73824213428106,26.,6.34217214624876));
#451743=CARTESIAN_POINT('Ctrl Pts',(-4.74462823867121,26.,6.34879370705498));
#451744=CARTESIAN_POINT('Ctrl Pts',(-4.77811675592868,26.,6.383516949862));
#451745=CARTESIAN_POINT('Ctrl Pts',(-4.81379250850578,26.,6.41605753626979));
#451746=CARTESIAN_POINT('Ctrl Pts',(-4.85136909771721,26.,6.44627580177665));
#451747=CARTESIAN_POINT('Ctrl Pts',(-4.88884303449548,26.,6.47641151645744));
#451748=CARTESIAN_POINT('Ctrl Pts',(-4.92820865018765,26.,6.5042380382894));
#451749=CARTESIAN_POINT('Ctrl Pts',(-4.96920312730568,26.,6.52957020069408));
#451750=CARTESIAN_POINT('Ctrl Pts',(-4.99115415972337,26.,6.54313464052225));
#451751=CARTESIAN_POINT('Ctrl Pts',(-5.01357247298336,26.,6.55598305841263));
#451752=CARTESIAN_POINT('Ctrl Pts',(-5.03641841922373,26.,6.5680808187763));
#451753=CARTESIAN_POINT('Ctrl Pts',(-5.04828493017013,26.,6.57436456838649));
#451754=CARTESIAN_POINT('Ctrl Pts',(-5.06026681276785,26.,6.58044572292179));
#451755=CARTESIAN_POINT('Ctrl Pts',(-5.07235847244907,26.,6.5863189316705));
#451756=CARTESIAN_POINT('Ctrl Pts',(-5.08162063377995,26.,6.59081778529314));
#451757=CARTESIAN_POINT('Ctrl Pts',(-5.09094758400247,26.,6.595194652643));
#451758=CARTESIAN_POINT('Ctrl Pts',(-5.1003228721107,26.,6.59944110229105));
#451759=CARTESIAN_POINT('Ctrl Pts',(-5.14250847571933,26.,6.61854867952265));
#451760=CARTESIAN_POINT('Ctrl Pts',(-5.18574009204136,26.,6.63505331110801));
#451761=CARTESIAN_POINT('Ctrl Pts',(-5.22977562435799,26.,6.64877678422178));
#451762=CARTESIAN_POINT('Ctrl Pts',(-5.2594804397383,26.,6.65803415466278));
#451763=CARTESIAN_POINT('Ctrl Pts',(-5.28955126504646,26.,6.66602500922537));
#451764=CARTESIAN_POINT('Ctrl Pts',(-5.31991283796277,26.,6.67268119205492));
#451765=CARTESIAN_POINT('Ctrl Pts',(-5.33301953811817,26.,6.67555458049125));
#451766=CARTESIAN_POINT('Ctrl Pts',(-5.34618251319858,26.,6.67817927295424));
#451767=CARTESIAN_POINT('Ctrl Pts',(-5.35937322816289,26.,6.68054575323129));
#451768=CARTESIAN_POINT('Ctrl Pts',(-5.40277073101277,26.,6.68833148242381));
#451769=CARTESIAN_POINT('Ctrl Pts',(-5.44652175703517,26.,6.69333871127755));
#451770=CARTESIAN_POINT('Ctrl Pts',(-5.4904069101605,26.,6.6953834466363));
#451771=CARTESIAN_POINT('Ctrl Pts',(-5.51211121371639,26.,6.69639471249176));
#451772=CARTESIAN_POINT('Ctrl Pts',(-5.53384821037469,26.,6.69668059243942));
#451773=CARTESIAN_POINT('Ctrl Pts',(-5.55559016156262,26.,6.69621420261903));
#451774=CARTESIAN_POINT('Ctrl Pts',(-5.56854309351446,26.,6.69593634735414));
#451775=CARTESIAN_POINT('Ctrl Pts',(-5.58149776570054,26.,6.69539142062068));
#451776=CARTESIAN_POINT('Ctrl Pts',(-5.59444726164187,26.,6.69458228414866));
#451777=CARTESIAN_POINT('Ctrl Pts',(-6.69274404704181,26.,5.59475217632212));
#451778=CARTESIAN_POINT('Ctrl Pts',(-6.69531021368757,26.,5.55137724984311));
#451779=CARTESIAN_POINT('Ctrl Pts',(-6.69492058849835,26.,5.50802061877154));
#451780=CARTESIAN_POINT('Ctrl Pts',(-6.69178524360462,26.,5.4649019749424));
#451781=CARTESIAN_POINT('Ctrl Pts',(-6.6885064316043,26.,5.41981030827847));
#451782=CARTESIAN_POINT('Ctrl Pts',(-6.6822250250606,26.,5.3749781156863));
#451783=CARTESIAN_POINT('Ctrl Pts',(-6.67312701402814,26.,5.33063916085636));
#451784=CARTESIAN_POINT('Ctrl Pts',(-6.66611881409995,26.,5.29648485405826));
#451785=CARTESIAN_POINT('Ctrl Pts',(-6.657438192268,26.,5.26262271564401));
#451786=CARTESIAN_POINT('Ctrl Pts',(-6.64714921184179,26.,5.22915790417526));
#451787=CARTESIAN_POINT('Ctrl Pts',(-6.64373212639213,26.,5.2180438660871));
#451788=CARTESIAN_POINT('Ctrl Pts',(-6.64013749916696,26.,5.20697366141539));
#451789=CARTESIAN_POINT('Ctrl Pts',(-6.63636725687979,26.,5.19595119703594));
#451790=CARTESIAN_POINT('Ctrl Pts',(-6.63377142469848,26.,5.18836217076809));
#451791=CARTESIAN_POINT('Ctrl Pts',(-6.63109312202817,26.,5.18079825567733));
#451792=CARTESIAN_POINT('Ctrl Pts',(-6.62833627003802,26.,5.17326885643069));
#451793=CARTESIAN_POINT('Ctrl Pts',(-6.61217427924751,26.,5.1291279008345));
#451794=CARTESIAN_POINT('Ctrl Pts',(-6.59328941999762,26.,5.08609247696685));
#451795=CARTESIAN_POINT('Ctrl Pts',(-6.57188267750787,26.,5.04440658587507));
#451796=CARTESIAN_POINT('Ctrl Pts',(-6.55005077161978,26.,5.00189276334404));
#451797=CARTESIAN_POINT('Ctrl Pts',(-6.52559561372727,26.,4.96078147197193));
#451798=CARTESIAN_POINT('Ctrl Pts',(-6.49867698438676,26.,4.92133403622236));
#451799=CARTESIAN_POINT('Ctrl Pts',(-6.48030858559407,26.,4.89441638666335));
#451800=CARTESIAN_POINT('Ctrl Pts',(-6.46079201260925,26.,4.86827351967756));
#451801=CARTESIAN_POINT('Ctrl Pts',(-6.4401650142142,26.,4.84299340446309));
#451802=CARTESIAN_POINT('Ctrl Pts',(-6.43429026385467,26.,4.83579340555386));
#451803=CARTESIAN_POINT('Ctrl Pts',(-6.42832537837765,26.,4.82866342617017));
#451804=CARTESIAN_POINT('Ctrl Pts',(-6.42227108527737,26.,4.82160559536045));
#451805=CARTESIAN_POINT('Ctrl Pts',(-6.41650772986347,26.,4.81488692701488));
#451806=CARTESIAN_POINT('Ctrl Pts',(-6.41066935775182,26.,4.80824066086902));
#451807=CARTESIAN_POINT('Ctrl Pts',(-6.40475816436008,26.,4.80166944006503));
#451808=CARTESIAN_POINT('Ctrl Pts',(-6.37181647988102,26.,4.76504957872374));
#451809=CARTESIAN_POINT('Ctrl Pts',(-6.3366074009898,26.,4.73074760271325));
#451810=CARTESIAN_POINT('Ctrl Pts',(-6.29931177973046,26.,4.69903040790721));
#451811=CARTESIAN_POINT('Ctrl Pts',(-6.27627712598951,26.,4.67944112167677));
#451812=CARTESIAN_POINT('Ctrl Pts',(-6.25244551905118,26.,4.66083800978401));
#451813=CARTESIAN_POINT('Ctrl Pts',(-6.22785054805505,26.,4.64328815682614));
#451814=CARTESIAN_POINT('Ctrl Pts',(-6.18906673591271,26.,4.61561379199964));
#451815=CARTESIAN_POINT('Ctrl Pts',(-6.14838638392197,26.,4.59055615782454));
#451816=CARTESIAN_POINT('Ctrl Pts',(-6.10609561292347,26.,4.56810357334095));
#451817=CARTESIAN_POINT('Ctrl Pts',(-6.0966350271612,26.,4.56308085571068));
#451818=CARTESIAN_POINT('Ctrl Pts',(-6.08709371894873,26.,4.55818866062255));
#451819=CARTESIAN_POINT('Ctrl Pts',(-6.0774746818157,26.,4.55342713549933));
#451820=CARTESIAN_POINT('Ctrl Pts',(-6.06937447312086,26.,4.54941744651794));
#451821=CARTESIAN_POINT('Ctrl Pts',(-6.06122106951547,26.,4.54550147490651));
#451822=CARTESIAN_POINT('Ctrl Pts',(-6.05302670560527,26.,4.54168378413803));
#451823=CARTESIAN_POINT('Ctrl Pts',(-6.00844180822155,26.,4.52091202527781));
#451824=CARTESIAN_POINT('Ctrl Pts',(-5.9625645247388,26.,4.5030051530968));
#451825=CARTESIAN_POINT('Ctrl Pts',(-5.91572767775388,26.,4.48791424199878));
#451826=CARTESIAN_POINT('Ctrl Pts',(-5.86771907710826,26.,4.4724457898949));
#451827=CARTESIAN_POINT('Ctrl Pts',(-5.81870139486952,26.,4.45993552318701));
#451828=CARTESIAN_POINT('Ctrl Pts',(-5.76899658983648,26.,4.45037293016505));
#451829=CARTESIAN_POINT('Ctrl Pts',(-5.73932381395939,26.,4.44466425311952));
#451830=CARTESIAN_POINT('Ctrl Pts',(-5.70940552486093,26.,4.4400069173499));
#451831=CARTESIAN_POINT('Ctrl Pts',(-5.67930640361674,26.,4.43640656180746));
#451832=CARTESIAN_POINT('Ctrl Pts',(-5.66273112491008,26.,4.4344238827759));
#451833=CARTESIAN_POINT('Ctrl Pts',(-5.6461009688343,26.,4.4327618494722));
#451834=CARTESIAN_POINT('Ctrl Pts',(-5.62942654610506,26.,4.4314222120057));
#451835=CARTESIAN_POINT('Ctrl Pts',(-5.62032969654203,26.,4.4306913632861));
#451836=CARTESIAN_POINT('Ctrl Pts',(-5.61122148290957,26.,4.43005669150461));
#451837=CARTESIAN_POINT('Ctrl Pts',(-5.60211289272811,26.,4.42951879017363));
#451838=CARTESIAN_POINT('Ctrl Pts',(-5.54956970763969,26.,4.4264158896556));
#451839=CARTESIAN_POINT('Ctrl Pts',(-5.4969304712558,26.,4.42652201105729));
#451840=CARTESIAN_POINT('Ctrl Pts',(-5.44453981443333,26.,4.42983270797829));
#451841=CARTESIAN_POINT('Ctrl Pts',(-5.40884734549178,26.,4.43208820455334));
#451842=CARTESIAN_POINT('Ctrl Pts',(-5.37326963814493,26.,4.43583203037196));
#451843=CARTESIAN_POINT('Ctrl Pts',(-5.33791219834493,26.,4.44107619046014));
#451844=CARTESIAN_POINT('Ctrl Pts',(-5.32154784147763,26.,4.44350332623801));
#451845=CARTESIAN_POINT('Ctrl Pts',(-5.3052257211536,26.,4.44625314527356));
#451846=CARTESIAN_POINT('Ctrl Pts',(-5.2889864307097,26.,4.44932134384721));
#451847=CARTESIAN_POINT('Ctrl Pts',(-5.23677996517828,26.,4.45918506317858));
#451848=CARTESIAN_POINT('Ctrl Pts',(-5.18537728352641,26.,4.47234120944802));
#451849=CARTESIAN_POINT('Ctrl Pts',(-5.13511946191399,26.,4.48880818879318));
#451850=CARTESIAN_POINT('Ctrl Pts',(-5.10845853162224,26.,4.49754364477499));
#451851=CARTESIAN_POINT('Ctrl Pts',(-5.08211963725754,26.,4.50721166236008));
#451852=CARTESIAN_POINT('Ctrl Pts',(-5.05615381819268,26.,4.51782098438608));
#451853=CARTESIAN_POINT('Ctrl Pts',(-5.04134050525441,26.,4.52387352626206));
#451854=CARTESIAN_POINT('Ctrl Pts',(-5.02664862375098,26.,4.53023250440261));
#451855=CARTESIAN_POINT('Ctrl Pts',(-5.01208247494515,26.,4.53689020456271));
#451856=CARTESIAN_POINT('Ctrl Pts',(-5.01302286563431,26.,-4.53900700771688));
#451857=CARTESIAN_POINT('Ctrl Pts',(-5.06076150603835,26.,-4.51730428611638));
#451858=CARTESIAN_POINT('Ctrl Pts',(-5.10974961966388,26.,-4.49883681289365));
#451859=CARTESIAN_POINT('Ctrl Pts',(-5.1596701907311,26.,-4.48353831525793));
#451860=CARTESIAN_POINT('Ctrl Pts',(-5.21017178076207,26.,-4.46806176041948));
#451861=CARTESIAN_POINT('Ctrl Pts',(-5.26162887990392,26.,-4.45582849042805));
#451862=CARTESIAN_POINT('Ctrl Pts',(-5.31372001428598,26.,-4.44682362697344));
#451863=CARTESIAN_POINT('Ctrl Pts',(-5.35139435755779,26.,-4.44031095795732));
#451864=CARTESIAN_POINT('Ctrl Pts',(-5.38940054503579,26.,-4.43548811807635));
#451865=CARTESIAN_POINT('Ctrl Pts',(-5.42761365593355,26.,-4.43236615256969));
#451866=CARTESIAN_POINT('Ctrl Pts',(-5.44398133170877,26.,-4.43102893301352));
#451867=CARTESIAN_POINT('Ctrl Pts',(-5.46038690932955,26.,-4.43000393185811));
#451868=CARTESIAN_POINT('Ctrl Pts',(-5.47682022646686,26.,-4.42929277127871));
#451869=CARTESIAN_POINT('Ctrl Pts',(-5.48697840405261,26.,-4.4288531707162));
#451870=CARTESIAN_POINT('Ctrl Pts',(-5.49714835623362,26.,-4.42853358462845));
#451871=CARTESIAN_POINT('Ctrl Pts',(-5.50731025740424,26.,-4.42833449333953));
#451872=CARTESIAN_POINT('Ctrl Pts',(-5.5588488060778,26.,-4.42732475353669));
#451873=CARTESIAN_POINT('Ctrl Pts',(-5.61028393904341,26.,-4.42940473009627));
#451874=CARTESIAN_POINT('Ctrl Pts',(-5.66131493504129,26.,-4.43455229706759));
#451875=CARTESIAN_POINT('Ctrl Pts',(-5.71118189317826,26.,-4.43958244593392));
#451876=CARTESIAN_POINT('Ctrl Pts',(-5.76066393975029,26.,-4.44754223429228));
#451877=CARTESIAN_POINT('Ctrl Pts',(-5.80946415691505,26.,-4.45845673166055));
#451878=CARTESIAN_POINT('Ctrl Pts',(-5.84341695886652,26.,-4.4660505045795));
#451879=CARTESIAN_POINT('Ctrl Pts',(-5.87703937807783,26.,-4.47507550289942));
#451880=CARTESIAN_POINT('Ctrl Pts',(-5.91022284174077,26.,-4.48555225879131));
#451881=CARTESIAN_POINT('Ctrl Pts',(-5.92194029476516,26.,-4.48925171874697));
#451882=CARTESIAN_POINT('Ctrl Pts',(-5.93360293701868,26.,-4.49313228205386));
#451883=CARTESIAN_POINT('Ctrl Pts',(-5.94520571072346,26.,-4.49719513448679));
#451884=CARTESIAN_POINT('Ctrl Pts',(-5.95377453098711,26.,-4.50019561119532));
#451885=CARTESIAN_POINT('Ctrl Pts',(-5.9623096149553,26.,-4.50329523564298));
#451886=CARTESIAN_POINT('Ctrl Pts',(-5.9707974074509,26.,-4.50648983139489));
#451887=CARTESIAN_POINT('Ctrl Pts',(-6.01606106274569,26.,-4.52352595486226));
#451888=CARTESIAN_POINT('Ctrl Pts',(-6.06007213720631,26.,-4.5432905285082));
#451889=CARTESIAN_POINT('Ctrl Pts',(-6.10256102530468,26.,-4.5657969891543));
#451890=CARTESIAN_POINT('Ctrl Pts',(-6.13297429953205,26.,-4.5819069696728));
#451891=CARTESIAN_POINT('Ctrl Pts',(-6.16260727985433,26.,-4.59942271301779));
#451892=CARTESIAN_POINT('Ctrl Pts',(-6.1913507700685,26.,-4.61836202894701));
#451893=CARTESIAN_POINT('Ctrl Pts',(-6.22965595338923,26.,-4.64360162105055));
#451894=CARTESIAN_POINT('Ctrl Pts',(-6.26638275459849,26.,-4.67136946042345));
#451895=CARTESIAN_POINT('Ctrl Pts',(-6.30137698491027,26.,-4.70144469586272));
#451896=CARTESIAN_POINT('Ctrl Pts',(-6.31060442836122,26.,-4.7093750755801));
#451897=CARTESIAN_POINT('Ctrl Pts',(-6.31971121578822,26.,-4.71746597339321));
#451898=CARTESIAN_POINT('Ctrl Pts',(-6.32869409556094,26.,-4.72571349227094));
#451899=CARTESIAN_POINT('Ctrl Pts',(-6.33546837134828,26.,-4.73193320898236));
#451900=CARTESIAN_POINT('Ctrl Pts',(-6.34217214625989,26.,-4.73824213429154));
#451901=CARTESIAN_POINT('Ctrl Pts',(-6.34879370707138,26.,-4.74462823868703));
#451902=CARTESIAN_POINT('Ctrl Pts',(-6.38351694987776,26.,-4.77811675594523));
#451903=CARTESIAN_POINT('Ctrl Pts',(-6.41605753628488,26.,-4.81379250852302));
#451904=CARTESIAN_POINT('Ctrl Pts',(-6.44627580179103,26.,-4.85136909773509));
#451905=CARTESIAN_POINT('Ctrl Pts',(-6.47641151647102,26.,-4.88884303451388));
#451906=CARTESIAN_POINT('Ctrl Pts',(-6.50423803830216,26.,-4.92820865020652));
#451907=CARTESIAN_POINT('Ctrl Pts',(-6.529570200706,26.,-4.96920312732498));
#451908=CARTESIAN_POINT('Ctrl Pts',(-6.54313464053326,26.,-4.99115415974213));
#451909=CARTESIAN_POINT('Ctrl Pts',(-6.55598305842276,26.,-5.01357247300154));
#451910=CARTESIAN_POINT('Ctrl Pts',(-6.5680808187856,26.,-5.0364184192413));
#451911=CARTESIAN_POINT('Ctrl Pts',(-6.57436456839916,26.,-5.04828493019454));
#451912=CARTESIAN_POINT('Ctrl Pts',(-6.58044572293759,26.,-5.06026681279923));
#451913=CARTESIAN_POINT('Ctrl Pts',(-6.58631893168919,26.,-5.07235847248755));
#451914=CARTESIAN_POINT('Ctrl Pts',(-6.59081778529731,26.,-5.08162063378941));
#451915=CARTESIAN_POINT('Ctrl Pts',(-6.59519465263342,26.,-5.09094758398249));
#451916=CARTESIAN_POINT('Ctrl Pts',(-6.59944110226853,26.,-5.10032287206098));
#451917=CARTESIAN_POINT('Ctrl Pts',(-6.61854867950197,26.,-5.14250847566835));
#451918=CARTESIAN_POINT('Ctrl Pts',(-6.63505331108929,26.,-5.18574009198917));
#451919=CARTESIAN_POINT('Ctrl Pts',(-6.64877678420517,26.,-5.22977562430468));
#451920=CARTESIAN_POINT('Ctrl Pts',(-6.65803415464525,26.,-5.25948043967676));
#451921=CARTESIAN_POINT('Ctrl Pts',(-6.66602500920764,26.,-5.28955126497656));
#451922=CARTESIAN_POINT('Ctrl Pts',(-6.67268119203775,26.,-5.31991283788441));
#451923=CARTESIAN_POINT('Ctrl Pts',(-6.6755545804784,26.,-5.33301953805478));
#451924=CARTESIAN_POINT('Ctrl Pts',(-6.67817927294514,26.,-5.34618251315033));
#451925=CARTESIAN_POINT('Ctrl Pts',(-6.68054575322537,26.,-5.35937322812986));
#451926=CARTESIAN_POINT('Ctrl Pts',(-6.68833148241942,26.,-5.40277073098025));
#451927=CARTESIAN_POINT('Ctrl Pts',(-6.69333871127465,26.,-5.44652175700321));
#451928=CARTESIAN_POINT('Ctrl Pts',(-6.69538344663484,26.,-5.49040691012916));
#451929=CARTESIAN_POINT('Ctrl Pts',(-6.69639471249149,26.,-5.51211121369546));
#451930=CARTESIAN_POINT('Ctrl Pts',(-6.69668059243965,26.,-5.53384821036422));
#451931=CARTESIAN_POINT('Ctrl Pts',(-6.69621420261903,26.,-5.55559016156262));
#451932=CARTESIAN_POINT('Ctrl Pts',(-6.69593634735414,26.,-5.56854309351446));
#451933=CARTESIAN_POINT('Ctrl Pts',(-6.69539142062068,26.,-5.58149776570054));
#451934=CARTESIAN_POINT('Ctrl Pts',(-6.69458228414866,26.,-5.59444726164187));
#451935=CARTESIAN_POINT('Ctrl Pts',(-5.59475217632212,26.,-6.69274404704181));
#451936=CARTESIAN_POINT('Ctrl Pts',(-5.55137724984312,26.,-6.69531021368757));
#451937=CARTESIAN_POINT('Ctrl Pts',(-5.50802061877154,26.,-6.69492058849835));
#451938=CARTESIAN_POINT('Ctrl Pts',(-5.46490197494241,26.,-6.69178524360462));
#451939=CARTESIAN_POINT('Ctrl Pts',(-5.4198103082784,26.,-6.68850643160429));
#451940=CARTESIAN_POINT('Ctrl Pts',(-5.37497811568615,26.,-6.68222502506058));
#451941=CARTESIAN_POINT('Ctrl Pts',(-5.33063916085613,26.,-6.67312701402809));
#451942=CARTESIAN_POINT('Ctrl Pts',(-5.29648485405804,26.,-6.6661188140999));
#451943=CARTESIAN_POINT('Ctrl Pts',(-5.2626227156438,26.,-6.65743819226794));
#451944=CARTESIAN_POINT('Ctrl Pts',(-5.22915790417506,26.,-6.64714921184172));
#451945=CARTESIAN_POINT('Ctrl Pts',(-5.21804386616628,26.,-6.64373212641647));
#451946=CARTESIAN_POINT('Ctrl Pts',(-5.20697366157331,26.,-6.64013749921824));
#451947=CARTESIAN_POINT('Ctrl Pts',(-5.19595119727191,26.,-6.6363672569605));
#451948=CARTESIAN_POINT('Ctrl Pts',(-5.1883621710592,26.,-6.63377142479994));
#451949=CARTESIAN_POINT('Ctrl Pts',(-5.18079825602294,26.,-6.63109312215148));
#451950=CARTESIAN_POINT('Ctrl Pts',(-5.17326885683034,26.,-6.62833627018435));
#451951=CARTESIAN_POINT('Ctrl Pts',(-5.1291279012311,26.,-6.61217427941162));
#451952=CARTESIAN_POINT('Ctrl Pts',(-5.08609247735947,26.,-6.59328942017928));
#451953=CARTESIAN_POINT('Ctrl Pts',(-5.04440658626274,26.,-6.57188267770694));
#451954=CARTESIAN_POINT('Ctrl Pts',(-5.00189276372273,26.,-6.5500507718346));
#451955=CARTESIAN_POINT('Ctrl Pts',(-4.9607814723409,26.,-6.52559561395722));
#451956=CARTESIAN_POINT('Ctrl Pts',(-4.92133403658083,26.,-6.49867698463137));
#451957=CARTESIAN_POINT('Ctrl Pts',(-4.89441638698506,26.,-6.4803085858285));
#451958=CARTESIAN_POINT('Ctrl Pts',(-4.86827351996386,26.,-6.46079201283075));
#451959=CARTESIAN_POINT('Ctrl Pts',(-4.84299340471559,26.,-6.44016501442022));
#451960=CARTESIAN_POINT('Ctrl Pts',(-4.83579340611366,26.,-6.43429026431488));
#451961=CARTESIAN_POINT('Ctrl Pts',(-4.82866342703126,26.,-6.42832537909978));
#451962=CARTESIAN_POINT('Ctrl Pts',(-4.8216055965165,26.,-6.42227108626905));
#451963=CARTESIAN_POINT('Ctrl Pts',(-4.81488692784565,26.,-6.41650773059184));
#451964=CARTESIAN_POINT('Ctrl Pts',(-4.80824066137958,26.,-6.41066935820828));
#451965=CARTESIAN_POINT('Ctrl Pts',(-4.80166944026328,26.,-6.40475816453841));
#451966=CARTESIAN_POINT('Ctrl Pts',(-4.76504957891336,26.,-6.37181648006733));
#451967=CARTESIAN_POINT('Ctrl Pts',(-4.73074760289381,26.,-6.33660740118367));
#451968=CARTESIAN_POINT('Ctrl Pts',(-4.69903040807827,26.,-6.2993117799316));
#451969=CARTESIAN_POINT('Ctrl Pts',(-4.67944112178507,26.,-6.27627712612825));
#451970=CARTESIAN_POINT('Ctrl Pts',(-4.6608380098351,26.,-6.25244551912277));
#451971=CARTESIAN_POINT('Ctrl Pts',(-4.64328815682614,26.,-6.22785054805505));
#451972=CARTESIAN_POINT('Ctrl Pts',(-4.61561379199964,26.,-6.1890667359127));
#451973=CARTESIAN_POINT('Ctrl Pts',(-4.59055615782454,26.,-6.14838638392196));
#451974=CARTESIAN_POINT('Ctrl Pts',(-4.56810357334094,26.,-6.10609561292346));
#451975=CARTESIAN_POINT('Ctrl Pts',(-4.56308085570443,26.,-6.09663502714943));
#451976=CARTESIAN_POINT('Ctrl Pts',(-4.55818866061037,26.,-6.08709371892498));
#451977=CARTESIAN_POINT('Ctrl Pts',(-4.55342713548155,26.,-6.07747468177979));
#451978=CARTESIAN_POINT('Ctrl Pts',(-4.54941744650604,26.,-6.0693744730961));
#451979=CARTESIAN_POINT('Ctrl Pts',(-4.54550147490024,26.,-6.06122106950204));
#451980=CARTESIAN_POINT('Ctrl Pts',(-4.54168378413711,26.,-6.05302670560328));
#451981=CARTESIAN_POINT('Ctrl Pts',(-4.52091202527692,26.,-6.00844180821941));
#451982=CARTESIAN_POINT('Ctrl Pts',(-4.50300515309595,26.,-5.96256452473651));
#451983=CARTESIAN_POINT('Ctrl Pts',(-4.487914241998,26.,-5.91572767775144));
#451984=CARTESIAN_POINT('Ctrl Pts',(-4.47244578989431,26.,-5.86771907710606));
#451985=CARTESIAN_POINT('Ctrl Pts',(-4.45993552318657,26.,-5.81870139486759));
#451986=CARTESIAN_POINT('Ctrl Pts',(-4.45037293016473,26.,-5.76899658983482));
#451987=CARTESIAN_POINT('Ctrl Pts',(-4.44466425311925,26.,-5.73932381395779));
#451988=CARTESIAN_POINT('Ctrl Pts',(-4.44000691734968,26.,-5.70940552485939));
#451989=CARTESIAN_POINT('Ctrl Pts',(-4.43640656180728,26.,-5.67930640361527));
#451990=CARTESIAN_POINT('Ctrl Pts',(-4.43442388277574,26.,-5.66273112490856));
#451991=CARTESIAN_POINT('Ctrl Pts',(-4.43276184947206,26.,-5.64610096883273));
#451992=CARTESIAN_POINT('Ctrl Pts',(-4.43142221200557,26.,-5.62942654610346));
#451993=CARTESIAN_POINT('Ctrl Pts',(-4.43069136328561,26.,-5.62032969653584));
#451994=CARTESIAN_POINT('Ctrl Pts',(-4.43005669150386,26.,-5.61122148289879));
#451995=CARTESIAN_POINT('Ctrl Pts',(-4.42951879017273,26.,-5.60211289271274));
#451996=CARTESIAN_POINT('Ctrl Pts',(-4.42641588965533,26.,-5.54956970762436));
#451997=CARTESIAN_POINT('Ctrl Pts',(-4.42652201105763,26.,-5.49693047124056));
#451998=CARTESIAN_POINT('Ctrl Pts',(-4.42983270797924,26.,-5.44453981441821));
#451999=CARTESIAN_POINT('Ctrl Pts',(-4.43208820455486,26.,-5.40884734547433));
#452000=CARTESIAN_POINT('Ctrl Pts',(-4.43583203037426,26.,-5.3732696381252));
#452001=CARTESIAN_POINT('Ctrl Pts',(-4.4410761904634,26.,-5.33791219832296));
#452002=CARTESIAN_POINT('Ctrl Pts',(-4.44350332624102,26.,-5.32154784145933));
#452003=CARTESIAN_POINT('Ctrl Pts',(-4.44625314527617,26.,-5.30522572113897));
#452004=CARTESIAN_POINT('Ctrl Pts',(-4.44932134384929,26.,-5.28898643069871));
#452005=CARTESIAN_POINT('Ctrl Pts',(-4.45918506318114,26.,-5.23677996516729));
#452006=CARTESIAN_POINT('Ctrl Pts',(-4.47234120945108,26.,-5.18537728351545));
#452007=CARTESIAN_POINT('Ctrl Pts',(-4.48880818879675,26.,-5.1351194619031));
#452008=CARTESIAN_POINT('Ctrl Pts',(-4.49754364477762,26.,-5.10845853161507));
#452009=CARTESIAN_POINT('Ctrl Pts',(-4.50721166236153,26.,-5.08211963725401));
#452010=CARTESIAN_POINT('Ctrl Pts',(-4.51782098438609,26.,-5.05615381819268));
#452011=CARTESIAN_POINT('Ctrl Pts',(-4.52387352626206,26.,-5.0413405052544));
#452012=CARTESIAN_POINT('Ctrl Pts',(-4.53023250440261,26.,-5.02664862375098));
#452013=CARTESIAN_POINT('Ctrl Pts',(-4.53689020456271,26.,-5.01208247494515));
#452014=CARTESIAN_POINT('Ctrl Pts',(4.53900700771688,26.,-5.01302286563431));
#452015=CARTESIAN_POINT('Ctrl Pts',(4.51730428611638,26.,-5.06076150603835));
#452016=CARTESIAN_POINT('Ctrl Pts',(4.49883681289365,26.,-5.10974961966388));
#452017=CARTESIAN_POINT('Ctrl Pts',(4.48353831525793,26.,-5.1596701907311));
#452018=CARTESIAN_POINT('Ctrl Pts',(4.46806176041948,26.,-5.21017178076207));
#452019=CARTESIAN_POINT('Ctrl Pts',(4.45582849042805,26.,-5.26162887990392));
#452020=CARTESIAN_POINT('Ctrl Pts',(4.44682362697344,26.,-5.31372001428598));
#452021=CARTESIAN_POINT('Ctrl Pts',(4.44031095795732,26.,-5.35139435755779));
#452022=CARTESIAN_POINT('Ctrl Pts',(4.43548811807635,26.,-5.38940054503579));
#452023=CARTESIAN_POINT('Ctrl Pts',(4.43236615256969,26.,-5.42761365593355));
#452024=CARTESIAN_POINT('Ctrl Pts',(4.43102893301352,26.,-5.44398133170877));
#452025=CARTESIAN_POINT('Ctrl Pts',(4.43000393185811,26.,-5.46038690932955));
#452026=CARTESIAN_POINT('Ctrl Pts',(4.42929277127871,26.,-5.47682022646686));
#452027=CARTESIAN_POINT('Ctrl Pts',(4.4288531707162,26.,-5.48697840405261));
#452028=CARTESIAN_POINT('Ctrl Pts',(4.42853358462845,26.,-5.49714835623362));
#452029=CARTESIAN_POINT('Ctrl Pts',(4.42833449333953,26.,-5.50731025740424));
#452030=CARTESIAN_POINT('Ctrl Pts',(4.42732475353669,26.,-5.5588488060778));
#452031=CARTESIAN_POINT('Ctrl Pts',(4.42940473009627,26.,-5.61028393904341));
#452032=CARTESIAN_POINT('Ctrl Pts',(4.43455229706759,26.,-5.66131493504129));
#452033=CARTESIAN_POINT('Ctrl Pts',(4.43958244593392,26.,-5.71118189317826));
#452034=CARTESIAN_POINT('Ctrl Pts',(4.44754223429228,26.,-5.76066393975029));
#452035=CARTESIAN_POINT('Ctrl Pts',(4.45845673166055,26.,-5.80946415691505));
#452036=CARTESIAN_POINT('Ctrl Pts',(4.4660505045795,26.,-5.84341695886652));
#452037=CARTESIAN_POINT('Ctrl Pts',(4.47507550289942,26.,-5.87703937807783));
#452038=CARTESIAN_POINT('Ctrl Pts',(4.48555225879131,26.,-5.91022284174077));
#452039=CARTESIAN_POINT('Ctrl Pts',(4.48925171874697,26.,-5.92194029476516));
#452040=CARTESIAN_POINT('Ctrl Pts',(4.49313228205386,26.,-5.93360293701868));
#452041=CARTESIAN_POINT('Ctrl Pts',(4.49719513448679,26.,-5.94520571072346));
#452042=CARTESIAN_POINT('Ctrl Pts',(4.50019561119532,26.,-5.95377453098711));
#452043=CARTESIAN_POINT('Ctrl Pts',(4.50329523564298,26.,-5.9623096149553));
#452044=CARTESIAN_POINT('Ctrl Pts',(4.50648983139489,26.,-5.9707974074509));
#452045=CARTESIAN_POINT('Ctrl Pts',(4.52352595486226,26.,-6.01606106274569));
#452046=CARTESIAN_POINT('Ctrl Pts',(4.5432905285082,26.,-6.06007213720631));
#452047=CARTESIAN_POINT('Ctrl Pts',(4.5657969891543,26.,-6.10256102530468));
#452048=CARTESIAN_POINT('Ctrl Pts',(4.5819069696728,26.,-6.13297429953205));
#452049=CARTESIAN_POINT('Ctrl Pts',(4.59942271301779,26.,-6.16260727985433));
#452050=CARTESIAN_POINT('Ctrl Pts',(4.61836202894701,26.,-6.1913507700685));
#452051=CARTESIAN_POINT('Ctrl Pts',(4.64360162105055,26.,-6.22965595338923));
#452052=CARTESIAN_POINT('Ctrl Pts',(4.67136946042345,26.,-6.26638275459849));
#452053=CARTESIAN_POINT('Ctrl Pts',(4.70144469586272,26.,-6.30137698491027));
#452054=CARTESIAN_POINT('Ctrl Pts',(4.7093750755801,26.,-6.31060442836122));
#452055=CARTESIAN_POINT('Ctrl Pts',(4.71746597339321,26.,-6.31971121578822));
#452056=CARTESIAN_POINT('Ctrl Pts',(4.72571349227094,26.,-6.32869409556094));
#452057=CARTESIAN_POINT('Ctrl Pts',(4.73193320898236,26.,-6.33546837134828));
#452058=CARTESIAN_POINT('Ctrl Pts',(4.73824213429154,26.,-6.34217214625989));
#452059=CARTESIAN_POINT('Ctrl Pts',(4.74462823868703,26.,-6.34879370707138));
#452060=CARTESIAN_POINT('Ctrl Pts',(4.77811675594523,26.,-6.38351694987776));
#452061=CARTESIAN_POINT('Ctrl Pts',(4.81379250852302,26.,-6.41605753628488));
#452062=CARTESIAN_POINT('Ctrl Pts',(4.85136909773509,26.,-6.44627580179103));
#452063=CARTESIAN_POINT('Ctrl Pts',(4.88884303451388,26.,-6.47641151647102));
#452064=CARTESIAN_POINT('Ctrl Pts',(4.92820865020652,26.,-6.50423803830216));
#452065=CARTESIAN_POINT('Ctrl Pts',(4.96920312732498,26.,-6.529570200706));
#452066=CARTESIAN_POINT('Ctrl Pts',(4.99115415974213,26.,-6.54313464053326));
#452067=CARTESIAN_POINT('Ctrl Pts',(5.01357247300154,26.,-6.55598305842276));
#452068=CARTESIAN_POINT('Ctrl Pts',(5.0364184192413,26.,-6.5680808187856));
#452069=CARTESIAN_POINT('Ctrl Pts',(5.04828493019454,26.,-6.57436456839916));
#452070=CARTESIAN_POINT('Ctrl Pts',(5.06026681279923,26.,-6.58044572293759));
#452071=CARTESIAN_POINT('Ctrl Pts',(5.07235847248755,26.,-6.58631893168919));
#452072=CARTESIAN_POINT('Ctrl Pts',(5.08162063378941,26.,-6.59081778529731));
#452073=CARTESIAN_POINT('Ctrl Pts',(5.09094758398249,26.,-6.59519465263342));
#452074=CARTESIAN_POINT('Ctrl Pts',(5.10032287206098,26.,-6.59944110226853));
#452075=CARTESIAN_POINT('Ctrl Pts',(5.14250847566835,26.,-6.61854867950197));
#452076=CARTESIAN_POINT('Ctrl Pts',(5.18574009198917,26.,-6.63505331108929));
#452077=CARTESIAN_POINT('Ctrl Pts',(5.22977562430468,26.,-6.64877678420517));
#452078=CARTESIAN_POINT('Ctrl Pts',(5.25948043967676,26.,-6.65803415464525));
#452079=CARTESIAN_POINT('Ctrl Pts',(5.28955126497656,26.,-6.66602500920764));
#452080=CARTESIAN_POINT('Ctrl Pts',(5.31991283788441,26.,-6.67268119203775));
#452081=CARTESIAN_POINT('Ctrl Pts',(5.33301953805478,26.,-6.6755545804784));
#452082=CARTESIAN_POINT('Ctrl Pts',(5.34618251315033,26.,-6.67817927294514));
#452083=CARTESIAN_POINT('Ctrl Pts',(5.35937322812986,26.,-6.68054575322537));
#452084=CARTESIAN_POINT('Ctrl Pts',(5.40277073098025,26.,-6.68833148241942));
#452085=CARTESIAN_POINT('Ctrl Pts',(5.44652175700321,26.,-6.69333871127465));
#452086=CARTESIAN_POINT('Ctrl Pts',(5.49040691012916,26.,-6.69538344663484));
#452087=CARTESIAN_POINT('Ctrl Pts',(5.51211121369546,26.,-6.69639471249149));
#452088=CARTESIAN_POINT('Ctrl Pts',(5.53384821036422,26.,-6.69668059243965));
#452089=CARTESIAN_POINT('Ctrl Pts',(5.55559016156262,26.,-6.69621420261903));
#452090=CARTESIAN_POINT('Ctrl Pts',(5.56854309351446,26.,-6.69593634735414));
#452091=CARTESIAN_POINT('Ctrl Pts',(5.58149776570054,26.,-6.69539142062068));
#452092=CARTESIAN_POINT('Ctrl Pts',(5.59444726164187,26.,-6.69458228414866));
#452093=CARTESIAN_POINT('Ctrl Pts',(6.69274404704181,26.,-5.59475217632212));
#452094=CARTESIAN_POINT('Ctrl Pts',(6.69531021368757,26.,-5.55137724984312));
#452095=CARTESIAN_POINT('Ctrl Pts',(6.69492058849835,26.,-5.50802061877154));
#452096=CARTESIAN_POINT('Ctrl Pts',(6.69178524360462,26.,-5.46490197494242));
#452097=CARTESIAN_POINT('Ctrl Pts',(6.6885064316043,26.,-5.41981030827848));
#452098=CARTESIAN_POINT('Ctrl Pts',(6.6822250250606,26.,-5.37497811568631));
#452099=CARTESIAN_POINT('Ctrl Pts',(6.67312701402814,26.,-5.33063916085636));
#452100=CARTESIAN_POINT('Ctrl Pts',(6.66611881409995,26.,-5.29648485405827));
#452101=CARTESIAN_POINT('Ctrl Pts',(6.657438192268,26.,-5.26262271564402));
#452102=CARTESIAN_POINT('Ctrl Pts',(6.64714921184178,26.,-5.22915790417526));
#452103=CARTESIAN_POINT('Ctrl Pts',(6.64373212641031,26.,-5.21804386614623));
#452104=CARTESIAN_POINT('Ctrl Pts',(6.6401374992052,26.,-5.20697366153317));
#452105=CARTESIAN_POINT('Ctrl Pts',(6.63636725693996,26.,-5.19595119721186));
#452106=CARTESIAN_POINT('Ctrl Pts',(6.63377142477236,26.,-5.18836217097996));
#452107=CARTESIAN_POINT('Ctrl Pts',(6.63109312211646,26.,-5.18079825592472));
#452108=CARTESIAN_POINT('Ctrl Pts',(6.62833627014149,26.,-5.17326885671329));
#452109=CARTESIAN_POINT('Ctrl Pts',(6.61217427936374,26.,-5.12912790111545));
#452110=CARTESIAN_POINT('Ctrl Pts',(6.59328942012651,26.,-5.08609247724548));
#452111=CARTESIAN_POINT('Ctrl Pts',(6.57188267764938,26.,-5.04440658615065));
#452112=CARTESIAN_POINT('Ctrl Pts',(6.55005077177248,26.,-5.00189276361322));
#452113=CARTESIAN_POINT('Ctrl Pts',(6.52559561389071,26.,-4.96078147223418));
#452114=CARTESIAN_POINT('Ctrl Pts',(6.49867698456061,26.,-4.92133403647713));
#452115=CARTESIAN_POINT('Ctrl Pts',(6.48030858576068,26.,-4.89441638689199));
#452116=CARTESIAN_POINT('Ctrl Pts',(6.46079201276668,26.,-4.86827351988104));
#452117=CARTESIAN_POINT('Ctrl Pts',(6.44016501436062,26.,-4.84299340464255));
#452118=CARTESIAN_POINT('Ctrl Pts',(6.43429026416939,26.,-4.83579340593657));
#452119=CARTESIAN_POINT('Ctrl Pts',(6.42832537886577,26.,-4.82866342675214));
#452120=CARTESIAN_POINT('Ctrl Pts',(6.42227108594394,26.,-4.82160559613751));
#452121=CARTESIAN_POINT('Ctrl Pts',(6.41650773035309,26.,-4.81488692757334));
#452122=CARTESIAN_POINT('Ctrl Pts',(6.41066935805872,26.,-4.80824066121229));
#452123=CARTESIAN_POINT('Ctrl Pts',(6.40475816448007,26.,-4.80166944019842));
#452124=CARTESIAN_POINT('Ctrl Pts',(6.37181648000639,26.,-4.76504957885134));
#452125=CARTESIAN_POINT('Ctrl Pts',(6.33660740112027,26.,-4.73074760283477));
#452126=CARTESIAN_POINT('Ctrl Pts',(6.29931177986584,26.,-4.69903040802235));
#452127=CARTESIAN_POINT('Ctrl Pts',(6.27627712608289,26.,-4.67944112174966));
#452128=CARTESIAN_POINT('Ctrl Pts',(6.25244551909937,26.,-4.6608380098184));
#452129=CARTESIAN_POINT('Ctrl Pts',(6.22785054805505,26.,-4.64328815682614));
#452130=CARTESIAN_POINT('Ctrl Pts',(6.18906673591271,26.,-4.61561379199964));
#452131=CARTESIAN_POINT('Ctrl Pts',(6.14838638392197,26.,-4.59055615782454));
#452132=CARTESIAN_POINT('Ctrl Pts',(6.10609561292348,26.,-4.56810357334095));
#452133=CARTESIAN_POINT('Ctrl Pts',(6.0966350271458,26.,-4.5630808557025));
#452134=CARTESIAN_POINT('Ctrl Pts',(6.08709371891765,26.,-4.55818866060661));
#452135=CARTESIAN_POINT('Ctrl Pts',(6.0774746817687,26.,-4.55342713547606));
#452136=CARTESIAN_POINT('Ctrl Pts',(6.06937447308074,26.,-4.54941744649855));
#452137=CARTESIAN_POINT('Ctrl Pts',(6.06122106948236,26.,-4.54550147489084));
#452138=CARTESIAN_POINT('Ctrl Pts',(6.05302670557925,26.,-4.54168378412591));
#452139=CARTESIAN_POINT('Ctrl Pts',(6.00844180819483,26.,-4.52091202526671));
#452140=CARTESIAN_POINT('Ctrl Pts',(5.96256452471144,26.,-4.50300515308674));
#452141=CARTESIAN_POINT('Ctrl Pts',(5.91572767772593,26.,-4.48791424198978));
#452142=CARTESIAN_POINT('Ctrl Pts',(5.86771907707987,26.,-4.47244578988703));
#452143=CARTESIAN_POINT('Ctrl Pts',(5.81870139484075,26.,-4.45993552318027));
#452144=CARTESIAN_POINT('Ctrl Pts',(5.76899658980738,26.,-4.45037293015945));
#452145=CARTESIAN_POINT('Ctrl Pts',(5.73932381393135,26.,-4.44466425311484));
#452146=CARTESIAN_POINT('Ctrl Pts',(5.70940552483398,26.,-4.44000691734606));
#452147=CARTESIAN_POINT('Ctrl Pts',(5.67930640359092,26.,-4.43640656180437));
#452148=CARTESIAN_POINT('Ctrl Pts',(5.66273112487801,26.,-4.43442388277241));
#452149=CARTESIAN_POINT('Ctrl Pts',(5.64610096879595,26.,-4.43276184946854));
#452150=CARTESIAN_POINT('Ctrl Pts',(5.62942654606042,26.,-4.43142221200212));
#452151=CARTESIAN_POINT('Ctrl Pts',(5.62032969647973,26.,-4.43069136328141));
#452152=CARTESIAN_POINT('Ctrl Pts',(5.61122148282963,26.,-4.4300566914992));
#452153=CARTESIAN_POINT('Ctrl Pts',(5.60211289263051,26.,-4.42951879016787));
#452154=CARTESIAN_POINT('Ctrl Pts',(5.54956970754168,26.,-4.4264158896538));
#452155=CARTESIAN_POINT('Ctrl Pts',(5.49693047115761,26.,-4.42652201105946));
#452156=CARTESIAN_POINT('Ctrl Pts',(5.44453981433516,26.,-4.42983270798449));
#452157=CARTESIAN_POINT('Ctrl Pts',(5.40884734538101,26.,-4.43208820456308));
#452158=CARTESIAN_POINT('Ctrl Pts',(5.37326963802174,26.,-4.43583203038632));
#452159=CARTESIAN_POINT('Ctrl Pts',(5.3379121982096,26.,-4.44107619048022));
#452160=CARTESIAN_POINT('Ctrl Pts',(5.32154784137259,26.,-4.4435033262554));
#452161=CARTESIAN_POINT('Ctrl Pts',(5.30522572107876,26.,-4.44625314528708));
#452162=CARTESIAN_POINT('Ctrl Pts',(5.2889864306648,26.,-4.4493213438557));
#452163=CARTESIAN_POINT('Ctrl Pts',(5.23677996513386,26.,-4.45918506318895));
#452164=CARTESIAN_POINT('Ctrl Pts',(5.18537728348257,26.,-4.47234120946028));
#452165=CARTESIAN_POINT('Ctrl Pts',(5.13511946187084,26.,-4.48880818880732));
#452166=CARTESIAN_POINT('Ctrl Pts',(5.10845853159382,26.,-4.49754364478542));
#452167=CARTESIAN_POINT('Ctrl Pts',(5.08211963724353,26.,-4.50721166236581));
#452168=CARTESIAN_POINT('Ctrl Pts',(5.05615381819268,26.,-4.51782098438608));
#452169=CARTESIAN_POINT('Ctrl Pts',(5.0413405052544,26.,-4.52387352626206));
#452170=CARTESIAN_POINT('Ctrl Pts',(5.02664862375098,26.,-4.53023250440261));
#452171=CARTESIAN_POINT('Ctrl Pts',(5.01208247494515,26.,-4.53689020456271));
#452172=CARTESIAN_POINT('Origin',(5.65685387860011,26.993675081176,5.65685387860011));
#452173=CARTESIAN_POINT('Ctrl Pts',(6.57057130100612,25.868675081176,4.74432962138981));
#452174=CARTESIAN_POINT('Ctrl Pts',(6.60882993708831,25.8656848283261,4.78199706987976));
#452175=CARTESIAN_POINT('Ctrl Pts',(6.92960341635462,25.8388668852448,5.14157728587623));
#452176=CARTESIAN_POINT('Ctrl Pts',(7.09568592881682,25.7882212519322,6.16255878293893));
#452177=CARTESIAN_POINT('Ctrl Pts',(6.01152748645437,25.716738181238,7.13997732676548));
#452178=CARTESIAN_POINT('Ctrl Pts',(4.60259286076204,25.6452551105438,6.75873746207651));
#452179=CARTESIAN_POINT('Ctrl Pts',(4.15947051927595,25.5737720398497,5.36788602689621));
#452180=CARTESIAN_POINT('Ctrl Pts',(5.0882746237623,25.5022889691555,4.24182426511434));
#452181=CARTESIAN_POINT('Ctrl Pts',(6.13675122222029,25.450589982931,4.36502559631504));
#452182=CARTESIAN_POINT('Ctrl Pts',(6.51790892062316,25.4227186869378,4.69148744470697));
#452183=CARTESIAN_POINT('Ctrl Pts',(6.56885365284802,25.418675081176,4.74334636410459));
#452184=CARTESIAN_POINT('Ctrl Pts',(6.56704169373441,25.906324918824,4.74450601134849));
#452185=CARTESIAN_POINT('Ctrl Pts',(6.7750658664325,25.8898945654199,4.9557394479142));
#452186=CARTESIAN_POINT('Ctrl Pts',(7.11639071403833,25.8496365217844,5.64807137163849));
#452187=CARTESIAN_POINT('Ctrl Pts',(6.60321033464885,25.7855507879174,6.8522203629011));
#452188=CARTESIAN_POINT('Ctrl Pts',(5.16550356767203,25.7140677172233,7.1004834147237));
#452189=CARTESIAN_POINT('Ctrl Pts',(4.17707919799325,25.6425846465291,6.0259636415713));
#452190=CARTESIAN_POINT('Ctrl Pts',(4.5448553014618,25.5711015758349,4.61334644908231));
#452191=CARTESIAN_POINT('Ctrl Pts',(5.74896333949311,25.5090149999332,4.21675923787012));
#452192=CARTESIAN_POINT('Ctrl Pts',(6.3830054663296,25.4707561142629,4.5629353888518));
#452193=CARTESIAN_POINT('Ctrl Pts',(6.56829321884323,25.456324918824,4.74640124271564));
#452194=CARTESIAN_POINT('Ctrl Pts',(5.59475217632212,26.,6.69274404704181));
#452195=CARTESIAN_POINT('Ctrl Pts',(5.25011429538726,25.9761723097686,6.67208297724159));
#452196=CARTESIAN_POINT('Ctrl Pts',(4.58904744425369,25.9285169293058,6.25991935236784));
#452197=CARTESIAN_POINT('Ctrl Pts',(4.57111450891619,25.8570338586116,5.08408179813166));
#452198=CARTESIAN_POINT('Ctrl Pts',(5.55001366141289,25.7855507879175,4.43501771280631));
#452199=CARTESIAN_POINT('Ctrl Pts',(6.62575617389683,25.7140677172233,4.90440858615388));
#452200=CARTESIAN_POINT('Ctrl Pts',(6.81433291744693,25.6425846465291,6.06367191307887));
#452201=CARTESIAN_POINT('Ctrl Pts',(5.94217367437589,25.5711015758349,6.8499634587037));
#452202=CARTESIAN_POINT('Ctrl Pts',(4.80874583886255,25.4996185051408,6.54327224197424));
#452203=CARTESIAN_POINT('Ctrl Pts',(4.45227280794999,25.4281354344466,5.42439156223909));
#452204=CARTESIAN_POINT('Ctrl Pts',(5.19945610983427,25.3566523637524,4.51852288527076));
#452205=CARTESIAN_POINT('Ctrl Pts',(6.36568271985868,25.2851692930583,4.65556044151952));
#452206=CARTESIAN_POINT('Ctrl Pts',(6.88249940298929,25.213686222364,5.70997789504277));
#452207=CARTESIAN_POINT('Ctrl Pts',(6.27639179734011,25.1422031516699,6.71571945020394));
#452208=CARTESIAN_POINT('Ctrl Pts',(5.10267450019953,25.0707200809757,6.7513451989237));
#452209=CARTESIAN_POINT('Ctrl Pts',(4.43668748453226,24.9992370102815,5.78421192833874));
#452210=CARTESIAN_POINT('Ctrl Pts',(4.88860074260097,24.9277539395873,4.7003955508837));
#452211=CARTESIAN_POINT('Ctrl Pts',(6.04437662247732,24.8562708688931,4.49287282235237));
#452212=CARTESIAN_POINT('Ctrl Pts',(6.84510966506768,24.784787798199,5.35177365831406));
#452213=CARTESIAN_POINT('Ctrl Pts',(6.55717903824976,24.7133047275048,6.49018471285717));
#452214=CARTESIAN_POINT('Ctrl Pts',(5.44438294256281,24.6418216568106,6.86510957377001));
#452215=CARTESIAN_POINT('Ctrl Pts',(4.52624977050191,24.5703385861164,6.13304718756447));
#452216=CARTESIAN_POINT('Ctrl Pts',(4.64396052187117,24.4988555154223,4.96470306042394));
#452217=CARTESIAN_POINT('Ctrl Pts',(5.68967021074952,24.4273724447281,4.43049797487471));
#452218=CARTESIAN_POINT('Ctrl Pts',(6.70531403099034,24.3558893740339,5.01986328076134));
#452219=CARTESIAN_POINT('Ctrl Pts',(6.76037309820141,24.2844063033397,6.19283059794665));
#452220=CARTESIAN_POINT('Ctrl Pts',(5.80440305573226,24.2129232326455,6.87474342740735));
#452221=CARTESIAN_POINT('Ctrl Pts',(4.71325048867858,24.1414401619514,6.44084262551864));
#452222=CARTESIAN_POINT('Ctrl Pts',(4.48661435222159,24.0699570912572,5.28866213152759));
#452223=CARTESIAN_POINT('Ctrl Pts',(5.33213555135881,23.9984740205631,4.47381384511066));
#452224=CARTESIAN_POINT('Ctrl Pts',(6.47515921171813,23.9269909498688,4.74285054378755));
#452225=CARTESIAN_POINT('Ctrl Pts',(6.86846279219781,23.8555078791747,5.84928450947304));
#452226=CARTESIAN_POINT('Ctrl Pts',(6.15170698086798,23.7840248084805,6.77941618151556));
#452227=CARTESIAN_POINT('Ctrl Pts',(4.98157355760958,23.7125417377863,6.68107173221035));
#452228=CARTESIAN_POINT('Ctrl Pts',(4.43012269359922,23.6410586670921,5.64435299191054));
#452229=CARTESIAN_POINT('Ctrl Pts',(5.00258598787076,23.569575596398,4.61908739135743));
#452230=CARTESIAN_POINT('Ctrl Pts',(6.17448062637044,23.4980925257038,4.54460915448657));
#452231=CARTESIAN_POINT('Ctrl Pts',(6.87213254456038,23.4266094550096,5.48915421344717));
#452232=CARTESIAN_POINT('Ctrl Pts',(6.45636332421143,23.3551263843154,6.5873433994568));
#452233=CARTESIAN_POINT('Ctrl Pts',(5.30809370313679,23.2836433136213,6.8330308949199));
#452234=CARTESIAN_POINT('Ctrl Pts',(4.47935503415496,23.212160242927,6.00112122066856));
#452235=CARTESIAN_POINT('Ctrl Pts',(4.72942128924326,23.1406771722329,4.85379852261456));
#452236=CARTESIAN_POINT('Ctrl Pts',(5.82919498069919,23.0691941015387,4.44222413342345));
#452237=CARTESIAN_POINT('Ctrl Pts',(6.77105943752211,22.9977110308445,5.14347668616413));
#452238=CARTESIAN_POINT('Ctrl Pts',(6.69212899367236,22.9262279601504,6.31507855179966));
#452239=CARTESIAN_POINT('Ctrl Pts',(5.66464494341573,22.8547448894562,6.88362364563197));
#452240=CARTESIAN_POINT('Ctrl Pts',(4.63011853598606,22.783261818762,6.32821994284799));
#452241=CARTESIAN_POINT('Ctrl Pts',(4.53608521045973,22.7117787480678,5.15771839492687));
#452242=CARTESIAN_POINT('Ctrl Pts',(5.46925286619012,22.6402956773736,4.4445208236608));
#452243=CARTESIAN_POINT('Ctrl Pts',(6.57357515235991,22.5688126066795,4.84204067651847));
#452244=CARTESIAN_POINT('Ctrl Pts',(6.8394368280484,22.4973295359852,5.98608844956735));
#452245=CARTESIAN_POINT('Ctrl Pts',(6.01893246982621,22.4258464652911,6.82851835303725));
#452246=CARTESIAN_POINT('Ctrl Pts',(5.25534692011694,22.3781910848283,6.67416374956871));
#452247=CARTESIAN_POINT('Ctrl Pts',(4.99063298333217,22.3543633945969,6.45251384441992));
#452248=CARTESIAN_POINT('Ctrl Pts',(5.58972040746333,26.0485455351344,6.77667668816907));
#452249=CARTESIAN_POINT('Ctrl Pts',(5.21715836192049,26.024717844903,6.75434156236399));
#452250=CARTESIAN_POINT('Ctrl Pts',(4.50252879876621,25.9770624644402,6.30878252293169));
#452251=CARTESIAN_POINT('Ctrl Pts',(4.4831428535712,25.905579393746,5.03767313923882));
#452252=CARTESIAN_POINT('Ctrl Pts',(5.54135696992154,25.8340963230518,4.33601886182374));
#452253=CARTESIAN_POINT('Ctrl Pts',(6.70426114586778,25.7626132523576,4.84344196766209));
#452254=CARTESIAN_POINT('Ctrl Pts',(6.90811725457023,25.6911301816635,6.09663420303223));
#452255=CARTESIAN_POINT('Ctrl Pts',(5.96529161173539,25.6196471109693,6.94663474805762));
#452256=CARTESIAN_POINT('Ctrl Pts',(4.7400281794957,25.5481640402751,6.61509398200833));
#452257=CARTESIAN_POINT('Ctrl Pts',(4.35467204505866,25.4766809695809,5.40555638379146));
#452258=CARTESIAN_POINT('Ctrl Pts',(5.16239561447694,25.4051978988867,4.42629001188529));
#452259=CARTESIAN_POINT('Ctrl Pts',(6.42311533054124,25.3337148281926,4.57443098853515));
#452260=CARTESIAN_POINT('Ctrl Pts',(6.98180690592903,25.2622317574984,5.71428225002475));
#452261=CARTESIAN_POINT('Ctrl Pts',(6.32658964203686,25.1907486868042,6.80151366539291));
#452262=CARTESIAN_POINT('Ctrl Pts',(5.05777230853438,25.11926561611,6.84002597802966));
#452263=CARTESIAN_POINT('Ctrl Pts',(4.33782392622387,25.0477825454159,5.79453107008661));
#452264=CARTESIAN_POINT('Ctrl Pts',(4.82635329907546,24.9762994747217,4.62289884706407));
#452265=CARTESIAN_POINT('Ctrl Pts',(6.07577551821105,24.9048164040275,4.39856166152736));
#452266=CARTESIAN_POINT('Ctrl Pts',(6.94138767747801,24.8333333333333,5.32705463942152));
#452267=CARTESIAN_POINT('Ctrl Pts',(6.63012757162215,24.7618502626391,6.55770505428216));
#452268=CARTESIAN_POINT('Ctrl Pts',(5.42716755876279,24.690367191945,6.96300807183686));
#452269=CARTESIAN_POINT('Ctrl Pts',(4.4346429653087,24.6188841212508,6.17163058503857));
#452270=CARTESIAN_POINT('Ctrl Pts',(4.56189118942602,24.5474010505566,4.90862178076926));
#452271=CARTESIAN_POINT('Ctrl Pts',(5.69232914266462,24.4759179798625,4.33113291369596));
#452272=CARTESIAN_POINT('Ctrl Pts',(6.79026515070139,24.4044349091683,4.96825133880203));
#452273=CARTESIAN_POINT('Ctrl Pts',(6.84978535971091,24.3329518384741,6.23625792548383));
#452274=CARTESIAN_POINT('Ctrl Pts',(5.81635817656469,24.2614687677799,6.97342250511928));
#452275=CARTESIAN_POINT('Ctrl Pts',(4.63679535172919,24.1899856970857,6.50436504145382));
#452276=CARTESIAN_POINT('Ctrl Pts',(4.39179610102783,24.1185026263916,5.2588295230962));
#452277=CARTESIAN_POINT('Ctrl Pts',(5.30582536167067,24.0470195556974,4.37795843727393));
#452278=CARTESIAN_POINT('Ctrl Pts',(6.54146211713177,23.9755364850032,4.66879374102307));
#452279=CARTESIAN_POINT('Ctrl Pts',(6.96663298362319,23.904053414309,5.86487613450725));
#452280=CARTESIAN_POINT('Ctrl Pts',(6.19180228161384,23.8325703436148,6.8703714022368));
#452281=CARTESIAN_POINT('Ctrl Pts',(4.92685920413015,23.7610872729207,6.76405862808226));
#452282=CARTESIAN_POINT('Ctrl Pts',(4.33072722538547,23.6896042022265,5.64334011190815));
#452283=CARTESIAN_POINT('Ctrl Pts',(4.94957415925549,23.6181211315323,4.53500272215098));
#452284=CARTESIAN_POINT('Ctrl Pts',(6.21642115383373,23.5466380608381,4.45448991200439));
#452285=CARTESIAN_POINT('Ctrl Pts',(6.97060007639641,23.475154990144,5.47556640632123));
#452286=CARTESIAN_POINT('Ctrl Pts',(6.52114329936776,23.4036719194498,6.66273598971974));
#452287=CARTESIAN_POINT('Ctrl Pts',(5.27983553104633,23.3321888487556,6.92833022917403));
#452288=CARTESIAN_POINT('Ctrl Pts',(4.38394859923605,23.2607057780614,6.02901536249358));
#452289=CARTESIAN_POINT('Ctrl Pts',(4.6542763857934,23.1892227073672,4.78873124130167));
#452290=CARTESIAN_POINT('Ctrl Pts',(5.84315885864169,23.1177396366731,4.34380918016856));
#452291=CARTESIAN_POINT('Ctrl Pts',(6.86133755596364,23.0462565659789,5.1018804774459));
#452292=CARTESIAN_POINT('Ctrl Pts',(6.77601180031397,22.9747734952847,6.36841097734037));
#452293=CARTESIAN_POINT('Ctrl Pts',(5.66527621173653,22.9032904245905,6.98302223994139));
#452294=CARTESIAN_POINT('Ctrl Pts',(4.54692766144197,22.8318073538963,6.3826171450343));
#452295=CARTESIAN_POINT('Ctrl Pts',(4.4452753183732,22.7603242832022,5.11727611571493));
#452296=CARTESIAN_POINT('Ctrl Pts',(5.45405255931453,22.688841212508,4.34629195893472));
#452297=CARTESIAN_POINT('Ctrl Pts',(6.64785217518362,22.6173581418138,4.77602071980922));
#452298=CARTESIAN_POINT('Ctrl Pts',(6.93525520080945,22.5458750711197,6.01276456633487));
#452299=CARTESIAN_POINT('Ctrl Pts',(6.04826976192828,22.4743920004254,6.92345206015257));
#452300=CARTESIAN_POINT('Ctrl Pts',(5.22281495825156,22.4267366199627,6.75659092854625));
#452301=CARTESIAN_POINT('Ctrl Pts',(4.93665266667552,22.4029089297313,6.5169819168131));
#452302=CARTESIAN_POINT('Ctrl Pts',(5.58468863860454,26.0970910702687,6.86060932929632));
#452303=CARTESIAN_POINT('Ctrl Pts',(5.18420242845371,26.0732633800373,6.83660014748639));
#452304=CARTESIAN_POINT('Ctrl Pts',(4.41601015327873,26.0256079995746,6.35764569349554));
#452305=CARTESIAN_POINT('Ctrl Pts',(4.39517119822623,25.9541249288803,4.99126448034597));
#452306=CARTESIAN_POINT('Ctrl Pts',(5.53270027843017,25.8826418581862,4.23702001084117));
#452307=CARTESIAN_POINT('Ctrl Pts',(6.78276611783875,25.811158787492,4.7824753491703));
#452308=CARTESIAN_POINT('Ctrl Pts',(7.00190159169352,25.7396757167979,6.12959649298558));
#452309=CARTESIAN_POINT('Ctrl Pts',(5.98840954909488,25.6681926461036,7.04330603741155));
#452310=CARTESIAN_POINT('Ctrl Pts',(4.67131052012887,25.5967095754095,6.68691572204241));
#452311=CARTESIAN_POINT('Ctrl Pts',(4.2570712821673,25.5252265047153,5.38672120534384));
#452312=CARTESIAN_POINT('Ctrl Pts',(5.12533511911963,25.4537434340211,4.33405713849982));
#452313=CARTESIAN_POINT('Ctrl Pts',(6.48054794122378,25.382260363327,4.49330153555078));
#452314=CARTESIAN_POINT('Ctrl Pts',(7.0811144088688,25.3107772926328,5.71858660500674));
#452315=CARTESIAN_POINT('Ctrl Pts',(6.37678748673361,25.2392942219386,6.88730788058188));
#452316=CARTESIAN_POINT('Ctrl Pts',(5.01287011686923,25.1678111512444,6.92870675713562));
#452317=CARTESIAN_POINT('Ctrl Pts',(4.23896036791547,25.0963280805502,5.80485021183448));
#452318=CARTESIAN_POINT('Ctrl Pts',(4.76410585554996,25.0248450098561,4.54540214324445));
#452319=CARTESIAN_POINT('Ctrl Pts',(6.10717441394477,24.9533619391619,4.30425050070234));
#452320=CARTESIAN_POINT('Ctrl Pts',(7.03766568988833,24.8818788684677,5.302335620529));
#452321=CARTESIAN_POINT('Ctrl Pts',(6.70307610499455,24.8103957977735,6.62522539570715));
#452322=CARTESIAN_POINT('Ctrl Pts',(5.40995217496278,24.7389127270793,7.06090656990369));
#452323=CARTESIAN_POINT('Ctrl Pts',(4.34303616011548,24.6674296563851,6.21021398251268));
#452324=CARTESIAN_POINT('Ctrl Pts',(4.47982185698087,24.595946585691,4.85254050111457));
#452325=CARTESIAN_POINT('Ctrl Pts',(5.69498807457971,24.5244635149968,4.23176785251722));
#452326=CARTESIAN_POINT('Ctrl Pts',(6.87521627041245,24.4529804443027,4.91663939684271));
#452327=CARTESIAN_POINT('Ctrl Pts',(6.93919762122039,24.3814973736084,6.27968525302103));
#452328=CARTESIAN_POINT('Ctrl Pts',(5.82831329739714,24.3100143029143,7.07210158283119));
#452329=CARTESIAN_POINT('Ctrl Pts',(4.56034021477979,24.2385312322201,6.567887457389));
#452330=CARTESIAN_POINT('Ctrl Pts',(4.29697784983407,24.1670481615259,5.2289969146648));
#452331=CARTESIAN_POINT('Ctrl Pts',(5.27951517198252,24.0955650908318,4.28210302943719));
#452332=CARTESIAN_POINT('Ctrl Pts',(6.60776502254541,24.0240820201375,4.59473693825861));
#452333=CARTESIAN_POINT('Ctrl Pts',(7.06480317504856,23.9525989494434,5.88046775954144));
#452334=CARTESIAN_POINT('Ctrl Pts',(6.2318975823597,23.8811158787492,6.96132662295805));
#452335=CARTESIAN_POINT('Ctrl Pts',(4.87214485065071,23.809632808055,6.84704552395415));
#452336=CARTESIAN_POINT('Ctrl Pts',(4.23133175717171,23.7381497373609,5.64232723190575));
#452337=CARTESIAN_POINT('Ctrl Pts',(4.89656233064023,23.6666666666667,4.45091805294455));
#452338=CARTESIAN_POINT('Ctrl Pts',(6.258361681297,23.5951835959725,4.3643706695222));
#452339=CARTESIAN_POINT('Ctrl Pts',(7.06906760823243,23.5237005252783,5.46197859919531));
#452340=CARTESIAN_POINT('Ctrl Pts',(6.58592327452408,23.4522174545842,6.73812857998267));
#452341=CARTESIAN_POINT('Ctrl Pts',(5.25157735895588,23.3807343838899,7.02362956342815));
#452342=CARTESIAN_POINT('Ctrl Pts',(4.28854216431713,23.3092513131958,6.05690950431861));
#452343=CARTESIAN_POINT('Ctrl Pts',(4.57913148234355,23.2377682425016,4.72366395998878));
#452344=CARTESIAN_POINT('Ctrl Pts',(5.85712273658419,23.1662851718074,4.24539422691366));
#452345=CARTESIAN_POINT('Ctrl Pts',(6.95161567440517,23.0948021011132,5.06028426872769));
#452346=CARTESIAN_POINT('Ctrl Pts',(6.85989460695557,23.0233190304191,6.42174340288107));
#452347=CARTESIAN_POINT('Ctrl Pts',(5.66590748005734,22.9518359597249,7.0824208342508));
#452348=CARTESIAN_POINT('Ctrl Pts',(4.46373678689787,22.8803528890307,6.43701434722061));
#452349=CARTESIAN_POINT('Ctrl Pts',(4.35446542628666,22.8088698183366,5.07683383650298));
#452350=CARTESIAN_POINT('Ctrl Pts',(5.43885225243895,22.7373867476423,4.24806309420865));
#452351=CARTESIAN_POINT('Ctrl Pts',(6.72212919800732,22.6659036769482,4.71000076309996));
#452352=CARTESIAN_POINT('Ctrl Pts',(7.03107357357049,22.594420606254,6.0394406831024));
#452353=CARTESIAN_POINT('Ctrl Pts',(6.07760705403035,22.5229375355598,7.01838576726789));
#452354=CARTESIAN_POINT('Ctrl Pts',(5.19028299638618,22.475282155097,6.83901810752379));
#452355=CARTESIAN_POINT('Ctrl Pts',(4.88267235001886,22.4514544648656,6.58144998920627));
#452356=CARTESIAN_POINT('Ctrl Pts',(5.57965686974575,26.1456366054031,6.94454197042357));
#452357=CARTESIAN_POINT('Ctrl Pts',(5.15124649498693,26.1218089151717,6.91885873260879));
#452358=CARTESIAN_POINT('Ctrl Pts',(4.32949150779126,26.0741535347089,6.40650886405939));
#452359=CARTESIAN_POINT('Ctrl Pts',(4.30719954288124,26.0026704640147,4.94485582145312));
#452360=CARTESIAN_POINT('Ctrl Pts',(5.52404358693882,25.9311873933206,4.1380211598586));
#452361=CARTESIAN_POINT('Ctrl Pts',(6.86127108980971,25.8597043226263,4.7215087306785));
#452362=CARTESIAN_POINT('Ctrl Pts',(7.09568592881682,25.7882212519322,6.16255878293893));
#452363=CARTESIAN_POINT('Ctrl Pts',(6.01152748645437,25.716738181238,7.13997732676548));
#452364=CARTESIAN_POINT('Ctrl Pts',(4.60259286076204,25.6452551105438,6.75873746207651));
#452365=CARTESIAN_POINT('Ctrl Pts',(4.15947051927595,25.5737720398497,5.36788602689621));
#452366=CARTESIAN_POINT('Ctrl Pts',(5.0882746237623,25.5022889691555,4.24182426511434));
#452367=CARTESIAN_POINT('Ctrl Pts',(6.53798055190634,25.4308058984613,4.41217208256641));
#452368=CARTESIAN_POINT('Ctrl Pts',(7.18042191180854,25.3593228277671,5.72289095998872));
#452369=CARTESIAN_POINT('Ctrl Pts',(6.42698533143036,25.287839757073,6.97310209577086));
#452370=CARTESIAN_POINT('Ctrl Pts',(4.96796792520407,25.2163566863788,7.01738753624157));
#452371=CARTESIAN_POINT('Ctrl Pts',(4.14009680960707,25.1448736156846,5.81516935358237));
#452372=CARTESIAN_POINT('Ctrl Pts',(4.70185841202445,25.0733905449904,4.4679054394248));
#452373=CARTESIAN_POINT('Ctrl Pts',(6.13857330967851,25.0019074742962,4.20993933987732));
#452374=CARTESIAN_POINT('Ctrl Pts',(7.13394370229865,24.930424403602,5.27761660163647));
#452375=CARTESIAN_POINT('Ctrl Pts',(6.77602463836695,24.8589413329079,6.69274573713214));
#452376=CARTESIAN_POINT('Ctrl Pts',(5.39273679116275,24.7874582622137,7.15880506797054));
#452377=CARTESIAN_POINT('Ctrl Pts',(4.25142935492228,24.7159751915195,6.24879737998678));
#452378=CARTESIAN_POINT('Ctrl Pts',(4.39775252453571,24.6444921208253,4.79645922145989));
#452379=CARTESIAN_POINT('Ctrl Pts',(5.69764700649482,24.5730090501312,4.13240279133847));
#452380=CARTESIAN_POINT('Ctrl Pts',(6.9601673901235,24.501525979437,4.86502745488341));
#452381=CARTESIAN_POINT('Ctrl Pts',(7.0286098827299,24.4300429087428,6.32311258055822));
#452382=CARTESIAN_POINT('Ctrl Pts',(5.84026841822956,24.3585598380486,7.17078066054311));
#452383=CARTESIAN_POINT('Ctrl Pts',(4.4838850778304,24.2870767673545,6.63140987332417));
#452384=CARTESIAN_POINT('Ctrl Pts',(4.2021595986403,24.2155936966603,5.19916430623342));
#452385=CARTESIAN_POINT('Ctrl Pts',(5.25320498229437,24.1441106259661,4.18624762160046));
#452386=CARTESIAN_POINT('Ctrl Pts',(6.67406792795905,24.0726275552719,4.52068013549415));
#452387=CARTESIAN_POINT('Ctrl Pts',(7.16297336647392,24.0011444845777,5.89605938457563));
#452388=CARTESIAN_POINT('Ctrl Pts',(6.27199288310558,23.9296614138836,7.0522818436793));
#452389=CARTESIAN_POINT('Ctrl Pts',(4.81743049717126,23.8581783431894,6.93003241982605));
#452390=CARTESIAN_POINT('Ctrl Pts',(4.13193628895796,23.7866952724952,5.64131435190337));
#452391=CARTESIAN_POINT('Ctrl Pts',(4.84355050202496,23.715212201801,4.3668333837381));
#452392=CARTESIAN_POINT('Ctrl Pts',(6.30030220876029,23.6437291311069,4.27425142704003));
#452393=CARTESIAN_POINT('Ctrl Pts',(7.16753514006844,23.5722460604127,5.44839079206937));
#452394=CARTESIAN_POINT('Ctrl Pts',(6.65070324968042,23.5007629897185,6.81352117024561));
#452395=CARTESIAN_POINT('Ctrl Pts',(5.22331918686542,23.4292799190243,7.11892889768229));
#452396=CARTESIAN_POINT('Ctrl Pts',(4.19313572939823,23.3577968483302,6.08480364614363));
#452397=CARTESIAN_POINT('Ctrl Pts',(4.50398657889369,23.2863137776359,4.65859667867589));
#452398=CARTESIAN_POINT('Ctrl Pts',(5.8710866145267,23.2148307069418,4.14697927365876));
#452399=CARTESIAN_POINT('Ctrl Pts',(7.04189379284668,23.1433476362476,5.01868806000948));
#452400=CARTESIAN_POINT('Ctrl Pts',(6.94377741359718,23.0718645655535,6.47507582842176));
#452401=CARTESIAN_POINT('Ctrl Pts',(5.66653874837814,23.0003814948592,7.18181942856023));
#452402=CARTESIAN_POINT('Ctrl Pts',(4.38054591235378,22.9288984241651,6.49141154940691));
#452403=CARTESIAN_POINT('Ctrl Pts',(4.26365553420012,22.8574153534709,5.03639155729104));
#452404=CARTESIAN_POINT('Ctrl Pts',(5.42365194556336,22.7859322827767,4.14983422948258));
#452405=CARTESIAN_POINT('Ctrl Pts',(6.79640622083105,22.7144492120825,4.6439808063907));
#452406=CARTESIAN_POINT('Ctrl Pts',(7.12689194633153,22.6429661413884,6.06611679986992));
#452407=CARTESIAN_POINT('Ctrl Pts',(6.10694434613243,22.5714830706942,7.11331947438321));
#452408=CARTESIAN_POINT('Ctrl Pts',(5.15775103452081,22.5238276902314,6.92144528650133));
#452409=CARTESIAN_POINT('Ctrl Pts',(4.8286920333622,22.5,6.64591806159944));
#452410=CARTESIAN_POINT('Ctrl Pts',(4.8286920333622,22.5,6.64591806159944));
#452411=CARTESIAN_POINT('Ctrl Pts',(4.8719367804586,22.5,6.6755807993511));
#452412=CARTESIAN_POINT('Ctrl Pts',(4.91697381282208,22.5,6.7022744086721));
#452413=CARTESIAN_POINT('Ctrl Pts',(4.96347942286292,22.5,6.72600910610866));
#452414=CARTESIAN_POINT('Ctrl Pts',(5.01052630347802,22.5,6.750020047493));
#452415=CARTESIAN_POINT('Ctrl Pts',(5.05907736675444,22.5,6.77100289981649));
#452416=CARTESIAN_POINT('Ctrl Pts',(5.10881343934042,22.5,6.78891649180094));
#452417=CARTESIAN_POINT('Ctrl Pts',(5.14478450961691,22.5,6.80187230118985));
#452418=CARTESIAN_POINT('Ctrl Pts',(5.18137581815852,22.5,6.81322157811539));
#452419=CARTESIAN_POINT('Ctrl Pts',(5.21846626007043,22.5,6.82293175279788));
#452420=CARTESIAN_POINT('Ctrl Pts',(5.23435307151024,22.5,6.82709087591091));
#452421=CARTESIAN_POINT('Ctrl Pts',(5.25033142515782,22.5,6.83094910537833));
#452422=CARTESIAN_POINT('Ctrl Pts',(5.26639159475908,22.5,6.83450307899072));
#452423=CARTESIAN_POINT('Ctrl Pts',(5.27631910355995,22.5,6.83669994896103));
#452424=CARTESIAN_POINT('Ctrl Pts',(5.28627904830748,22.5,6.83878067254843));
#452425=CARTESIAN_POINT('Ctrl Pts',(5.29625198803563,22.5,6.8407413340506));
#452426=CARTESIAN_POINT('Ctrl Pts',(5.34683220766748,22.5,6.8506853116647));
#452427=CARTESIAN_POINT('Ctrl Pts',(5.39784710619139,22.5,6.85756855483867));
#452428=CARTESIAN_POINT('Ctrl Pts',(5.44899668904261,22.5,6.86136063349203));
#452429=CARTESIAN_POINT('Ctrl Pts',(5.4989795280052,22.5,6.86506621320742));
#452430=CARTESIAN_POINT('Ctrl Pts',(5.5490920296864,22.5,6.86581982211597));
#452431=CARTESIAN_POINT('Ctrl Pts',(5.59904614057211,22.5,6.86354521214504));
#452432=CARTESIAN_POINT('Ctrl Pts',(5.63380176660143,22.5,6.86196264982713));
#452433=CARTESIAN_POINT('Ctrl Pts',(5.66848055894767,22.5,6.8589132351154));
#452434=CARTESIAN_POINT('Ctrl Pts',(5.70297915970175,22.5,6.85435789423314));
#452435=CARTESIAN_POINT('Ctrl Pts',(5.71516099278645,22.5,6.85274935356602));
#452436=CARTESIAN_POINT('Ctrl Pts',(5.72732029612368,22.5,6.85095294339145));
#452437=CARTESIAN_POINT('Ctrl Pts',(5.73945229469627,22.5,6.84896661767721));
#452438=CARTESIAN_POINT('Ctrl Pts',(5.74841196470285,22.5,6.84749968518305));
#452439=CARTESIAN_POINT('Ctrl Pts',(5.75735562780225,22.5,6.84592925290685));
#452440=CARTESIAN_POINT('Ctrl Pts',(5.76626920948405,22.5,6.84425708000572));
#452441=CARTESIAN_POINT('Ctrl Pts',(5.81380349733577,22.5,6.83533972771596));
#452442=CARTESIAN_POINT('Ctrl Pts',(5.86057802478339,22.5,6.82351786783565));
#452443=CARTESIAN_POINT('Ctrl Pts',(5.90632961568247,22.5,6.80873145101255));
#452444=CARTESIAN_POINT('Ctrl Pts',(5.93907832139669,22.5,6.79814742532969));
#452445=CARTESIAN_POINT('Ctrl Pts',(5.97130269582608,22.5,6.78604349575646));
#452446=CARTESIAN_POINT('Ctrl Pts',(6.00289829431615,22.5,6.77238316128915));
#452447=CARTESIAN_POINT('Ctrl Pts',(6.0450043450931,22.5,6.75417864027363));
#452448=CARTESIAN_POINT('Ctrl Pts',(6.08599501913005,22.5,6.73321019789003));
#452449=CARTESIAN_POINT('Ctrl Pts',(6.12568011956913,22.5,6.70966855565445));
#452450=CARTESIAN_POINT('Ctrl Pts',(6.13614447303852,22.5,6.7034609849824));
#452451=CARTESIAN_POINT('Ctrl Pts',(6.14651787724421,22.5,6.69707438313333));
#452452=CARTESIAN_POINT('Ctrl Pts',(6.1567964532414,22.5,6.69051202329594));
#452453=CARTESIAN_POINT('Ctrl Pts',(6.1645478556042,22.5,6.68556313820106));
#452454=CARTESIAN_POINT('Ctrl Pts',(6.17224531908615,22.5,6.68051415741144));
#452455=CARTESIAN_POINT('Ctrl Pts',(6.17987521950616,22.5,6.67537489370653));
#452456=CARTESIAN_POINT('Ctrl Pts',(6.21988616021516,22.5,6.64842476800822));
#452457=CARTESIAN_POINT('Ctrl Pts',(6.25812741389502,22.5,6.61894162118579));
#452458=CARTESIAN_POINT('Ctrl Pts',(6.29441170508163,22.5,6.58718324857477));
#452459=CARTESIAN_POINT('Ctrl Pts',(6.33059687379256,22.5,6.55551163440422));
#452460=CARTESIAN_POINT('Ctrl Pts',(6.36483641843439,22.5,6.52157609274862));
#452461=CARTESIAN_POINT('Ctrl Pts',(6.39690234758754,22.5,6.48560329463389));
#452462=CARTESIAN_POINT('Ctrl Pts',(6.41407247164262,22.5,6.46634118614209));
#452463=CARTESIAN_POINT('Ctrl Pts',(6.4306185942519,22.5,6.44649455990001));
#452464=CARTESIAN_POINT('Ctrl Pts',(6.44649972121378,22.5,6.42609644704949));
#452465=CARTESIAN_POINT('Ctrl Pts',(6.45474860376629,22.5,6.41550137797154));
#452466=CARTESIAN_POINT('Ctrl Pts',(6.4628180032753,22.5,6.40475750978787));
#452467=CARTESIAN_POINT('Ctrl Pts',(6.47070167883221,22.5,6.39386942293182));
#452468=CARTESIAN_POINT('Ctrl Pts',(6.47674054415646,22.5,6.38552919004326));
#452469=CARTESIAN_POINT('Ctrl Pts',(6.48267052688883,22.5,6.37710396981869));
#452470=CARTESIAN_POINT('Ctrl Pts',(6.48848046699456,22.5,6.3686084992472));
#452471=CARTESIAN_POINT('Ctrl Pts',(6.51462321287319,22.5,6.33038178361366));
#452472=CARTESIAN_POINT('Ctrl Pts',(6.53838419602365,22.5,6.29067294990532));
#452473=CARTESIAN_POINT('Ctrl Pts',(6.55954587128772,22.5,6.24968947065537));
#452474=CARTESIAN_POINT('Ctrl Pts',(6.57382078988697,22.5,6.22204346329034));
#452475=CARTESIAN_POINT('Ctrl Pts',(6.58691199084907,22.5,6.19381707848861));
#452476=CARTESIAN_POINT('Ctrl Pts',(6.59873928456135,22.5,6.16507260006602));
#452477=CARTESIAN_POINT('Ctrl Pts',(6.60384497627704,22.5,6.15266397566519));
#452478=CARTESIAN_POINT('Ctrl Pts',(6.6087155221976,22.5,6.14015674565985));
#452479=CARTESIAN_POINT('Ctrl Pts',(6.61333659561112,22.5,6.12757735912736));
#452480=CARTESIAN_POINT('Ctrl Pts',(6.6285399411254,22.5,6.08619113936898));
#452481=CARTESIAN_POINT('Ctrl Pts',(6.64106838659551,22.5,6.04397428614735));
#452482=CARTESIAN_POINT('Ctrl Pts',(6.65070263630215,22.5,6.00111091245467));
#452483=CARTESIAN_POINT('Ctrl Pts',(6.65546745351706,22.5,5.9799119455316));
#452484=CARTESIAN_POINT('Ctrl Pts',(6.65952358177373,22.5,5.9585548202981));
#452485=CARTESIAN_POINT('Ctrl Pts',(6.66283972884874,22.5,5.93706218561481));
#452486=CARTESIAN_POINT('Ctrl Pts',(6.66481534816931,22.5,5.92425778841234));
#452487=CARTESIAN_POINT('Ctrl Pts',(6.6665282555788,22.5,5.91140530098883));
#452488=CARTESIAN_POINT('Ctrl Pts',(6.66798006829994,22.5,5.89851203167795));
#452489=CARTESIAN_POINT('Ctrl Pts',(6.39051881327128,25.2730384757729,4.92197603118329));
#452490=CARTESIAN_POINT('Ctrl Pts',(6.34953594825859,25.2770820815347,4.8802577415671));
#452491=CARTESIAN_POINT('Ctrl Pts',(6.3050503566324,25.2811256872965,4.84215579969383));
#452492=CARTESIAN_POINT('Ctrl Pts',(6.25744773204304,25.2851692930582,4.80845709106527));
#452493=CARTESIAN_POINT('Ctrl Pts',(5.97694051651721,25.3089969832896,4.60988125610327));
#452494=CARTESIAN_POINT('Ctrl Pts',(5.58819831317574,25.332824673521,4.56420207068701));
#452495=CARTESIAN_POINT('Ctrl Pts',(5.26929666119096,25.3566523637524,4.69234059080694));
#452496=CARTESIAN_POINT('Ctrl Pts',(4.95039500920618,25.3804800539838,4.82047911092687));
#452497=CARTESIAN_POINT('Ctrl Pts',(4.70133390857808,25.4043077442152,5.12243533658298));
#452498=CARTESIAN_POINT('Ctrl Pts',(4.6362155300828,25.4281354344466,5.45989356270023));
#452499=CARTESIAN_POINT('Ctrl Pts',(4.57109715158751,25.451963124678,5.79735178881747));
#452500=CARTESIAN_POINT('Ctrl Pts',(4.68992149522503,25.4757908149094,6.17031201539585));
#452501=CARTESIAN_POINT('Ctrl Pts',(4.93823830629601,25.4996185051408,6.40790733147329));
#452502=CARTESIAN_POINT('Ctrl Pts',(5.186555117367,25.5234461953722,6.64550264755072));
#452503=CARTESIAN_POINT('Ctrl Pts',(5.56436439587144,25.5472738856035,6.74773305312721));
#452504=CARTESIAN_POINT('Ctrl Pts',(5.89862890896884,25.5711015758349,6.66779966497798));
#452505=CARTESIAN_POINT('Ctrl Pts',(6.23289342206624,25.5949292660663,6.58786627682875));
#452506=CARTESIAN_POINT('Ctrl Pts',(6.52361316975658,25.6187569562977,6.32576909495381));
#452507=CARTESIAN_POINT('Ctrl Pts',(6.63754358634341,25.6425846465291,6.00150994952884));
#452508=CARTESIAN_POINT('Ctrl Pts',(6.75147400293023,25.6664123367605,5.67725080410387));
#452509=CARTESIAN_POINT('Ctrl Pts',(6.68861508841353,25.6902400269919,5.29082969512888));
#452510=CARTESIAN_POINT('Ctrl Pts',(6.47789521240786,25.7140677172233,5.01938732841678));
#452511=CARTESIAN_POINT('Ctrl Pts',(6.45145094929911,25.7170579700732,4.98532270432787));
#452512=CARTESIAN_POINT('Ctrl Pts',(6.42267802952733,25.720048222923,4.95306887608107));
#452513=CARTESIAN_POINT('Ctrl Pts',(6.39190058798136,25.7230384757729,4.92276701974739));
#452514=CARTESIAN_POINT('Ctrl Pts',(5.01302286563431,26.,4.53900700771688));
#452515=CARTESIAN_POINT('Ctrl Pts',(5.38492752167559,25.9761723097686,4.32480615636363));
#452516=CARTESIAN_POINT('Ctrl Pts',(6.35301914505848,25.9285169293058,4.30067277954968));
#452517=CARTESIAN_POINT('Ctrl Pts',(7.17562648915451,25.8570338586117,5.50907794609548));
#452518=CARTESIAN_POINT('Ctrl Pts',(6.60321033464885,25.7855507879174,6.8522203629011));
#452519=CARTESIAN_POINT('Ctrl Pts',(5.16550356767203,25.7140677172233,7.1004834147237));
#452520=CARTESIAN_POINT('Ctrl Pts',(4.17707919799325,25.6425846465291,6.0259636415713));
#452521=CARTESIAN_POINT('Ctrl Pts',(4.5448553014618,25.5711015758349,4.61334644908231));
#452522=CARTESIAN_POINT('Ctrl Pts',(5.93119910857215,25.4996185051408,4.15673773385264));
#452523=CARTESIAN_POINT('Ctrl Pts',(7.06630891143689,25.4281354344466,5.07453447980768));
#452524=CARTESIAN_POINT('Ctrl Pts',(6.91003560334641,25.3566523637524,6.5258341885166));
#452525=CARTESIAN_POINT('Ctrl Pts',(5.60564496305,25.2851692930582,7.18099123031483));
#452526=CARTESIAN_POINT('Ctrl Pts',(4.34815567114858,25.213686222364,6.43975200870338));
#452527=CARTESIAN_POINT('Ctrl Pts',(4.28968558428151,25.1422031516699,4.98123363545819));
#452528=CARTESIAN_POINT('Ctrl Pts',(5.48379221455872,25.0707200809757,4.14170854437417));
#452529=CARTESIAN_POINT('Ctrl Pts',(6.8364576202828,24.9992370102815,4.69033908735646));
#452530=CARTESIAN_POINT('Ctrl Pts',(7.10838527255517,24.9277539395874,6.12447699388039));
#452531=CARTESIAN_POINT('Ctrl Pts',(6.05044038944422,24.8562708688931,7.13018513270865));
#452532=CARTESIAN_POINT('Ctrl Pts',(4.63189669239788,24.784787798199,6.78604742232837));
#452533=CARTESIAN_POINT('Ctrl Pts',(4.15240479236238,24.7133047275048,5.40735816264999));
#452534=CARTESIAN_POINT('Ctrl Pts',(5.0512683537124,24.6418216568106,4.25725342975252));
#452535=CARTESIAN_POINT('Ctrl Pts',(6.50496106867921,24.5703385861164,4.38944335790392));
#452536=CARTESIAN_POINT('Ctrl Pts',(7.18162963832199,24.4988555154223,5.68281734635597));
#452537=CARTESIAN_POINT('Ctrl Pts',(6.46131966662841,24.4273724447281,6.95240396480877));
#452538=CARTESIAN_POINT('Ctrl Pts',(5.00396921476326,24.3558893740339,7.03502543671246));
#452539=CARTESIAN_POINT('Ctrl Pts',(4.14478270244581,24.2844063033397,5.85498510857851));
#452540=CARTESIAN_POINT('Ctrl Pts',(4.67093497503136,24.2129232326456,4.49341967622111));
#452541=CARTESIAN_POINT('Ctrl Pts',(6.10037256921808,24.1414401619514,4.19777663638434));
#452542=CARTESIAN_POINT('Ctrl Pts',(7.12346444664167,24.0699570912572,5.23892007073304));
#452543=CARTESIAN_POINT('Ctrl Pts',(6.80286792203874,23.998474020563,6.662968703113));
#452544=CARTESIAN_POINT('Ctrl Pts',(5.43230911237055,23.9269909498688,7.16522879152533));
#452545=CARTESIAN_POINT('Ctrl Pts',(4.26747512907024,23.8555078791747,6.2855365564656));
#452546=CARTESIAN_POINT('Ctrl Pts',(4.37557081254884,23.7840248084805,4.82985391579145));
#452547=CARTESIAN_POINT('Ctrl Pts',(5.6575604101698,23.7125417377863,4.13185724083954));
#452548=CARTESIAN_POINT('Ctrl Pts',(6.93890266242659,23.6410586670921,4.83104150205929));
#452549=CARTESIAN_POINT('Ctrl Pts',(7.04564953674368,23.569575596398,6.28682364983267));
#452550=CARTESIAN_POINT('Ctrl Pts',(5.88000083782648,23.4980925257038,7.16543624640093));
#452551=CARTESIAN_POINT('Ctrl Pts',(4.50990820099156,23.4266094550096,6.66190630419616));
#452552=CARTESIAN_POINT('Ctrl Pts',(4.19063094092434,23.3551263843154,5.23756146736659));
#452553=CARTESIAN_POINT('Ctrl Pts',(5.21468783779196,23.2836433136212,4.19736598356862));
#452554=CARTESIAN_POINT('Ctrl Pts',(6.64384941569999,23.2121602429271,4.49433434427902));
#452555=CARTESIAN_POINT('Ctrl Pts',(7.16874271925581,23.1406771722329,5.85638486317849));
#452556=CARTESIAN_POINT('Ctrl Pts',(6.30845753745629,23.0691941015387,7.03563221165043));
#452557=CARTESIAN_POINT('Ctrl Pts',(4.85119529970875,22.9977110308445,6.95165327175697));
#452558=CARTESIAN_POINT('Ctrl Pts',(4.13204038713623,22.9262279601503,5.68141376558384));
#452559=CARTESIAN_POINT('Ctrl Pts',(4.80994952176022,22.8547448894562,4.38863987327371));
#452560=CARTESIAN_POINT('Ctrl Pts',(6.26368089065206,22.783261818762,4.25785081625158));
#452561=CARTESIAN_POINT('Ctrl Pts',(7.16164157512573,22.7117787480678,5.40868234342553));
#452562=CARTESIAN_POINT('Ctrl Pts',(6.68055232418451,22.6402956773736,6.78713386963137));
#452563=CARTESIAN_POINT('Ctrl Pts',(5.26231872215201,22.5688126066795,7.12954990426925));
#452564=CARTESIAN_POINT('Ctrl Pts',(4.20406666678212,22.4973295359853,6.12366999440581));
#452565=CARTESIAN_POINT('Ctrl Pts',(4.47983331463011,22.4258464652911,4.68809392709694));
#452566=CARTESIAN_POINT('Ctrl Pts',(5.37807265034296,22.3781910848283,4.32622391325397));
#452567=CARTESIAN_POINT('Ctrl Pts',(5.80443435631943,22.3543633945969,4.37532354240196));
#452568=CARTESIAN_POINT('Ctrl Pts',(5.05498833669907,26.0485455351344,4.61186924884874));
#452569=CARTESIAN_POINT('Ctrl Pts',(5.40265192052163,26.024717844903,4.41163019717349));
#452570=CARTESIAN_POINT('Ctrl Pts',(6.30764248137266,25.9770624644402,4.38906985506272));
#452571=CARTESIAN_POINT('Ctrl Pts',(7.07663155607638,25.905579393746,5.51871011120511));
#452572=CARTESIAN_POINT('Ctrl Pts',(6.54152598941931,25.8340963230518,6.77430532526158));
#452573=CARTESIAN_POINT('Ctrl Pts',(5.1975302126156,25.7626132523576,7.00638637325414));
#452574=CARTESIAN_POINT('Ctrl Pts',(4.27353221173564,25.6911301816635,6.00190474293836));
#452575=CARTESIAN_POINT('Ctrl Pts',(4.61733634566934,25.6196471109693,4.68136318011483));
#452576=CARTESIAN_POINT('Ctrl Pts',(5.91331704545575,25.5481640402751,4.25451662209878));
#452577=CARTESIAN_POINT('Ctrl Pts',(6.97443939411569,25.4766809695809,5.11249056981941));
#452578=CARTESIAN_POINT('Ctrl Pts',(6.82835211754091,25.4051978988868,6.46919328847101));
#452579=CARTESIAN_POINT('Ctrl Pts',(5.60898280515531,25.3337148281926,7.08164661869467));
#452580=CARTESIAN_POINT('Ctrl Pts',(4.43345777007097,25.2622317574984,6.38872202076577));
#452581=CARTESIAN_POINT('Ctrl Pts',(4.37879881483496,25.1907486868042,5.02527115647435));
#452582=CARTESIAN_POINT('Ctrl Pts',(5.49507252586478,25.1192656161101,4.24046704839446));
#452583=CARTESIAN_POINT('Ctrl Pts',(6.75957001205555,25.0477825454158,4.75333737058416));
#452584=CARTESIAN_POINT('Ctrl Pts',(7.01377318104996,24.9762994747217,6.09399690839474));
#452585=CARTESIAN_POINT('Ctrl Pts',(6.0247860748808,24.9048164040275,7.03415210716631));
#452586=CARTESIAN_POINT('Ctrl Pts',(4.69870430227373,24.8333333333333,6.71244559509181));
#452587=CARTESIAN_POINT('Ctrl Pts',(4.25046610554157,24.7618502626392,5.42362051261082));
#452588=CARTESIAN_POINT('Ctrl Pts',(5.09074095026354,24.6903671919449,4.34848061663154));
#452589=CARTESIAN_POINT('Ctrl Pts',(6.44968069692276,24.6188841212508,4.47205428913018));
#452590=CARTESIAN_POINT('Ctrl Pts',(7.08224341470704,24.5474010505566,5.68112502471735));
#452591=CARTESIAN_POINT('Ctrl Pts',(6.40888387979891,24.4759179798625,6.86795887198032));
#452592=CARTESIAN_POINT('Ctrl Pts',(5.04652481074591,24.4044349091682,6.94519500375797));
#452593=CARTESIAN_POINT('Ctrl Pts',(4.24334083014217,24.3329518384741,5.84207074093976));
#452594=CARTESIAN_POINT('Ctrl Pts',(4.73519803534796,24.2614687677799,4.56925333967074));
#452595=CARTESIAN_POINT('Ctrl Pts',(6.07146363130893,24.1899856970857,4.29288057290862));
#452596=CARTESIAN_POINT('Ctrl Pts',(7.02786948132165,24.1185026263916,5.2661613635068));
#452597=CARTESIAN_POINT('Ctrl Pts',(6.72816971985337,24.0470195556973,6.59738925492609));
#452598=CARTESIAN_POINT('Ctrl Pts',(5.44694513750786,23.9755364850032,7.0669115895136));
#452599=CARTESIAN_POINT('Ctrl Pts',(4.35803605660743,23.904053414309,6.2445584671913));
#452600=CARTESIAN_POINT('Ctrl Pts',(4.45908596846911,23.8325703436148,4.88375849993059));
#452601=CARTESIAN_POINT('Ctrl Pts',(5.65751435782136,23.7610872729207,4.2312578614791));
#452602=CARTESIAN_POINT('Ctrl Pts',(6.85533759634902,23.6896042022265,4.88486867828213));
#452603=CARTESIAN_POINT('Ctrl Pts',(6.95512661561532,23.6181211315323,6.24576166668191));
#452604=CARTESIAN_POINT('Ctrl Pts',(5.86545592297768,23.5466380608381,7.06710552229816));
#452605=CARTESIAN_POINT('Ctrl Pts',(4.58466712791062,23.475154990144,6.59639610410402));
#452606=CARTESIAN_POINT('Ctrl Pts',(4.28620064015657,23.4036719194498,5.26489131510138));
#452607=CARTESIAN_POINT('Ctrl Pts',(5.24350860879812,23.3321888487556,4.2924966868042));
#452608=CARTESIAN_POINT('Ctrl Pts',(6.57951617946397,23.2607057780614,4.57010838886106));
#452609=CARTESIAN_POINT('Ctrl Pts',(7.07019647634743,23.1892227073672,5.84337925830513));
#452610=CARTESIAN_POINT('Ctrl Pts',(6.26598543850372,23.1177396366731,6.94576222857241));
#452611=CARTESIAN_POINT('Ctrl Pts',(4.90370883369462,23.0462565659789,6.86725710976116));
#452612=CARTESIAN_POINT('Ctrl Pts',(4.23142907013928,22.9747734952847,5.67981293057308));
#452613=CARTESIAN_POINT('Ctrl Pts',(4.86515149178938,22.9032904245905,4.47130317633407));
#452614=CARTESIAN_POINT('Ctrl Pts',(6.22412737287685,22.8318073538963,4.34903906495375));
#452615=CARTESIAN_POINT('Ctrl Pts',(7.06355819103049,22.7603242832022,5.42485838212006));
#452616=CARTESIAN_POINT('Ctrl Pts',(6.613826760128,22.688841212508,6.7134612268051));
#452617=CARTESIAN_POINT('Ctrl Pts',(5.28803487026933,22.6173581418138,7.03355828347467));
#452618=CARTESIAN_POINT('Ctrl Pts',(4.29876061359894,22.5458750711196,6.0932425098549));
#452619=CARTESIAN_POINT('Ctrl Pts',(4.55655254906459,22.4743920004255,4.75123855184286));
#452620=CARTESIAN_POINT('Ctrl Pts',(5.39624385572484,22.4267366199627,4.41295554342414));
#452621=CARTESIAN_POINT('Ctrl Pts',(5.79481493112442,22.4029089297313,4.45885481560765));
#452622=CARTESIAN_POINT('Ctrl Pts',(5.09695380776383,26.0970910702687,4.6847314899806));
#452623=CARTESIAN_POINT('Ctrl Pts',(5.42037631936769,26.0732633800373,4.49845423798335));
#452624=CARTESIAN_POINT('Ctrl Pts',(6.26226581768684,26.0256079995745,4.47746693057576));
#452625=CARTESIAN_POINT('Ctrl Pts',(6.97763662299825,25.9541249288804,5.52834227631475));
#452626=CARTESIAN_POINT('Ctrl Pts',(6.47984164418979,25.8826418581862,6.69639028762206));
#452627=CARTESIAN_POINT('Ctrl Pts',(5.22955685755916,25.811158787492,6.91228933178459));
#452628=CARTESIAN_POINT('Ctrl Pts',(4.36998522547805,25.7396757167978,5.97784584430541));
#452629=CARTESIAN_POINT('Ctrl Pts',(4.68981738987686,25.6681926461037,4.74937991114736));
#452630=CARTESIAN_POINT('Ctrl Pts',(5.89543498233936,25.5967095754095,4.35229551034491));
#452631=CARTESIAN_POINT('Ctrl Pts',(6.88256987679448,25.5252265047153,5.15044665983115));
#452632=CARTESIAN_POINT('Ctrl Pts',(6.74666863173542,25.4537434340211,6.41255238842542));
#452633=CARTESIAN_POINT('Ctrl Pts',(5.61232064726061,25.3822603633269,6.9823020070745));
#452634=CARTESIAN_POINT('Ctrl Pts',(4.51875986899336,25.3107772926328,6.33769203282816));
#452635=CARTESIAN_POINT('Ctrl Pts',(4.46791204538842,25.2392942219386,5.06930867749052));
#452636=CARTESIAN_POINT('Ctrl Pts',(5.50635283717083,25.1678111512444,4.33922555241474));
#452637=CARTESIAN_POINT('Ctrl Pts',(6.68268240382831,25.0963280805502,4.81633565381187));
#452638=CARTESIAN_POINT('Ctrl Pts',(6.91916108954474,25.0248450098561,6.06351682290909));
#452639=CARTESIAN_POINT('Ctrl Pts',(5.99913176031738,24.9533619391618,6.93811908162396));
#452640=CARTESIAN_POINT('Ctrl Pts',(4.76551191214957,24.8818788684677,6.63884376785527));
#452641=CARTESIAN_POINT('Ctrl Pts',(4.34852741872076,24.8103957977735,5.43988286257165));
#452642=CARTESIAN_POINT('Ctrl Pts',(5.13021354681469,24.7389127270793,4.43970780351056));
#452643=CARTESIAN_POINT('Ctrl Pts',(6.39440032516631,24.6674296563851,4.55466522035643));
#452644=CARTESIAN_POINT('Ctrl Pts',(6.9828571910921,24.595946585691,5.67943270307875));
#452645=CARTESIAN_POINT('Ctrl Pts',(6.35644809296942,24.5244635149968,6.78351377915185));
#452646=CARTESIAN_POINT('Ctrl Pts',(5.08908040672856,24.4529804443026,6.8553645708035));
#452647=CARTESIAN_POINT('Ctrl Pts',(4.34189895783853,24.3814973736085,5.82915637330097));
#452648=CARTESIAN_POINT('Ctrl Pts',(4.79946109566455,24.3100143029142,4.64508700312038));
#452649=CARTESIAN_POINT('Ctrl Pts',(6.0425546933998,24.2385312322201,4.38798450943289));
#452650=CARTESIAN_POINT('Ctrl Pts',(6.93227451600162,24.1670481615259,5.29340265628057));
#452651=CARTESIAN_POINT('Ctrl Pts',(6.65347151766801,24.0955650908317,6.53180980673917));
#452652=CARTESIAN_POINT('Ctrl Pts',(5.46158116264517,24.0240820201376,6.96859438750187));
#452653=CARTESIAN_POINT('Ctrl Pts',(4.44859698414461,23.9525989494434,6.20358037791699));
#452654=CARTESIAN_POINT('Ctrl Pts',(4.54260112438938,23.8811158787492,4.93766308406974));
#452655=CARTESIAN_POINT('Ctrl Pts',(5.65746830547292,23.809632808055,4.33065848211867));
#452656=CARTESIAN_POINT('Ctrl Pts',(6.77177253027144,23.7381497373608,4.93869585450498));
#452657=CARTESIAN_POINT('Ctrl Pts',(6.86460369448697,23.6666666666667,6.20469968353116));
#452658=CARTESIAN_POINT('Ctrl Pts',(5.85091100812889,23.5951835959725,6.96877479819537));
#452659=CARTESIAN_POINT('Ctrl Pts',(4.65942605482967,23.5237005252783,6.53088590401187));
#452660=CARTESIAN_POINT('Ctrl Pts',(4.3817703393888,23.4522174545841,5.29222116283617));
#452661=CARTESIAN_POINT('Ctrl Pts',(5.27232937980428,23.38073438389,4.38762739003978));
#452662=CARTESIAN_POINT('Ctrl Pts',(6.51518294322793,23.3092513131958,4.6458824334431));
#452663=CARTESIAN_POINT('Ctrl Pts',(6.97165023343906,23.2377682425016,5.83037365343178));
#452664=CARTESIAN_POINT('Ctrl Pts',(6.22351333955115,23.1662851718074,6.85589224549438));
#452665=CARTESIAN_POINT('Ctrl Pts',(4.9562223676805,23.0948021011132,6.78286094776533));
#452666=CARTESIAN_POINT('Ctrl Pts',(4.33081775314232,23.0233190304191,5.67821209556232));
#452667=CARTESIAN_POINT('Ctrl Pts',(4.92035346181854,22.9518359597249,4.55396647939443));
#452668=CARTESIAN_POINT('Ctrl Pts',(6.18457385510162,22.8803528890307,4.44022731365593));
#452669=CARTESIAN_POINT('Ctrl Pts',(6.96547480693525,22.8088698183366,5.44103442081457));
#452670=CARTESIAN_POINT('Ctrl Pts',(6.5471011960715,22.7373867476423,6.63978858397884));
#452671=CARTESIAN_POINT('Ctrl Pts',(5.31375101838666,22.6659036769482,6.93756666268008));
#452672=CARTESIAN_POINT('Ctrl Pts',(4.39345456041576,22.594420606254,6.06281502530401));
#452673=CARTESIAN_POINT('Ctrl Pts',(4.63327178349907,22.5229375355598,4.81438317658877));
#452674=CARTESIAN_POINT('Ctrl Pts',(5.41441506110672,22.475282155097,4.49968717359432));
#452675=CARTESIAN_POINT('Ctrl Pts',(5.78519550592941,22.4514544648656,4.54238608881333));
#452676=CARTESIAN_POINT('Ctrl Pts',(5.13891927882859,26.1456366054031,4.75759373111246));
#452677=CARTESIAN_POINT('Ctrl Pts',(5.43810071821374,26.1218089151717,4.58527827879321));
#452678=CARTESIAN_POINT('Ctrl Pts',(6.21688915400102,26.0741535347089,4.5658640060888));
#452679=CARTESIAN_POINT('Ctrl Pts',(6.87864168992013,26.0026704640147,5.53797444142439));
#452680=CARTESIAN_POINT('Ctrl Pts',(6.41815729896025,25.9311873933205,6.61847524998255));
#452681=CARTESIAN_POINT('Ctrl Pts',(5.26158350250274,25.8597043226264,6.81819229031504));
#452682=CARTESIAN_POINT('Ctrl Pts',(4.46643823922045,25.7882212519322,5.95378694567247));
#452683=CARTESIAN_POINT('Ctrl Pts',(4.76229843408439,25.716738181238,4.81739664217988));
#452684=CARTESIAN_POINT('Ctrl Pts',(5.87755291922296,25.6452551105439,4.45007439859106));
#452685=CARTESIAN_POINT('Ctrl Pts',(6.79070035947327,25.5737720398496,5.18840274984287));
#452686=CARTESIAN_POINT('Ctrl Pts',(6.66498514592993,25.5022889691555,6.35591148837983));
#452687=CARTESIAN_POINT('Ctrl Pts',(5.61565848936591,25.4308058984613,6.88295739545434));
#452688=CARTESIAN_POINT('Ctrl Pts',(4.60406196791575,25.3593228277671,6.28666204489054));
#452689=CARTESIAN_POINT('Ctrl Pts',(4.55702527594187,25.2878397570729,5.11334619850669));
#452690=CARTESIAN_POINT('Ctrl Pts',(5.5176331484769,25.2163566863788,4.43798405643501));
#452691=CARTESIAN_POINT('Ctrl Pts',(6.60579479560105,25.1448736156845,4.87933393703958));
#452692=CARTESIAN_POINT('Ctrl Pts',(6.82454899803954,25.0733905449905,6.03303673742345));
#452693=CARTESIAN_POINT('Ctrl Pts',(5.97347744575396,25.0019074742962,6.84208605608161));
#452694=CARTESIAN_POINT('Ctrl Pts',(4.83231952202542,24.9304244036021,6.56524194061872));
#452695=CARTESIAN_POINT('Ctrl Pts',(4.44658873189995,24.8589413329078,5.45614521253248));
#452696=CARTESIAN_POINT('Ctrl Pts',(5.16968614336583,24.7874582622137,4.53093499038958));
#452697=CARTESIAN_POINT('Ctrl Pts',(6.33911995340987,24.7159751915195,4.63727615158269));
#452698=CARTESIAN_POINT('Ctrl Pts',(6.88347096747714,24.6444921208254,5.67774038144014));
#452699=CARTESIAN_POINT('Ctrl Pts',(6.30401230613993,24.5730090501312,6.69906868632339));
#452700=CARTESIAN_POINT('Ctrl Pts',(5.13163600271121,24.501525979437,6.76553413784902));
#452701=CARTESIAN_POINT('Ctrl Pts',(4.44045708553489,24.4300429087428,5.8162420056622));
#452702=CARTESIAN_POINT('Ctrl Pts',(4.86372415598115,24.3585598380486,4.72092066657002));
#452703=CARTESIAN_POINT('Ctrl Pts',(6.01364575549064,24.2870767673545,4.48308844595715));
#452704=CARTESIAN_POINT('Ctrl Pts',(6.83667955068161,24.2155936966602,5.32064394905434));
#452705=CARTESIAN_POINT('Ctrl Pts',(6.57877331548261,24.1441106259661,6.46623035855224));
#452706=CARTESIAN_POINT('Ctrl Pts',(5.4762171877825,24.0726275552719,6.87027718549015));
#452707=CARTESIAN_POINT('Ctrl Pts',(4.53915791168179,24.0011444845778,6.16260228864268));
#452708=CARTESIAN_POINT('Ctrl Pts',(4.62611628030965,23.9296614138835,4.99156766820889));
#452709=CARTESIAN_POINT('Ctrl Pts',(5.65742225312448,23.8581783431894,4.43005910275823));
#452710=CARTESIAN_POINT('Ctrl Pts',(6.68820746419386,23.7866952724952,4.99252303072782));
#452711=CARTESIAN_POINT('Ctrl Pts',(6.77408077335862,23.715212201801,6.16363770038041));
#452712=CARTESIAN_POINT('Ctrl Pts',(5.83636609328008,23.6437291311068,6.87044407409259));
#452713=CARTESIAN_POINT('Ctrl Pts',(4.73418498174874,23.5722460604127,6.46537570391973));
#452714=CARTESIAN_POINT('Ctrl Pts',(4.47734003862102,23.5007629897185,5.31955101057097));
#452715=CARTESIAN_POINT('Ctrl Pts',(5.30115015081045,23.4292799190243,4.48275809327536));
#452716=CARTESIAN_POINT('Ctrl Pts',(6.4508497069919,23.3577968483301,4.72165647802514));
#452717=CARTESIAN_POINT('Ctrl Pts',(6.87310399053069,23.286313777636,5.81736804855842));
#452718=CARTESIAN_POINT('Ctrl Pts',(6.18104124059857,23.2148307069418,6.76602226241636));
#452719=CARTESIAN_POINT('Ctrl Pts',(5.00873590166638,23.1433476362476,6.69846478576952));
#452720=CARTESIAN_POINT('Ctrl Pts',(4.43020643614535,23.0718645655534,5.67661126055156));
#452721=CARTESIAN_POINT('Ctrl Pts',(4.97555543184771,23.0003814948593,4.63662978245478));
#452722=CARTESIAN_POINT('Ctrl Pts',(6.1450203373264,22.9288984241651,4.5314155623581));
#452723=CARTESIAN_POINT('Ctrl Pts',(6.86739142284002,22.8574153534709,5.4572104595091));
#452724=CARTESIAN_POINT('Ctrl Pts',(6.48037563201499,22.7859322827767,6.56611594115258));
#452725=CARTESIAN_POINT('Ctrl Pts',(5.33946716650399,22.7144492120825,6.8415750418855));
#452726=CARTESIAN_POINT('Ctrl Pts',(4.48814850723257,22.6429661413884,6.03238754075311));
#452727=CARTESIAN_POINT('Ctrl Pts',(4.70999101793355,22.5714830706942,4.87752780133467));
#452728=CARTESIAN_POINT('Ctrl Pts',(5.4325862664886,22.5238276902314,4.58641880376449));
#452729=CARTESIAN_POINT('Ctrl Pts',(5.7755760807344,22.5,4.62591736201901));
#452730=CARTESIAN_POINT('Ctrl Pts',(5.7755760807344,22.5,4.62591736201901));
#452731=CARTESIAN_POINT('Ctrl Pts',(5.73330573132647,22.5,4.61585820529768));
#452732=CARTESIAN_POINT('Ctrl Pts',(5.69054013141041,22.5,4.60871311258362));
#452733=CARTESIAN_POINT('Ctrl Pts',(5.64753211382414,22.5,4.60431335211636));
#452734=CARTESIAN_POINT('Ctrl Pts',(5.60255613397391,22.5,4.59971226726691));
#452735=CARTESIAN_POINT('Ctrl Pts',(5.557314290973,22.5,4.59811321835507));
#452736=CARTESIAN_POINT('Ctrl Pts',(5.51206909394922,22.5,4.59937363334921));
#452737=CARTESIAN_POINT('Ctrl Pts',(5.47721670522078,22.5,4.60034453139419));
#452738=CARTESIAN_POINT('Ctrl Pts',(5.4423616330716,22.5,4.60301317840862));
#452739=CARTESIAN_POINT('Ctrl Pts',(5.40761856297735,22.5,4.60733474482711));
#452740=CARTESIAN_POINT('Ctrl Pts',(5.39607992713772,22.5,4.60876999453373));
#452741=CARTESIAN_POINT('Ctrl Pts',(5.38455362913149,22.5,4.61038770271512));
#452742=CARTESIAN_POINT('Ctrl Pts',(5.37304385113196,22.5,4.61218665032394));
#452743=CARTESIAN_POINT('Ctrl Pts',(5.36511930671851,22.5,4.6134252354838));
#452744=CARTESIAN_POINT('Ctrl Pts',(5.35720517151447,22.5,4.61474939979765));
#452745=CARTESIAN_POINT('Ctrl Pts',(5.34931138805236,22.5,4.61615691477762));
#452746=CARTESIAN_POINT('Ctrl Pts',(5.30303453466167,22.5,4.62440839072526));
#452747=CARTESIAN_POINT('Ctrl Pts',(5.25737359700834,22.5,4.63553334197763));
#452748=CARTESIAN_POINT('Ctrl Pts',(5.2126037699498,22.5,4.64937620694302));
#452749=CARTESIAN_POINT('Ctrl Pts',(5.16694476107272,22.5,4.66349400761069));
#452750=CARTESIAN_POINT('Ctrl Pts',(5.12221145352414,22.5,4.6804387537632));
#452751=CARTESIAN_POINT('Ctrl Pts',(5.07868894732045,22.5,4.70009847065797));
#452752=CARTESIAN_POINT('Ctrl Pts',(5.04899062899618,22.5,4.71351361104013));
#452753=CARTESIAN_POINT('Ctrl Pts',(5.01985594352847,22.5,4.72819401930014));
#452754=CARTESIAN_POINT('Ctrl Pts',(4.99137807844692,22.5,4.74411779584756));
#452755=CARTESIAN_POINT('Ctrl Pts',(4.98326707951891,22.5,4.74865316864099));
#452756=CARTESIAN_POINT('Ctrl Pts',(4.97520938781291,22.5,4.75328947204393));
#452757=CARTESIAN_POINT('Ctrl Pts',(4.96720722656343,22.5,4.75802635928808));
#452758=CARTESIAN_POINT('Ctrl Pts',(4.95959010108946,22.5,4.76253532422516));
#452759=CARTESIAN_POINT('Ctrl Pts',(4.95203124878916,22.5,4.76713073184038));
#452760=CARTESIAN_POINT('Ctrl Pts',(4.94453365155277,22.5,4.77181088041349));
#452761=CARTESIAN_POINT('Ctrl Pts',(4.90274986858405,22.5,4.79789314464756));
#452762=CARTESIAN_POINT('Ctrl Pts',(4.86285502868317,22.5,4.826610852241));
#452763=CARTESIAN_POINT('Ctrl Pts',(4.82514337767408,22.5,4.85783224447811));
#452764=CARTESIAN_POINT('Ctrl Pts',(4.80185182418205,22.5,4.87711526996037));
#452765=CARTESIAN_POINT('Ctrl Pts',(4.77939307000758,22.5,4.89735438402041));
#452766=CARTESIAN_POINT('Ctrl Pts',(4.75783901282981,22.5,4.9185281570127));
#452767=CARTESIAN_POINT('Ctrl Pts',(4.72385034361533,22.5,4.95191715474625));
#452768=CARTESIAN_POINT('Ctrl Pts',(4.69210932076019,22.5,4.98762826934671));
#452769=CARTESIAN_POINT('Ctrl Pts',(4.66265412509277,22.5,5.02537769858569));
#452770=CARTESIAN_POINT('Ctrl Pts',(4.65606489345436,22.5,5.03382237966274));
#452771=CARTESIAN_POINT('Ctrl Pts',(4.64959018437146,22.5,5.04236922201164));
#452772=CARTESIAN_POINT('Ctrl Pts',(4.64323066284989,22.5,5.05101530317395));
#452773=CARTESIAN_POINT('Ctrl Pts',(4.63787530249446,22.5,5.05829617802112));
#452774=CARTESIAN_POINT('Ctrl Pts',(4.63260299860475,22.5,5.06564571345099));
#452775=CARTESIAN_POINT('Ctrl Pts',(4.62742036981385,22.5,5.07305265320345));
#452776=CARTESIAN_POINT('Ctrl Pts',(4.59922209460147,22.5,5.11335322923306));
#452777=CARTESIAN_POINT('Ctrl Pts',(4.57362076198805,22.5,5.15542403883563));
#452778=CARTESIAN_POINT('Ctrl Pts',(4.55062598367203,22.5,5.19892882008167));
#452779=CARTESIAN_POINT('Ctrl Pts',(4.52705592798244,22.5,5.24352199261156));
#452780=CARTESIAN_POINT('Ctrl Pts',(4.50622389130747,22.5,5.28962259945306));
#452781=CARTESIAN_POINT('Ctrl Pts',(4.48817542916681,22.5,5.33691174796499));
#452782=CARTESIAN_POINT('Ctrl Pts',(4.47740085898595,22.5,5.36514242188412));
#452783=CARTESIAN_POINT('Ctrl Pts',(4.46761902478338,22.5,5.39379744240128));
#452784=CARTESIAN_POINT('Ctrl Pts',(4.45884671158303,22.5,5.42281409035157));
#452785=CARTESIAN_POINT('Ctrl Pts',(4.45401588346689,22.5,5.43879327800172));
#452786=CARTESIAN_POINT('Ctrl Pts',(4.44949130096016,22.5,5.4548821890281));
#452787=CARTESIAN_POINT('Ctrl Pts',(4.4452765301246,22.5,5.47107067779953));
#452788=CARTESIAN_POINT('Ctrl Pts',(4.44297713124816,22.5,5.47990242556109));
#452789=CARTESIAN_POINT('Ctrl Pts',(4.44077047507025,22.5,5.48876206567358));
#452790=CARTESIAN_POINT('Ctrl Pts',(4.4386590540276,22.5,5.49763888067812));
#452791=CARTESIAN_POINT('Ctrl Pts',(4.42647927127823,22.5,5.54884500019556));
#452792=CARTESIAN_POINT('Ctrl Pts',(4.41744307914003,22.5,5.60070295226456));
#452793=CARTESIAN_POINT('Ctrl Pts',(4.411605943275,22.5,5.6528725699024));
#452794=CARTESIAN_POINT('Ctrl Pts',(4.4076292437891,22.5,5.68841446860706));
#452795=CARTESIAN_POINT('Ctrl Pts',(4.40513819218715,22.5,5.72410179499005));
#452796=CARTESIAN_POINT('Ctrl Pts',(4.40416293207702,22.5,5.75983273054518));
#452797=CARTESIAN_POINT('Ctrl Pts',(4.40371155802895,22.5,5.77636987469309));
#452798=CARTESIAN_POINT('Ctrl Pts',(4.4035852965956,22.5,5.79292145716924));
#452799=CARTESIAN_POINT('Ctrl Pts',(4.40378695835843,22.5,5.80944675439426));
#452800=CARTESIAN_POINT('Ctrl Pts',(4.40443526815155,22.5,5.86257289925538));
#452801=CARTESIAN_POINT('Ctrl Pts',(4.40846556103476,22.5,5.91547919598232));
#452802=CARTESIAN_POINT('Ctrl Pts',(4.41595519071752,22.5,5.96783294656611));
#452803=CARTESIAN_POINT('Ctrl Pts',(4.41992831406983,22.5,5.99560573612131));
#452804=CARTESIAN_POINT('Ctrl Pts',(4.42487575252187,22.5,6.023223319992));
#452805=CARTESIAN_POINT('Ctrl Pts',(4.43081497898236,22.5,6.05063695240159));
#452806=CARTESIAN_POINT('Ctrl Pts',(4.43420326443596,22.5,6.06627623009907));
#452807=CARTESIAN_POINT('Ctrl Pts',(4.43791441703144,22.5,6.0818491333573));
#452808=CARTESIAN_POINT('Ctrl Pts',(4.44194158662795,22.5,6.09735008669016));
#452809=CARTESIAN_POINT('Ctrl Pts',(6.39006796800885,25.6019615242271,4.92443355077908));
#452810=CARTESIAN_POINT('Ctrl Pts',(6.48712194011206,25.5925650294346,5.02053320993752));
#452811=CARTESIAN_POINT('Ctrl Pts',(6.56580235206401,25.5831685346421,5.13467106978717));
#452812=CARTESIAN_POINT('Ctrl Pts',(6.617556583841,25.5737720398497,5.25993281439039));
#452813=CARTESIAN_POINT('Ctrl Pts',(6.74879528829216,25.5499443496183,5.57757232935519));
#452814=CARTESIAN_POINT('Ctrl Pts',(6.70689021711104,25.5261166593869,5.96674190886751));
#452815=CARTESIAN_POINT('Ctrl Pts',(6.51104990542648,25.5022889691555,6.24916768313609));
#452816=CARTESIAN_POINT('Ctrl Pts',(6.31520959374192,25.4784612789241,6.53159345740467));
#452817=CARTESIAN_POINT('Ctrl Pts',(5.96543404155392,25.4546335886927,6.7072754264295));
#452818=CARTESIAN_POINT('Ctrl Pts',(5.62194684521822,25.4308058984613,6.69573385251462));
#452819=CARTESIAN_POINT('Ctrl Pts',(5.27845964888252,25.4069782082299,6.68419227859974));
#452820=CARTESIAN_POINT('Ctrl Pts',(4.94126080839914,25.3831505179985,6.48542716174514));
#452821=CARTESIAN_POINT('Ctrl Pts',(4.76482193949513,25.3593228277671,6.19049196225386));
#452822=CARTESIAN_POINT('Ctrl Pts',(4.58838307059113,25.3354951375357,5.89555676276259));
#452823=CARTESIAN_POINT('Ctrl Pts',(4.57270417326649,25.3116674473043,5.50445148063464));
#452824=CARTESIAN_POINT('Ctrl Pts',(4.72496603669335,25.2878397570729,5.19633848255872));
#452825=CARTESIAN_POINT('Ctrl Pts',(4.87722790012021,25.2640120668416,4.8882254844828));
#452826=CARTESIAN_POINT('Ctrl Pts',(5.19743052429855,25.2401843766102,4.66310477045891));
#452827=CARTESIAN_POINT('Ctrl Pts',(5.53889211090842,25.2163566863788,4.62410272688105));
#452828=CARTESIAN_POINT('Ctrl Pts',(5.84649605160076,25.1948916323282,4.58896793348097));
#452829=CARTESIAN_POINT('Ctrl Pts',(6.17135209942283,25.1734265782776,4.70487246063661));
#452830=CARTESIAN_POINT('Ctrl Pts',(6.39198798715975,25.151961524227,4.92254817630007));
#452831=CARTESIAN_POINT('Origin',(3.50148276475995,22.5,-3.50148276475995));
#452832=CARTESIAN_POINT('',(7.42462120245875,22.5,7.42462120245875));
#452833=CARTESIAN_POINT('Origin',(0.,22.5,0.));
#452834=CARTESIAN_POINT('Ctrl Pts',(6.64591806159944,22.5,-4.8286920333622));
#452835=CARTESIAN_POINT('Ctrl Pts',(6.6755807993511,22.5,-4.8719367804586));
#452836=CARTESIAN_POINT('Ctrl Pts',(6.70227440867208,22.5,-4.91697381282205));
#452837=CARTESIAN_POINT('Ctrl Pts',(6.72600910610864,22.5,-4.96347942286289));
#452838=CARTESIAN_POINT('Ctrl Pts',(6.75002004749321,22.5,-5.01052630347844));
#452839=CARTESIAN_POINT('Ctrl Pts',(6.77100289981689,22.5,-5.05907736675537));
#452840=CARTESIAN_POINT('Ctrl Pts',(6.78891649180145,22.5,-5.10881343934184));
#452841=CARTESIAN_POINT('Ctrl Pts',(6.8018723011903,22.5,-5.14478450961828));
#452842=CARTESIAN_POINT('Ctrl Pts',(6.81322157811577,22.5,-5.18137581815984));
#452843=CARTESIAN_POINT('Ctrl Pts',(6.82293175279821,22.5,-5.21846626007171));
#452844=CARTESIAN_POINT('Ctrl Pts',(6.82709087591144,22.5,-5.23435307151234));
#452845=CARTESIAN_POINT('Ctrl Pts',(6.83094910537903,22.5,-5.25033142516077));
#452846=CARTESIAN_POINT('Ctrl Pts',(6.83450307899155,22.5,-5.26639159476287));
#452847=CARTESIAN_POINT('Ctrl Pts',(6.83669994897119,22.5,-5.27631910360604));
#452848=CARTESIAN_POINT('Ctrl Pts',(6.83878067256692,22.5,-5.28627904839608));
#452849=CARTESIAN_POINT('Ctrl Pts',(6.84074133407639,22.5,-5.29625198816685));
#452850=CARTESIAN_POINT('Ctrl Pts',(6.85068531168518,22.5,-5.34683220779938));
#452851=CARTESIAN_POINT('Ctrl Pts',(6.85756855485384,22.5,-5.39784710632373));
#452852=CARTESIAN_POINT('Ctrl Pts',(6.86136063350185,22.5,-5.44899668917511));
#452853=CARTESIAN_POINT('Ctrl Pts',(6.86506621321198,22.5,-5.49897952813742));
#452854=CARTESIAN_POINT('Ctrl Pts',(6.86581982211528,22.5,-5.54909202981808));
#452855=CARTESIAN_POINT('Ctrl Pts',(6.86354521213908,22.5,-5.59904614070299));
#452856=CARTESIAN_POINT('Ctrl Pts',(6.86196264981798,22.5,-5.63380176672122));
#452857=CARTESIAN_POINT('Ctrl Pts',(6.85891323510394,22.5,-5.66848055905629));
#452858=CARTESIAN_POINT('Ctrl Pts',(6.85435789422027,22.5,-5.7029791597992));
#452859=CARTESIAN_POINT('Ctrl Pts',(6.85274935352435,22.5,-5.71516099309431));
#452860=CARTESIAN_POINT('Ctrl Pts',(6.85095294331449,22.5,-5.72732029664114));
#452861=CARTESIAN_POINT('Ctrl Pts',(6.84896661755834,22.5,-5.73945229542231));
#452862=CARTESIAN_POINT('Ctrl Pts',(6.8474996850627,22.5,-5.74841196540296));
#452863=CARTESIAN_POINT('Ctrl Pts',(6.84592925278567,22.5,-5.75735562847588));
#452864=CARTESIAN_POINT('Ctrl Pts',(6.84425707988428,22.5,-5.7662692101314));
#452865=CARTESIAN_POINT('Ctrl Pts',(6.83533972756861,22.5,-5.81380349797354));
#452866=CARTESIAN_POINT('Ctrl Pts',(6.82351786766256,22.5,-5.86057802541052));
#452867=CARTESIAN_POINT('Ctrl Pts',(6.80873145081366,22.5,-5.90632961629785));
#452868=CARTESIAN_POINT('Ctrl Pts',(6.79814742517805,22.5,-5.93907832180037));
#452869=CARTESIAN_POINT('Ctrl Pts',(6.78604349567089,22.5,-5.97130269602399));
#452870=CARTESIAN_POINT('Ctrl Pts',(6.77238316128915,22.5,-6.00289829431615));
#452871=CARTESIAN_POINT('Ctrl Pts',(6.75417864027363,22.5,-6.0450043450931));
#452872=CARTESIAN_POINT('Ctrl Pts',(6.73321019789003,22.5,-6.08599501913005));
#452873=CARTESIAN_POINT('Ctrl Pts',(6.70966855565445,22.5,-6.12568011956913));
#452874=CARTESIAN_POINT('Ctrl Pts',(6.70346098498274,22.5,-6.13614447303795));
#452875=CARTESIAN_POINT('Ctrl Pts',(6.69707438313402,22.5,-6.1465178772431));
#452876=CARTESIAN_POINT('Ctrl Pts',(6.690512023297,22.5,-6.15679645323974));
#452877=CARTESIAN_POINT('Ctrl Pts',(6.68556313817567,22.5,-6.16454785564401));
#452878=CARTESIAN_POINT('Ctrl Pts',(6.68051415735856,22.5,-6.17224531916678));
#452879=CARTESIAN_POINT('Ctrl Pts',(6.67537489362519,22.5,-6.17987521962693));
#452880=CARTESIAN_POINT('Ctrl Pts',(6.6484247679217,22.5,-6.21988616033247));
#452881=CARTESIAN_POINT('Ctrl Pts',(6.61894162109436,22.5,-6.25812741400869));
#452882=CARTESIAN_POINT('Ctrl Pts',(6.58718324847867,22.5,-6.29441170519143));
#452883=CARTESIAN_POINT('Ctrl Pts',(6.55551163430383,22.5,-6.33059687389808));
#452884=CARTESIAN_POINT('Ctrl Pts',(6.52157609264422,22.5,-6.36483641853547));
#452885=CARTESIAN_POINT('Ctrl Pts',(6.48560329452573,22.5,-6.39690234768395));
#452886=CARTESIAN_POINT('Ctrl Pts',(6.46634118603625,22.5,-6.41407247173267));
#452887=CARTESIAN_POINT('Ctrl Pts',(6.44649455979684,22.5,-6.4306185943358));
#452888=CARTESIAN_POINT('Ctrl Pts',(6.42609644694928,22.5,-6.44649972129179));
#452889=CARTESIAN_POINT('Ctrl Pts',(6.41550137782644,22.5,-6.45474860387739));
#452890=CARTESIAN_POINT('Ctrl Pts',(6.40475750959663,22.5,-6.46281800341801));
#452891=CARTESIAN_POINT('Ctrl Pts',(6.3938694226933,22.5,-6.47070167900491));
#452892=CARTESIAN_POINT('Ctrl Pts',(6.3855291898448,22.5,-6.47674054429691));
#452893=CARTESIAN_POINT('Ctrl Pts',(6.37710396966129,22.5,-6.48267052699799));
#452894=CARTESIAN_POINT('Ctrl Pts',(6.36860849913158,22.5,-6.48848046707363));
#452895=CARTESIAN_POINT('Ctrl Pts',(6.33038178349398,22.5,-6.51462321294818));
#452896=CARTESIAN_POINT('Ctrl Pts',(6.29067294978169,22.5,-6.53838419609424));
#452897=CARTESIAN_POINT('Ctrl Pts',(6.24968947052795,22.5,-6.55954587135352));
#452898=CARTESIAN_POINT('Ctrl Pts',(6.2220434631434,22.5,-6.57382078995829));
#452899=CARTESIAN_POINT('Ctrl Pts',(6.1938170783215,22.5,-6.58691199092427));
#452900=CARTESIAN_POINT('Ctrl Pts',(6.16507259987822,22.5,-6.59873928463863));
#452901=CARTESIAN_POINT('Ctrl Pts',(6.15266397552728,22.5,-6.60384497633101));
#452902=CARTESIAN_POINT('Ctrl Pts',(6.14015674557275,22.5,-6.60871552223012));
#452903=CARTESIAN_POINT('Ctrl Pts',(6.12757735909169,22.5,-6.61333659562422));
#452904=CARTESIAN_POINT('Ctrl Pts',(6.08619113933328,22.5,-6.6285399411368));
#452905=CARTESIAN_POINT('Ctrl Pts',(6.04397428611167,22.5,-6.64106838660522));
#452906=CARTESIAN_POINT('Ctrl Pts',(6.00111091241908,22.5,-6.65070263631015));
#452907=CARTESIAN_POINT('Ctrl Pts',(5.97991194550769,22.5,-6.6554674535216));
#452908=CARTESIAN_POINT('Ctrl Pts',(5.95855482028607,22.5,-6.65952358177559));
#452909=CARTESIAN_POINT('Ctrl Pts',(5.93706218561481,22.5,-6.66283972884874));
#452910=CARTESIAN_POINT('Ctrl Pts',(5.92425778841234,22.5,-6.66481534816932));
#452911=CARTESIAN_POINT('Ctrl Pts',(5.91140530098883,22.5,-6.66652825557881));
#452912=CARTESIAN_POINT('Ctrl Pts',(5.89851203167795,22.5,-6.66798006829994));
#452913=CARTESIAN_POINT('Ctrl Pts',(4.62591736201901,22.5,-5.7755760807344));
#452914=CARTESIAN_POINT('Ctrl Pts',(4.61585820529768,22.5,-5.73330573132648));
#452915=CARTESIAN_POINT('Ctrl Pts',(4.60871311258362,22.5,-5.69054013141041));
#452916=CARTESIAN_POINT('Ctrl Pts',(4.60431335211636,22.5,-5.64753211382415));
#452917=CARTESIAN_POINT('Ctrl Pts',(4.59971226726699,22.5,-5.60255613397477));
#452918=CARTESIAN_POINT('Ctrl Pts',(4.59811321835513,22.5,-5.5573142909747));
#452919=CARTESIAN_POINT('Ctrl Pts',(4.59937363334914,22.5,-5.51206909395177));
#452920=CARTESIAN_POINT('Ctrl Pts',(4.60034453139403,22.5,-5.47721670522323));
#452921=CARTESIAN_POINT('Ctrl Pts',(4.6030131784084,22.5,-5.4423616330739));
#452922=CARTESIAN_POINT('Ctrl Pts',(4.60733474482684,22.5,-5.40761856297955));
#452923=CARTESIAN_POINT('Ctrl Pts',(4.6087699944925,22.5,-5.39607992746903));
#452924=CARTESIAN_POINT('Ctrl Pts',(4.61038770262252,22.5,-5.38455362979122));
#452925=CARTESIAN_POINT('Ctrl Pts',(4.61218665016966,22.5,-5.37304385211902));
#452926=CARTESIAN_POINT('Ctrl Pts',(4.61342523528797,22.5,-5.36511930792512));
#452927=CARTESIAN_POINT('Ctrl Pts',(4.61474939955571,22.5,-5.35720517293886));
#452928=CARTESIAN_POINT('Ctrl Pts',(4.61615691448497,22.5,-5.3493113896936));
#452929=CARTESIAN_POINT('Ctrl Pts',(4.62440839035928,22.5,-5.30303453631806));
#452930=CARTESIAN_POINT('Ctrl Pts',(4.63553334153678,22.5,-5.25737359867573));
#452931=CARTESIAN_POINT('Ctrl Pts',(4.64937620642544,22.5,-5.21260377162372));
#452932=CARTESIAN_POINT('Ctrl Pts',(4.66349400702439,22.5,-5.16694476272245));
#452933=CARTESIAN_POINT('Ctrl Pts',(4.68043875311008,22.5,-5.12221145514625));
#452934=CARTESIAN_POINT('Ctrl Pts',(4.70009846993925,22.5,-5.07868894891155));
#452935=CARTESIAN_POINT('Ctrl Pts',(4.71351361033608,22.5,-5.04899063043454));
#452936=CARTESIAN_POINT('Ctrl Pts',(4.72819401862254,22.5,-5.01985594481751));
#452937=CARTESIAN_POINT('Ctrl Pts',(4.74411779520772,22.5,-4.99137807959121));
#452938=CARTESIAN_POINT('Ctrl Pts',(4.7486531673282,22.5,-4.98326708184471));
#452939=CARTESIAN_POINT('Ctrl Pts',(4.75328947002864,22.5,-4.97520939130455));
#452940=CARTESIAN_POINT('Ctrl Pts',(4.75802635654096,22.5,-4.96720723120421));
#452941=CARTESIAN_POINT('Ctrl Pts',(4.76253532219619,22.5,-4.95959010443409));
#452942=CARTESIAN_POINT('Ctrl Pts',(4.7671307305627,22.5,-4.95203125085003));
#452943=CARTESIAN_POINT('Ctrl Pts',(4.7718108799136,22.5,-4.9445336523536));
#452944=CARTESIAN_POINT('Ctrl Pts',(4.79789314411416,22.5,-4.90274986936038));
#452945=CARTESIAN_POINT('Ctrl Pts',(4.82661085167514,22.5,-4.86285502943318));
#452946=CARTESIAN_POINT('Ctrl Pts',(4.85783224388052,22.5,-4.8251433783959));
#452947=CARTESIAN_POINT('Ctrl Pts',(4.87711526954221,22.5,-4.80185182464605));
#452948=CARTESIAN_POINT('Ctrl Pts',(4.89735438380168,22.5,-4.77939307023024));
#452949=CARTESIAN_POINT('Ctrl Pts',(4.9185281570127,22.5,-4.75783901282981));
#452950=CARTESIAN_POINT('Ctrl Pts',(4.95191715474625,22.5,-4.72385034361532));
#452951=CARTESIAN_POINT('Ctrl Pts',(4.98762826934674,22.5,-4.69210932076016));
#452952=CARTESIAN_POINT('Ctrl Pts',(5.02537769858573,22.5,-4.66265412509274));
#452953=CARTESIAN_POINT('Ctrl Pts',(5.03382237964628,22.5,-4.6560648934672));
#452954=CARTESIAN_POINT('Ctrl Pts',(5.04236922197827,22.5,-4.64959018439674));
#452955=CARTESIAN_POINT('Ctrl Pts',(5.0510153031233,22.5,-4.64323066288715));
#452956=CARTESIAN_POINT('Ctrl Pts',(5.05829617800763,22.5,-4.63787530250376));
#452957=CARTESIAN_POINT('Ctrl Pts',(5.06564571347538,22.5,-4.63260299858695));
#452958=CARTESIAN_POINT('Ctrl Pts',(5.07305265326631,22.5,-4.62742036976986));
#452959=CARTESIAN_POINT('Ctrl Pts',(5.1133532292971,22.5,-4.59922209456066));
#452960=CARTESIAN_POINT('Ctrl Pts',(5.15542403890062,22.5,-4.57362076195032));
#452961=CARTESIAN_POINT('Ctrl Pts',(5.19892882014737,22.5,-4.55062598363731));
#452962=CARTESIAN_POINT('Ctrl Pts',(5.24352199267827,22.5,-4.52705592795066));
#452963=CARTESIAN_POINT('Ctrl Pts',(5.28962259952057,22.5,-4.50622389127859));
#452964=CARTESIAN_POINT('Ctrl Pts',(5.33691174803316,22.5,-4.48817542914079));
#452965=CARTESIAN_POINT('Ctrl Pts',(5.36514242195013,22.5,-4.47740085896262));
#452966=CARTESIAN_POINT('Ctrl Pts',(5.39379744246496,22.5,-4.46761902476255));
#452967=CARTESIAN_POINT('Ctrl Pts',(5.42281409041283,22.5,-4.45884671156451));
#452968=CARTESIAN_POINT('Ctrl Pts',(5.4387932780761,22.5,-4.45401588344527));
#452969=CARTESIAN_POINT('Ctrl Pts',(5.4548821891158,22.5,-4.44949130093593));
#452970=CARTESIAN_POINT('Ctrl Pts',(5.47107067790065,22.5,-4.44527653009828));
#452971=CARTESIAN_POINT('Ctrl Pts',(5.47990242565713,22.5,-4.44297713122391));
#452972=CARTESIAN_POINT('Ctrl Pts',(5.48876206576444,22.5,-4.440770475048));
#452973=CARTESIAN_POINT('Ctrl Pts',(5.49763888076378,22.5,-4.43865905400722));
#452974=CARTESIAN_POINT('Ctrl Pts',(5.54884500028241,22.5,-4.42647927126125));
#452975=CARTESIAN_POINT('Ctrl Pts',(5.60070295235243,22.5,-4.41744307912653));
#452976=CARTESIAN_POINT('Ctrl Pts',(5.6528725699911,22.5,-4.41160594326508));
#452977=CARTESIAN_POINT('Ctrl Pts',(5.68841446871037,22.5,-4.40762924378005));
#452978=CARTESIAN_POINT('Ctrl Pts',(5.72410179510797,22.5,-4.40513819218018));
#452979=CARTESIAN_POINT('Ctrl Pts',(5.75983273067766,22.5,-4.4041629320734));
#452980=CARTESIAN_POINT('Ctrl Pts',(5.77636987481073,22.5,-4.40371155802747));
#452981=CARTESIAN_POINT('Ctrl Pts',(5.79292145727197,22.5,-4.4035852965957));
#452982=CARTESIAN_POINT('Ctrl Pts',(5.80944675448204,22.5,-4.40378695835951));
#452983=CARTESIAN_POINT('Ctrl Pts',(5.86257289934304,22.5,-4.40443526815635));
#452984=CARTESIAN_POINT('Ctrl Pts',(5.91547919606967,22.5,-4.40846556104334));
#452985=CARTESIAN_POINT('Ctrl Pts',(5.96783294665298,22.5,-4.41595519072995));
#452986=CARTESIAN_POINT('Ctrl Pts',(5.99560573617887,22.5,-4.41992831408015));
#452987=CARTESIAN_POINT('Ctrl Pts',(6.02322332002059,22.5,-4.42487575252807));
#452988=CARTESIAN_POINT('Ctrl Pts',(6.05063695240159,22.5,-4.43081497898236));
#452989=CARTESIAN_POINT('Ctrl Pts',(6.06627623009907,22.5,-4.43420326443596));
#452990=CARTESIAN_POINT('Ctrl Pts',(6.0818491333573,22.5,-4.43791441703144));
#452991=CARTESIAN_POINT('Ctrl Pts',(6.09735008669015,22.5,-4.44194158662795));
#452992=CARTESIAN_POINT('Ctrl Pts',(-4.8286920333622,22.5,-6.64591806159944));
#452993=CARTESIAN_POINT('Ctrl Pts',(-4.8719367804586,22.5,-6.6755807993511));
#452994=CARTESIAN_POINT('Ctrl Pts',(-4.91697381282206,22.5,-6.70227440867209));
#452995=CARTESIAN_POINT('Ctrl Pts',(-4.9634794228629,22.5,-6.72600910610865));
#452996=CARTESIAN_POINT('Ctrl Pts',(-5.01052630347777,22.5,-6.75002004749286));
#452997=CARTESIAN_POINT('Ctrl Pts',(-5.05907736675395,22.5,-6.77100289981628));
#452998=CARTESIAN_POINT('Ctrl Pts',(-5.10881343933966,22.5,-6.78891649180067));
#452999=CARTESIAN_POINT('Ctrl Pts',(-5.14478450961618,22.5,-6.80187230118961));
#453000=CARTESIAN_POINT('Ctrl Pts',(-5.18137581815778,22.5,-6.81322157811517));
#453001=CARTESIAN_POINT('Ctrl Pts',(-5.21846626006973,22.5,-6.82293175279769));
#453002=CARTESIAN_POINT('Ctrl Pts',(-5.23435307150809,22.5,-6.82709087591036));
#453003=CARTESIAN_POINT('Ctrl Pts',(-5.25033142515424,22.5,-6.83094910537747));
#453004=CARTESIAN_POINT('Ctrl Pts',(-5.26639159475403,22.5,-6.8345030789896));
#453005=CARTESIAN_POINT('Ctrl Pts',(-5.27631910353288,22.5,-6.83669994895507));
#453006=CARTESIAN_POINT('Ctrl Pts',(-5.28627904825824,22.5,-6.83878067253816));
#453007=CARTESIAN_POINT('Ctrl Pts',(-5.29625198796418,22.5,-6.84074133403655));
#453008=CARTESIAN_POINT('Ctrl Pts',(-5.34683220759866,22.5,-6.85068531165414));
#453009=CARTESIAN_POINT('Ctrl Pts',(-5.39784710612543,22.5,-6.85756855483123));
#453010=CARTESIAN_POINT('Ctrl Pts',(-5.44899668897961,22.5,-6.86136063348736));
#453011=CARTESIAN_POINT('Ctrl Pts',(-5.49897952794281,22.5,-6.86506621320529));
#453012=CARTESIAN_POINT('Ctrl Pts',(-5.54909202962473,22.5,-6.86581982211631));
#453013=CARTESIAN_POINT('Ctrl Pts',(-5.59904614051128,22.5,-6.8635452121478));
#453014=CARTESIAN_POINT('Ctrl Pts',(-5.63380176654577,22.5,-6.86196264983138));
#453015=CARTESIAN_POINT('Ctrl Pts',(-5.66848055889722,22.5,-6.85891323512072));
#453016=CARTESIAN_POINT('Ctrl Pts',(-5.70297915965648,22.5,-6.85435789423911));
#453017=CARTESIAN_POINT('Ctrl Pts',(-5.71516099264261,22.5,-6.85274935358548));
#453018=CARTESIAN_POINT('Ctrl Pts',(-5.72732029588166,22.5,-6.85095294342745));
#453019=CARTESIAN_POINT('Ctrl Pts',(-5.73945229435654,22.5,-6.84896661773283));
#453020=CARTESIAN_POINT('Ctrl Pts',(-5.74841196443544,22.5,-6.84749968522951));
#453021=CARTESIAN_POINT('Ctrl Pts',(-5.75735562760714,22.5,-6.84592925294246));
#453022=CARTESIAN_POINT('Ctrl Pts',(-5.76626920936078,22.5,-6.84425708002884));
#453023=CARTESIAN_POINT('Ctrl Pts',(-5.81380349721498,22.5,-6.83533972774389));
#453024=CARTESIAN_POINT('Ctrl Pts',(-5.86057802466526,22.5,-6.82351786786828));
#453025=CARTESIAN_POINT('Ctrl Pts',(-5.9063296155672,22.5,-6.8087314510498));
#453026=CARTESIAN_POINT('Ctrl Pts',(-5.93907832132107,22.5,-6.79814742535809));
#453027=CARTESIAN_POINT('Ctrl Pts',(-5.97130269578902,22.5,-6.78604349577248));
#453028=CARTESIAN_POINT('Ctrl Pts',(-6.00289829431615,22.5,-6.77238316128915));
#453029=CARTESIAN_POINT('Ctrl Pts',(-6.0450043450931,22.5,-6.75417864027363));
#453030=CARTESIAN_POINT('Ctrl Pts',(-6.08599501913005,22.5,-6.73321019789003));
#453031=CARTESIAN_POINT('Ctrl Pts',(-6.12568011956913,22.5,-6.70966855565445));
#453032=CARTESIAN_POINT('Ctrl Pts',(-6.13614447303768,22.5,-6.7034609849829));
#453033=CARTESIAN_POINT('Ctrl Pts',(-6.14651787724254,22.5,-6.69707438313436));
#453034=CARTESIAN_POINT('Ctrl Pts',(-6.15679645323891,22.5,-6.69051202329753));
#453035=CARTESIAN_POINT('Ctrl Pts',(-6.164547855591,22.5,-6.68556313820952));
#453036=CARTESIAN_POINT('Ctrl Pts',(-6.17224531906237,22.5,-6.68051415742705));
#453037=CARTESIAN_POINT('Ctrl Pts',(-6.17987521947202,22.5,-6.67537489372953));
#453038=CARTESIAN_POINT('Ctrl Pts',(-6.21988616018154,22.5,-6.64842476803299));
#453039=CARTESIAN_POINT('Ctrl Pts',(-6.25812741386204,22.5,-6.61894162121229));
#453040=CARTESIAN_POINT('Ctrl Pts',(-6.29441170504936,22.5,-6.58718324860302));
#453041=CARTESIAN_POINT('Ctrl Pts',(-6.33059687376143,22.5,-6.55551163443383));
#453042=CARTESIAN_POINT('Ctrl Pts',(-6.36483641840449,22.5,-6.52157609277951));
#453043=CARTESIAN_POINT('Ctrl Pts',(-6.39690234755893,22.5,-6.48560329466599));
#453044=CARTESIAN_POINT('Ctrl Pts',(-6.41407247161589,22.5,-6.4663411861735));
#453045=CARTESIAN_POINT('Ctrl Pts',(-6.43061859422698,22.5,-6.44649455993064));
#453046=CARTESIAN_POINT('Ctrl Pts',(-6.44649972119062,22.5,-6.42609644707924));
#453047=CARTESIAN_POINT('Ctrl Pts',(-6.4547486037322,22.5,-6.41550137801605));
#453048=CARTESIAN_POINT('Ctrl Pts',(-6.46281800323078,22.5,-6.40475750984752));
#453049=CARTESIAN_POINT('Ctrl Pts',(-6.47070167877777,22.5,-6.39386942300701));
#453050=CARTESIAN_POINT('Ctrl Pts',(-6.47674054409838,22.5,-6.38552919012489));
#453051=CARTESIAN_POINT('Ctrl Pts',(-6.48267052682731,22.5,-6.37710396990682));
#453052=CARTESIAN_POINT('Ctrl Pts',(-6.48848046692978,22.5,-6.36860849934192));
#453053=CARTESIAN_POINT('Ctrl Pts',(-6.51462321281365,22.5,-6.33038178370894));
#453054=CARTESIAN_POINT('Ctrl Pts',(-6.53838419596926,22.5,-6.29067295000084));
#453055=CARTESIAN_POINT('Ctrl Pts',(-6.55954587123842,22.5,-6.24968947075085));
#453056=CARTESIAN_POINT('Ctrl Pts',(-6.5738207898325,22.5,-6.22204346340245));
#453057=CARTESIAN_POINT('Ctrl Pts',(-6.58691199079083,22.5,-6.1938170786179));
#453058=CARTESIAN_POINT('Ctrl Pts',(-6.59873928450088,22.5,-6.16507260021298));
#453059=CARTESIAN_POINT('Ctrl Pts',(-6.60384497623248,22.5,-6.15266397577878));
#453060=CARTESIAN_POINT('Ctrl Pts',(-6.60871552216769,22.5,-6.14015674573947));
#453061=CARTESIAN_POINT('Ctrl Pts',(-6.61333659559451,22.5,-6.12757735917257));
#453062=CARTESIAN_POINT('Ctrl Pts',(-6.62853994111127,22.5,-6.08619113941338));
#453063=CARTESIAN_POINT('Ctrl Pts',(-6.64106838658374,22.5,-6.04397428619079));
#453064=CARTESIAN_POINT('Ctrl Pts',(-6.65070263629263,22.5,-6.00111091249705));
#453065=CARTESIAN_POINT('Ctrl Pts',(-6.65546745351165,22.5,-5.97991194556006));
#453066=CARTESIAN_POINT('Ctrl Pts',(-6.65952358177152,22.5,-5.95855482031242));
#453067=CARTESIAN_POINT('Ctrl Pts',(-6.66283972884874,22.5,-5.93706218561481));
#453068=CARTESIAN_POINT('Ctrl Pts',(-6.66481534816932,22.5,-5.92425778841234));
#453069=CARTESIAN_POINT('Ctrl Pts',(-6.66652825557881,22.5,-5.91140530098883));
#453070=CARTESIAN_POINT('Ctrl Pts',(-6.66798006829994,22.5,-5.89851203167795));
#453071=CARTESIAN_POINT('Ctrl Pts',(-5.7755760807344,22.5,-4.62591736201901));
#453072=CARTESIAN_POINT('Ctrl Pts',(-5.73330573132648,22.5,-4.61585820529768));
#453073=CARTESIAN_POINT('Ctrl Pts',(-5.69054013141041,22.5,-4.60871311258362));
#453074=CARTESIAN_POINT('Ctrl Pts',(-5.64753211382415,22.5,-4.60431335211636));
#453075=CARTESIAN_POINT('Ctrl Pts',(-5.60255613397477,22.5,-4.59971226726699));
#453076=CARTESIAN_POINT('Ctrl Pts',(-5.5573142909747,22.5,-4.59811321835513));
#453077=CARTESIAN_POINT('Ctrl Pts',(-5.51206909395177,22.5,-4.59937363334914));
#453078=CARTESIAN_POINT('Ctrl Pts',(-5.47721670522323,22.5,-4.60034453139403));
#453079=CARTESIAN_POINT('Ctrl Pts',(-5.4423616330739,22.5,-4.6030131784084));
#453080=CARTESIAN_POINT('Ctrl Pts',(-5.40761856297955,22.5,-4.60733474482684));
#453081=CARTESIAN_POINT('Ctrl Pts',(-5.39607992746903,22.5,-4.6087699944925));
#453082=CARTESIAN_POINT('Ctrl Pts',(-5.38455362979122,22.5,-4.61038770262252));
#453083=CARTESIAN_POINT('Ctrl Pts',(-5.37304385211902,22.5,-4.61218665016966));
#453084=CARTESIAN_POINT('Ctrl Pts',(-5.36511930792512,22.5,-4.61342523528797));
#453085=CARTESIAN_POINT('Ctrl Pts',(-5.35720517293886,22.5,-4.61474939955571));
#453086=CARTESIAN_POINT('Ctrl Pts',(-5.3493113896936,22.5,-4.61615691448497));
#453087=CARTESIAN_POINT('Ctrl Pts',(-5.30303453631806,22.5,-4.62440839035928));
#453088=CARTESIAN_POINT('Ctrl Pts',(-5.25737359867573,22.5,-4.63553334153678));
#453089=CARTESIAN_POINT('Ctrl Pts',(-5.21260377162372,22.5,-4.64937620642544));
#453090=CARTESIAN_POINT('Ctrl Pts',(-5.16694476272245,22.5,-4.66349400702439));
#453091=CARTESIAN_POINT('Ctrl Pts',(-5.12221145514625,22.5,-4.68043875311008));
#453092=CARTESIAN_POINT('Ctrl Pts',(-5.07868894891155,22.5,-4.70009846993925));
#453093=CARTESIAN_POINT('Ctrl Pts',(-5.04899063043454,22.5,-4.71351361033608));
#453094=CARTESIAN_POINT('Ctrl Pts',(-5.01985594481751,22.5,-4.72819401862254));
#453095=CARTESIAN_POINT('Ctrl Pts',(-4.99137807959121,22.5,-4.74411779520772));
#453096=CARTESIAN_POINT('Ctrl Pts',(-4.98326708184471,22.5,-4.7486531673282));
#453097=CARTESIAN_POINT('Ctrl Pts',(-4.97520939130455,22.5,-4.75328947002864));
#453098=CARTESIAN_POINT('Ctrl Pts',(-4.96720723120421,22.5,-4.75802635654096));
#453099=CARTESIAN_POINT('Ctrl Pts',(-4.95959010443409,22.5,-4.76253532219619));
#453100=CARTESIAN_POINT('Ctrl Pts',(-4.95203125085003,22.5,-4.7671307305627));
#453101=CARTESIAN_POINT('Ctrl Pts',(-4.9445336523536,22.5,-4.7718108799136));
#453102=CARTESIAN_POINT('Ctrl Pts',(-4.90274986936038,22.5,-4.79789314411416));
#453103=CARTESIAN_POINT('Ctrl Pts',(-4.86285502943318,22.5,-4.82661085167514));
#453104=CARTESIAN_POINT('Ctrl Pts',(-4.8251433783959,22.5,-4.85783224388052));
#453105=CARTESIAN_POINT('Ctrl Pts',(-4.80185182464605,22.5,-4.87711526954221));
#453106=CARTESIAN_POINT('Ctrl Pts',(-4.77939307023024,22.5,-4.89735438380168));
#453107=CARTESIAN_POINT('Ctrl Pts',(-4.75783901282981,22.5,-4.9185281570127));
#453108=CARTESIAN_POINT('Ctrl Pts',(-4.72385034361532,22.5,-4.95191715474625));
#453109=CARTESIAN_POINT('Ctrl Pts',(-4.69210932076016,22.5,-4.98762826934674));
#453110=CARTESIAN_POINT('Ctrl Pts',(-4.66265412509274,22.5,-5.02537769858573));
#453111=CARTESIAN_POINT('Ctrl Pts',(-4.6560648934672,22.5,-5.03382237964628));
#453112=CARTESIAN_POINT('Ctrl Pts',(-4.64959018439674,22.5,-5.04236922197827));
#453113=CARTESIAN_POINT('Ctrl Pts',(-4.64323066288715,22.5,-5.0510153031233));
#453114=CARTESIAN_POINT('Ctrl Pts',(-4.63787530250376,22.5,-5.05829617800763));
#453115=CARTESIAN_POINT('Ctrl Pts',(-4.63260299858695,22.5,-5.06564571347538));
#453116=CARTESIAN_POINT('Ctrl Pts',(-4.62742036976986,22.5,-5.07305265326631));
#453117=CARTESIAN_POINT('Ctrl Pts',(-4.59922209456066,22.5,-5.1133532292971));
#453118=CARTESIAN_POINT('Ctrl Pts',(-4.57362076195032,22.5,-5.15542403890062));
#453119=CARTESIAN_POINT('Ctrl Pts',(-4.55062598363731,22.5,-5.19892882014737));
#453120=CARTESIAN_POINT('Ctrl Pts',(-4.52705592795066,22.5,-5.24352199267827));
#453121=CARTESIAN_POINT('Ctrl Pts',(-4.50622389127859,22.5,-5.28962259952057));
#453122=CARTESIAN_POINT('Ctrl Pts',(-4.48817542914079,22.5,-5.33691174803316));
#453123=CARTESIAN_POINT('Ctrl Pts',(-4.47740085896262,22.5,-5.36514242195013));
#453124=CARTESIAN_POINT('Ctrl Pts',(-4.46761902476255,22.5,-5.39379744246496));
#453125=CARTESIAN_POINT('Ctrl Pts',(-4.45884671156451,22.5,-5.42281409041283));
#453126=CARTESIAN_POINT('Ctrl Pts',(-4.45401588344527,22.5,-5.4387932780761));
#453127=CARTESIAN_POINT('Ctrl Pts',(-4.44949130093593,22.5,-5.4548821891158));
#453128=CARTESIAN_POINT('Ctrl Pts',(-4.44527653009828,22.5,-5.47107067790065));
#453129=CARTESIAN_POINT('Ctrl Pts',(-4.44297713122391,22.5,-5.47990242565713));
#453130=CARTESIAN_POINT('Ctrl Pts',(-4.440770475048,22.5,-5.48876206576444));
#453131=CARTESIAN_POINT('Ctrl Pts',(-4.43865905400722,22.5,-5.49763888076378));
#453132=CARTESIAN_POINT('Ctrl Pts',(-4.42647927126125,22.5,-5.54884500028241));
#453133=CARTESIAN_POINT('Ctrl Pts',(-4.41744307912653,22.5,-5.60070295235243));
#453134=CARTESIAN_POINT('Ctrl Pts',(-4.41160594326508,22.5,-5.6528725699911));
#453135=CARTESIAN_POINT('Ctrl Pts',(-4.40762924378005,22.5,-5.68841446871037));
#453136=CARTESIAN_POINT('Ctrl Pts',(-4.40513819218018,22.5,-5.72410179510797));
#453137=CARTESIAN_POINT('Ctrl Pts',(-4.4041629320734,22.5,-5.75983273067766));
#453138=CARTESIAN_POINT('Ctrl Pts',(-4.40371155802747,22.5,-5.77636987481073));
#453139=CARTESIAN_POINT('Ctrl Pts',(-4.4035852965957,22.5,-5.79292145727197));
#453140=CARTESIAN_POINT('Ctrl Pts',(-4.40378695835951,22.5,-5.80944675448204));
#453141=CARTESIAN_POINT('Ctrl Pts',(-4.40443526815635,22.5,-5.86257289934304));
#453142=CARTESIAN_POINT('Ctrl Pts',(-4.40846556104334,22.5,-5.91547919606967));
#453143=CARTESIAN_POINT('Ctrl Pts',(-4.41595519072995,22.5,-5.96783294665298));
#453144=CARTESIAN_POINT('Ctrl Pts',(-4.41992831408015,22.5,-5.99560573617887));
#453145=CARTESIAN_POINT('Ctrl Pts',(-4.42487575252807,22.5,-6.02322332002059));
#453146=CARTESIAN_POINT('Ctrl Pts',(-4.43081497898236,22.5,-6.05063695240159));
#453147=CARTESIAN_POINT('Ctrl Pts',(-4.43420326443596,22.5,-6.06627623009907));
#453148=CARTESIAN_POINT('Ctrl Pts',(-4.43791441703144,22.5,-6.0818491333573));
#453149=CARTESIAN_POINT('Ctrl Pts',(-4.44194158662795,22.5,-6.09735008669015));
#453150=CARTESIAN_POINT('Ctrl Pts',(-6.64591806159944,22.5,4.8286920333622));
#453151=CARTESIAN_POINT('Ctrl Pts',(-6.6755807993511,22.5,4.8719367804586));
#453152=CARTESIAN_POINT('Ctrl Pts',(-6.7022744086721,22.5,4.91697381282208));
#453153=CARTESIAN_POINT('Ctrl Pts',(-6.72600910610866,22.5,4.96347942286292));
#453154=CARTESIAN_POINT('Ctrl Pts',(-6.750020047493,22.5,5.01052630347802));
#453155=CARTESIAN_POINT('Ctrl Pts',(-6.77100289981649,22.5,5.05907736675444));
#453156=CARTESIAN_POINT('Ctrl Pts',(-6.78891649180094,22.5,5.10881343934042));
#453157=CARTESIAN_POINT('Ctrl Pts',(-6.80187230118985,22.5,5.14478450961691));
#453158=CARTESIAN_POINT('Ctrl Pts',(-6.81322157811539,22.5,5.18137581815852));
#453159=CARTESIAN_POINT('Ctrl Pts',(-6.82293175279788,22.5,5.21846626007043));
#453160=CARTESIAN_POINT('Ctrl Pts',(-6.82709087591091,22.5,5.23435307151024));
#453161=CARTESIAN_POINT('Ctrl Pts',(-6.83094910537833,22.5,5.25033142515782));
#453162=CARTESIAN_POINT('Ctrl Pts',(-6.83450307899072,22.5,5.26639159475908));
#453163=CARTESIAN_POINT('Ctrl Pts',(-6.83669994896103,22.5,5.27631910355995));
#453164=CARTESIAN_POINT('Ctrl Pts',(-6.83878067254843,22.5,5.28627904830748));
#453165=CARTESIAN_POINT('Ctrl Pts',(-6.8407413340506,22.5,5.29625198803563));
#453166=CARTESIAN_POINT('Ctrl Pts',(-6.8506853116647,22.5,5.34683220766748));
#453167=CARTESIAN_POINT('Ctrl Pts',(-6.85756855483867,22.5,5.39784710619139));
#453168=CARTESIAN_POINT('Ctrl Pts',(-6.86136063349203,22.5,5.44899668904261));
#453169=CARTESIAN_POINT('Ctrl Pts',(-6.86506621320742,22.5,5.4989795280052));
#453170=CARTESIAN_POINT('Ctrl Pts',(-6.86581982211597,22.5,5.5490920296864));
#453171=CARTESIAN_POINT('Ctrl Pts',(-6.86354521214504,22.5,5.59904614057211));
#453172=CARTESIAN_POINT('Ctrl Pts',(-6.86196264982713,22.5,5.63380176660143));
#453173=CARTESIAN_POINT('Ctrl Pts',(-6.8589132351154,22.5,5.66848055894767));
#453174=CARTESIAN_POINT('Ctrl Pts',(-6.85435789423314,22.5,5.70297915970175));
#453175=CARTESIAN_POINT('Ctrl Pts',(-6.85274935356602,22.5,5.71516099278645));
#453176=CARTESIAN_POINT('Ctrl Pts',(-6.85095294339145,22.5,5.72732029612368));
#453177=CARTESIAN_POINT('Ctrl Pts',(-6.84896661767721,22.5,5.73945229469627));
#453178=CARTESIAN_POINT('Ctrl Pts',(-6.84749968518305,22.5,5.74841196470285));
#453179=CARTESIAN_POINT('Ctrl Pts',(-6.84592925290685,22.5,5.75735562780225));
#453180=CARTESIAN_POINT('Ctrl Pts',(-6.84425708000572,22.5,5.76626920948405));
#453181=CARTESIAN_POINT('Ctrl Pts',(-6.83533972771596,22.5,5.81380349733577));
#453182=CARTESIAN_POINT('Ctrl Pts',(-6.82351786783565,22.5,5.86057802478339));
#453183=CARTESIAN_POINT('Ctrl Pts',(-6.80873145101255,22.5,5.90632961568247));
#453184=CARTESIAN_POINT('Ctrl Pts',(-6.79814742532969,22.5,5.93907832139669));
#453185=CARTESIAN_POINT('Ctrl Pts',(-6.78604349575646,22.5,5.97130269582608));
#453186=CARTESIAN_POINT('Ctrl Pts',(-6.77238316128915,22.5,6.00289829431615));
#453187=CARTESIAN_POINT('Ctrl Pts',(-6.75417864027363,22.5,6.0450043450931));
#453188=CARTESIAN_POINT('Ctrl Pts',(-6.73321019789003,22.5,6.08599501913005));
#453189=CARTESIAN_POINT('Ctrl Pts',(-6.70966855565445,22.5,6.12568011956913));
#453190=CARTESIAN_POINT('Ctrl Pts',(-6.7034609849824,22.5,6.13614447303852));
#453191=CARTESIAN_POINT('Ctrl Pts',(-6.69707438313333,22.5,6.14651787724421));
#453192=CARTESIAN_POINT('Ctrl Pts',(-6.69051202329594,22.5,6.1567964532414));
#453193=CARTESIAN_POINT('Ctrl Pts',(-6.68556313820106,22.5,6.1645478556042));
#453194=CARTESIAN_POINT('Ctrl Pts',(-6.68051415741144,22.5,6.17224531908615));
#453195=CARTESIAN_POINT('Ctrl Pts',(-6.67537489370653,22.5,6.17987521950616));
#453196=CARTESIAN_POINT('Ctrl Pts',(-6.64842476800822,22.5,6.21988616021516));
#453197=CARTESIAN_POINT('Ctrl Pts',(-6.61894162118579,22.5,6.25812741389502));
#453198=CARTESIAN_POINT('Ctrl Pts',(-6.58718324857477,22.5,6.29441170508163));
#453199=CARTESIAN_POINT('Ctrl Pts',(-6.55551163440422,22.5,6.33059687379256));
#453200=CARTESIAN_POINT('Ctrl Pts',(-6.52157609274862,22.5,6.36483641843439));
#453201=CARTESIAN_POINT('Ctrl Pts',(-6.48560329463389,22.5,6.39690234758754));
#453202=CARTESIAN_POINT('Ctrl Pts',(-6.46634118614209,22.5,6.41407247164262));
#453203=CARTESIAN_POINT('Ctrl Pts',(-6.44649455990001,22.5,6.4306185942519));
#453204=CARTESIAN_POINT('Ctrl Pts',(-6.42609644704949,22.5,6.44649972121378));
#453205=CARTESIAN_POINT('Ctrl Pts',(-6.41550137797154,22.5,6.45474860376629));
#453206=CARTESIAN_POINT('Ctrl Pts',(-6.40475750978787,22.5,6.4628180032753));
#453207=CARTESIAN_POINT('Ctrl Pts',(-6.39386942293182,22.5,6.47070167883221));
#453208=CARTESIAN_POINT('Ctrl Pts',(-6.38552919004326,22.5,6.47674054415646));
#453209=CARTESIAN_POINT('Ctrl Pts',(-6.37710396981869,22.5,6.48267052688883));
#453210=CARTESIAN_POINT('Ctrl Pts',(-6.3686084992472,22.5,6.48848046699456));
#453211=CARTESIAN_POINT('Ctrl Pts',(-6.33038178361366,22.5,6.51462321287319));
#453212=CARTESIAN_POINT('Ctrl Pts',(-6.29067294990532,22.5,6.53838419602365));
#453213=CARTESIAN_POINT('Ctrl Pts',(-6.24968947065537,22.5,6.55954587128772));
#453214=CARTESIAN_POINT('Ctrl Pts',(-6.22204346329034,22.5,6.57382078988697));
#453215=CARTESIAN_POINT('Ctrl Pts',(-6.19381707848861,22.5,6.58691199084907));
#453216=CARTESIAN_POINT('Ctrl Pts',(-6.16507260006602,22.5,6.59873928456135));
#453217=CARTESIAN_POINT('Ctrl Pts',(-6.15266397566519,22.5,6.60384497627704));
#453218=CARTESIAN_POINT('Ctrl Pts',(-6.14015674565985,22.5,6.6087155221976));
#453219=CARTESIAN_POINT('Ctrl Pts',(-6.12757735912736,22.5,6.61333659561112));
#453220=CARTESIAN_POINT('Ctrl Pts',(-6.08619113936898,22.5,6.6285399411254));
#453221=CARTESIAN_POINT('Ctrl Pts',(-6.04397428614735,22.5,6.64106838659551));
#453222=CARTESIAN_POINT('Ctrl Pts',(-6.00111091245467,22.5,6.65070263630215));
#453223=CARTESIAN_POINT('Ctrl Pts',(-5.9799119455316,22.5,6.65546745351706));
#453224=CARTESIAN_POINT('Ctrl Pts',(-5.9585548202981,22.5,6.65952358177373));
#453225=CARTESIAN_POINT('Ctrl Pts',(-5.93706218561481,22.5,6.66283972884874));
#453226=CARTESIAN_POINT('Ctrl Pts',(-5.92425778841234,22.5,6.66481534816931));
#453227=CARTESIAN_POINT('Ctrl Pts',(-5.91140530098883,22.5,6.6665282555788));
#453228=CARTESIAN_POINT('Ctrl Pts',(-5.89851203167795,22.5,6.66798006829994));
#453229=CARTESIAN_POINT('Ctrl Pts',(-4.62591736201901,22.5,5.7755760807344));
#453230=CARTESIAN_POINT('Ctrl Pts',(-4.61585820529768,22.5,5.73330573132647));
#453231=CARTESIAN_POINT('Ctrl Pts',(-4.60871311258362,22.5,5.69054013141041));
#453232=CARTESIAN_POINT('Ctrl Pts',(-4.60431335211636,22.5,5.64753211382414));
#453233=CARTESIAN_POINT('Ctrl Pts',(-4.59971226726699,22.5,5.60255613397471));
#453234=CARTESIAN_POINT('Ctrl Pts',(-4.59811321835512,22.5,5.55731429097459));
#453235=CARTESIAN_POINT('Ctrl Pts',(-4.59937363334914,22.5,5.51206909395162));
#453236=CARTESIAN_POINT('Ctrl Pts',(-4.60034453139405,22.5,5.47721670522309));
#453237=CARTESIAN_POINT('Ctrl Pts',(-4.60301317840841,22.5,5.4423616330738));
#453238=CARTESIAN_POINT('Ctrl Pts',(-4.60733474482685,22.5,5.40761856297945));
#453239=CARTESIAN_POINT('Ctrl Pts',(-4.60876999454272,22.5,5.39607992706529));
#453240=CARTESIAN_POINT('Ctrl Pts',(-4.61038770273571,22.5,5.38455362898469));
#453241=CARTESIAN_POINT('Ctrl Pts',(-4.61218665035847,22.5,5.37304385091102));
#453242=CARTESIAN_POINT('Ctrl Pts',(-4.61342523552785,22.5,5.365119306447));
#453243=CARTESIAN_POINT('Ctrl Pts',(-4.61474939985228,22.5,5.35720517119277));
#453244=CARTESIAN_POINT('Ctrl Pts',(-4.61615691484389,22.5,5.3493113876807));
#453245=CARTESIAN_POINT('Ctrl Pts',(-4.6244083908066,22.5,5.30303453429517));
#453246=CARTESIAN_POINT('Ctrl Pts',(-4.63553334207333,22.5,5.25737359664772));
#453247=CARTESIAN_POINT('Ctrl Pts',(-4.64937620705251,22.5,5.21260376959567));
#453248=CARTESIAN_POINT('Ctrl Pts',(-4.6634940077344,22.5,5.16694476072476));
#453249=CARTESIAN_POINT('Ctrl Pts',(-4.6804387539006,22.5,5.12221145318303));
#453250=CARTESIAN_POINT('Ctrl Pts',(-4.70009847080866,22.5,5.07868894698685));
#453251=CARTESIAN_POINT('Ctrl Pts',(-4.71351361118775,22.5,5.0489906286946));
#453252=CARTESIAN_POINT('Ctrl Pts',(-4.72819401944222,22.5,5.0198559432582));
#453253=CARTESIAN_POINT('Ctrl Pts',(-4.74411779598172,22.5,4.991378078207));
#453254=CARTESIAN_POINT('Ctrl Pts',(-4.7486531689218,22.5,4.98326707902134));
#453255=CARTESIAN_POINT('Ctrl Pts',(-4.75328947247782,22.5,4.9752093870611));
#453256=CARTESIAN_POINT('Ctrl Pts',(-4.75802635988146,22.5,4.96720722556103));
#453257=CARTESIAN_POINT('Ctrl Pts',(-4.76253532466324,22.5,4.95959010036734));
#453258=CARTESIAN_POINT('Ctrl Pts',(-4.76713073211599,22.5,4.95203124834462));
#453259=CARTESIAN_POINT('Ctrl Pts',(-4.77181088052091,22.5,4.94453365138069));
#453260=CARTESIAN_POINT('Ctrl Pts',(-4.79789314476199,22.5,4.90274986841753));
#453261=CARTESIAN_POINT('Ctrl Pts',(-4.82661085236217,22.5,4.86285502852259));
#453262=CARTESIAN_POINT('Ctrl Pts',(-4.85783224460585,22.5,4.82514337751978));
#453263=CARTESIAN_POINT('Ctrl Pts',(-4.87711527004975,22.5,4.80185182408287));
#453264=CARTESIAN_POINT('Ctrl Pts',(-4.89735438406717,22.5,4.77939306995998));
#453265=CARTESIAN_POINT('Ctrl Pts',(-4.9185281570127,22.5,4.75783901282981));
#453266=CARTESIAN_POINT('Ctrl Pts',(-4.95191715474625,22.5,4.72385034361533));
#453267=CARTESIAN_POINT('Ctrl Pts',(-4.98762826934672,22.5,4.69210932076018));
#453268=CARTESIAN_POINT('Ctrl Pts',(-5.02537769858569,22.5,4.66265412509277));
#453269=CARTESIAN_POINT('Ctrl Pts',(-5.03382237968492,22.5,4.65606489343705));
#453270=CARTESIAN_POINT('Ctrl Pts',(-5.04236922205654,22.5,4.64959018433745));
#453271=CARTESIAN_POINT('Ctrl Pts',(-5.05101530324207,22.5,4.64323066279978));
#453272=CARTESIAN_POINT('Ctrl Pts',(-5.05829617806584,22.5,4.6378753024624));
#453273=CARTESIAN_POINT('Ctrl Pts',(-5.06564571347179,22.5,4.63260299859024));
#453274=CARTESIAN_POINT('Ctrl Pts',(-5.07305265319997,22.5,4.62742036981628));
#453275=CARTESIAN_POINT('Ctrl Pts',(-5.11335322922775,22.5,4.59922209460497));
#453276=CARTESIAN_POINT('Ctrl Pts',(-5.15542403882833,22.5,4.5736207619924));
#453277=CARTESIAN_POINT('Ctrl Pts',(-5.19892882007228,22.5,4.550625983677));
#453278=CARTESIAN_POINT('Ctrl Pts',(-5.24352199260122,22.5,4.5270559279874));
#453279=CARTESIAN_POINT('Ctrl Pts',(-5.28962259944175,22.5,4.50622389131235));
#453280=CARTESIAN_POINT('Ctrl Pts',(-5.33691174795269,22.5,4.4881754291715));
#453281=CARTESIAN_POINT('Ctrl Pts',(-5.3651424218722,22.5,4.47740085899016));
#453282=CARTESIAN_POINT('Ctrl Pts',(-5.39379744238978,22.5,4.46761902478714));
#453283=CARTESIAN_POINT('Ctrl Pts',(-5.4228140903405,22.5,4.45884671158638));
#453284=CARTESIAN_POINT('Ctrl Pts',(-5.43879327798787,22.5,4.45401588347092));
#453285=CARTESIAN_POINT('Ctrl Pts',(-5.45488218901142,22.5,4.44949130096477));
#453286=CARTESIAN_POINT('Ctrl Pts',(-5.47107067778001,22.5,4.44527653012968));
#453287=CARTESIAN_POINT('Ctrl Pts',(-5.47990242551106,22.5,4.44297713126103));
#453288=CARTESIAN_POINT('Ctrl Pts',(-5.48876206559289,22.5,4.44077047509027));
#453289=CARTESIAN_POINT('Ctrl Pts',(-5.49763888056664,22.5,4.43865905405411));
#453290=CARTESIAN_POINT('Ctrl Pts',(-5.54884500008372,22.5,4.42647927130003));
#453291=CARTESIAN_POINT('Ctrl Pts',(-5.60070295215265,22.5,4.41744307915717));
#453292=CARTESIAN_POINT('Ctrl Pts',(-5.65287256979064,22.5,4.41160594328751));
#453293=CARTESIAN_POINT('Ctrl Pts',(-5.68841446847963,22.5,4.40762924380021));
#453294=CARTESIAN_POINT('Ctrl Pts',(-5.72410179484693,22.5,4.40513819219555));
#453295=CARTESIAN_POINT('Ctrl Pts',(-5.7598327303865,22.5,4.40416293208135));
#453296=CARTESIAN_POINT('Ctrl Pts',(-5.77636987462536,22.5,4.40371155802871));
#453297=CARTESIAN_POINT('Ctrl Pts',(-5.79292145719268,22.5,4.40358529659437));
#453298=CARTESIAN_POINT('Ctrl Pts',(-5.80944675450856,22.5,4.40378695835983));
#453299=CARTESIAN_POINT('Ctrl Pts',(-5.86257289936903,22.5,4.40443526815779));
#453300=CARTESIAN_POINT('Ctrl Pts',(-5.9154791960951,22.5,4.40846556104586));
#453301=CARTESIAN_POINT('Ctrl Pts',(-5.96783294667778,22.5,4.41595519073349));
#453302=CARTESIAN_POINT('Ctrl Pts',(-5.99560573619532,22.5,4.41992831408309));
#453303=CARTESIAN_POINT('Ctrl Pts',(-6.02322332002874,22.5,4.42487575252983));
#453304=CARTESIAN_POINT('Ctrl Pts',(-6.05063695240159,22.5,4.43081497898236));
#453305=CARTESIAN_POINT('Ctrl Pts',(-6.06627623009907,22.5,4.43420326443596));
#453306=CARTESIAN_POINT('Ctrl Pts',(-6.0818491333573,22.5,4.43791441703144));
#453307=CARTESIAN_POINT('Ctrl Pts',(-6.09735008669016,22.5,4.44194158662795));
#453308=CARTESIAN_POINT('',(3.50148276475995,22.5,3.50148276475995));
#453309=CARTESIAN_POINT('Origin',(0.,22.5,0.));
#453310=CARTESIAN_POINT('Origin',(5.65685387860011,26.,5.65685387860011));
#453311=CARTESIAN_POINT('Origin',(0.,25.,0.));
#453312=CARTESIAN_POINT('',(6.92964645562817,23.5,6.92964645562816));
#453313=CARTESIAN_POINT('Origin',(0.,23.5,0.));
#453314=CARTESIAN_POINT('',(6.92964645562817,25.,6.92964645562816));
#453315=CARTESIAN_POINT('',(6.92964645562816,25.,6.92964645562817));
#453316=CARTESIAN_POINT('Origin',(0.,25.,0.));
#453317=CARTESIAN_POINT('Origin',(0.,14.8,0.));
#453318=CARTESIAN_POINT('',(2.47487373415291,13.3,2.47487373415291));
#453319=CARTESIAN_POINT('',(1.41421356237307,14.8,1.41421356237307));
#453320=CARTESIAN_POINT('Origin',(0.,13.3,0.));
#453321=CARTESIAN_POINT('Origin',(0.,14.8,0.));
#453322=CARTESIAN_POINT('',(2.47487373415292,0.,2.47487373415292));
#453323=CARTESIAN_POINT('',(2.47487373415292,14.8,2.47487373415292));
#453324=CARTESIAN_POINT('Origin',(0.,0.,0.));
#453325=CARTESIAN_POINT('Origin',(0.,0.,0.));
#453326=CARTESIAN_POINT('',(7.42462120245875,25.,7.42462120245875));
#453327=CARTESIAN_POINT('Origin',(0.,25.,0.));
#453328=CARTESIAN_POINT('',(7.42462120245875,0.,7.42462120245875));
#453329=CARTESIAN_POINT('Origin',(0.,0.,0.));
#453330=CARTESIAN_POINT('',(7.42462120245875,23.5,7.42462120245875));
#453331=CARTESIAN_POINT('',(7.42462120245875,0.,7.42462120245875));
#453332=CARTESIAN_POINT('Origin',(0.,23.5,0.));
#453333=CARTESIAN_POINT('Origin',(0.,0.,0.));
#453334=CARTESIAN_POINT('',(3.50148276475995,21.,3.50148276475995));
#453335=CARTESIAN_POINT('Origin',(0.,21.,0.));
#453336=CARTESIAN_POINT('',(3.50148276475995,0.,3.50148276475995));
#453337=CARTESIAN_POINT('Origin',(0.,0.,0.));
#453338=CARTESIAN_POINT('',(7.42462120245875,20.,7.42462120245875));
#453339=CARTESIAN_POINT('Origin',(0.,20.,0.));
#453340=CARTESIAN_POINT('',(7.42462120245875,21.,7.42462120245875));
#453341=CARTESIAN_POINT('',(7.42462120245875,0.,7.42462120245875));
#453342=CARTESIAN_POINT('Origin',(0.,21.,0.));
#453343=CARTESIAN_POINT('Origin',(0.,0.,0.));
#453344=CARTESIAN_POINT('',(3.59412750505487,18.5,3.59412750505487));
#453345=CARTESIAN_POINT('Origin',(0.,18.5,0.));
#453346=CARTESIAN_POINT('',(3.59412750505487,20.,3.59412750505487));
#453347=CARTESIAN_POINT('',(3.59412750505487,0.,3.59412750505487));
#453348=CARTESIAN_POINT('Origin',(0.,20.,0.));
#453349=CARTESIAN_POINT('Origin',(0.,0.,0.));
#453350=CARTESIAN_POINT('',(7.42462120245875,17.5,7.42462120245875));
#453351=CARTESIAN_POINT('Origin',(0.,17.5,0.));
#453352=CARTESIAN_POINT('',(7.42462120245875,18.5,7.42462120245875));
#453353=CARTESIAN_POINT('',(7.42462120245875,0.,7.42462120245875));
#453354=CARTESIAN_POINT('Origin',(0.,18.5,0.));
#453355=CARTESIAN_POINT('Origin',(0.,0.,0.));
#453356=CARTESIAN_POINT('',(3.68677224534978,16.,3.68677224534978));
#453357=CARTESIAN_POINT('Origin',(0.,16.,0.));
#453358=CARTESIAN_POINT('',(3.68677224534978,17.5,3.68677224534978));
#453359=CARTESIAN_POINT('',(3.68677224534978,0.,3.68677224534978));
#453360=CARTESIAN_POINT('Origin',(0.,17.5,0.));
#453361=CARTESIAN_POINT('Origin',(0.,0.,0.));
#453362=CARTESIAN_POINT('',(7.42462120245875,15.,7.42462120245875));
#453363=CARTESIAN_POINT('Origin',(0.,15.,0.));
#453364=CARTESIAN_POINT('',(7.42462120245875,16.,7.42462120245875));
#453365=CARTESIAN_POINT('',(7.42462120245875,0.,7.42462120245875));
#453366=CARTESIAN_POINT('Origin',(0.,16.,0.));
#453367=CARTESIAN_POINT('Origin',(0.,0.,0.));
#453368=CARTESIAN_POINT('',(3.7794169856447,13.5,3.7794169856447));
#453369=CARTESIAN_POINT('Origin',(0.,13.5,0.));
#453370=CARTESIAN_POINT('',(3.7794169856447,15.,3.7794169856447));
#453371=CARTESIAN_POINT('',(3.7794169856447,0.,3.7794169856447));
#453372=CARTESIAN_POINT('Origin',(0.,15.,0.));
#453373=CARTESIAN_POINT('Origin',(0.,0.,0.));
#453374=CARTESIAN_POINT('',(7.42462120245875,12.5,7.42462120245875));
#453375=CARTESIAN_POINT('Origin',(0.,12.5,0.));
#453376=CARTESIAN_POINT('',(7.42462120245875,13.5,7.42462120245875));
#453377=CARTESIAN_POINT('',(7.42462120245875,0.,7.42462120245875));
#453378=CARTESIAN_POINT('Origin',(0.,13.5,0.));
#453379=CARTESIAN_POINT('Origin',(0.,0.,0.));
#453380=CARTESIAN_POINT('',(3.87206172593962,11.,3.87206172593962));
#453381=CARTESIAN_POINT('Origin',(0.,11.,0.));
#453382=CARTESIAN_POINT('',(3.87206172593962,12.5,3.87206172593962));
#453383=CARTESIAN_POINT('',(3.87206172593962,0.,3.87206172593962));
#453384=CARTESIAN_POINT('Origin',(0.,12.5,0.));
#453385=CARTESIAN_POINT('Origin',(0.,0.,0.));
#453386=CARTESIAN_POINT('',(7.42462120245875,10.,7.42462120245875));
#453387=CARTESIAN_POINT('Origin',(0.,10.,0.));
#453388=CARTESIAN_POINT('',(7.42462120245875,11.,7.42462120245875));
#453389=CARTESIAN_POINT('',(7.42462120245875,0.,7.42462120245875));
#453390=CARTESIAN_POINT('Origin',(0.,11.,0.));
#453391=CARTESIAN_POINT('Origin',(0.,0.,0.));
#453392=CARTESIAN_POINT('',(3.96470646623454,8.5,3.96470646623454));
#453393=CARTESIAN_POINT('Origin',(0.,8.5,0.));
#453394=CARTESIAN_POINT('',(3.96470646623454,10.,3.96470646623454));
#453395=CARTESIAN_POINT('',(3.96470646623454,0.,3.96470646623454));
#453396=CARTESIAN_POINT('Origin',(0.,10.,0.));
#453397=CARTESIAN_POINT('Origin',(0.,0.,0.));
#453398=CARTESIAN_POINT('',(7.42462120245875,7.5,7.42462120245875));
#453399=CARTESIAN_POINT('Origin',(0.,7.5,0.));
#453400=CARTESIAN_POINT('',(7.42462120245875,8.5,7.42462120245875));
#453401=CARTESIAN_POINT('',(7.42462120245875,0.,7.42462120245875));
#453402=CARTESIAN_POINT('Origin',(0.,8.5,0.));
#453403=CARTESIAN_POINT('Origin',(0.,0.,0.));
#453404=CARTESIAN_POINT('',(4.05735120652945,6.,4.05735120652945));
#453405=CARTESIAN_POINT('Origin',(0.,6.,0.));
#453406=CARTESIAN_POINT('',(4.05735120652945,7.5,4.05735120652945));
#453407=CARTESIAN_POINT('',(4.05735120652945,0.,4.05735120652945));
#453408=CARTESIAN_POINT('Origin',(0.,7.5,0.));
#453409=CARTESIAN_POINT('Origin',(0.,0.,0.));
#453410=CARTESIAN_POINT('',(7.42462120245875,5.,7.42462120245875));
#453411=CARTESIAN_POINT('Origin',(0.,5.,0.));
#453412=CARTESIAN_POINT('',(7.42462120245875,6.,7.42462120245875));
#453413=CARTESIAN_POINT('',(7.42462120245875,0.,7.42462120245875));
#453414=CARTESIAN_POINT('Origin',(0.,6.,0.));
#453415=CARTESIAN_POINT('Origin',(0.,0.,0.));
#453416=CARTESIAN_POINT('',(4.14999594682437,3.5,4.14999594682437));
#453417=CARTESIAN_POINT('Origin',(0.,3.5,0.));
#453418=CARTESIAN_POINT('',(4.14999594682437,5.,4.14999594682437));
#453419=CARTESIAN_POINT('',(4.14999594682437,0.,4.14999594682437));
#453420=CARTESIAN_POINT('Origin',(0.,5.,0.));
#453421=CARTESIAN_POINT('Origin',(0.,0.,0.));
#453422=CARTESIAN_POINT('',(7.42462120245875,2.5,7.42462120245875));
#453423=CARTESIAN_POINT('Origin',(0.,2.5,0.));
#453424=CARTESIAN_POINT('',(7.42462120245875,3.5,7.42462120245875));
#453425=CARTESIAN_POINT('',(7.42462120245875,0.,7.42462120245875));
#453426=CARTESIAN_POINT('Origin',(0.,3.5,0.));
#453427=CARTESIAN_POINT('Origin',(0.,0.,0.));
#453428=CARTESIAN_POINT('',(4.24264068711929,0.999999999999999,4.24264068711929));
#453429=CARTESIAN_POINT('Origin',(0.,0.999999999999999,0.));
#453430=CARTESIAN_POINT('',(4.24264068711929,2.5,4.24264068711929));
#453431=CARTESIAN_POINT('',(4.24264068711929,0.,4.24264068711929));
#453432=CARTESIAN_POINT('Origin',(0.,2.5,0.));
#453433=CARTESIAN_POINT('Origin',(0.,0.,0.));
#453434=CARTESIAN_POINT('',(7.42462120245875,0.,7.42462120245875));
#453435=CARTESIAN_POINT('Origin',(0.,0.,0.));
#453436=CARTESIAN_POINT('',(7.42462120245875,1.,7.42462120245875));
#453437=CARTESIAN_POINT('',(7.42462120245875,0.,7.42462120245875));
#453438=CARTESIAN_POINT('Origin',(0.,1.,0.));
#453439=CARTESIAN_POINT('Origin',(0.,0.,0.));
#453440=CARTESIAN_POINT('Origin',(7.88424061023,1.,-7.88424061023001));
#453441=CARTESIAN_POINT('Origin',(4.24264068711929,2.5,-4.24264068711929));
#453442=CARTESIAN_POINT('Origin',(7.88424061023,3.5,-7.88424061023001));
#453443=CARTESIAN_POINT('Origin',(4.14999594682437,5.,-4.14999594682437));
#453444=CARTESIAN_POINT('Origin',(7.88424061023,6.,-7.88424061023001));
#453445=CARTESIAN_POINT('Origin',(4.05735120652945,7.5,-4.05735120652945));
#453446=CARTESIAN_POINT('Origin',(7.88424061023,8.5,-7.88424061023001));
#453447=CARTESIAN_POINT('Origin',(3.96470646623454,10.,-3.96470646623454));
#453448=CARTESIAN_POINT('Origin',(7.88424061023,11.,-7.88424061023001));
#453449=CARTESIAN_POINT('Origin',(3.87206172593962,12.5,-3.87206172593962));
#453450=CARTESIAN_POINT('Origin',(7.88424061023,13.5,-7.88424061023001));
#453451=CARTESIAN_POINT('Origin',(3.7794169856447,15.,-3.7794169856447));
#453452=CARTESIAN_POINT('Origin',(7.88424061023,16.,-7.88424061023001));
#453453=CARTESIAN_POINT('Origin',(3.68677224534978,17.5,-3.68677224534978));
#453454=CARTESIAN_POINT('Origin',(7.88424061023,18.5,-7.88424061023001));
#453455=CARTESIAN_POINT('Origin',(3.59412750505487,20.,-3.59412750505487));
#453456=CARTESIAN_POINT('Origin',(7.88424061023,21.,-7.88424061023001));
#453457=CARTESIAN_POINT('Origin',(7.88424061023,23.5,-7.88424061023001));
#453458=CARTESIAN_POINT('Origin',(3.40883802446503,25.,-3.40883802446503));
#453459=CARTESIAN_POINT('Origin',(-5.65685387860011,26.993675081176,5.65685387860011));
#453460=CARTESIAN_POINT('Ctrl Pts',(-4.74432962138981,25.868675081176,6.57057130100612));
#453461=CARTESIAN_POINT('Ctrl Pts',(-4.78199706987976,25.8656848283261,
6.60882993708831));
#453462=CARTESIAN_POINT('Ctrl Pts',(-5.14157728587623,25.8388668852448,
6.92960341635462));
#453463=CARTESIAN_POINT('Ctrl Pts',(-6.16255878293893,25.7882212519322,
7.09568592881682));
#453464=CARTESIAN_POINT('Ctrl Pts',(-7.13997732676548,25.716738181238,6.01152748645437));
#453465=CARTESIAN_POINT('Ctrl Pts',(-6.75873746207651,25.6452551105438,
4.60259286076204));
#453466=CARTESIAN_POINT('Ctrl Pts',(-5.36788602689621,25.5737720398497,
4.15947051927595));
#453467=CARTESIAN_POINT('Ctrl Pts',(-4.24182426511434,25.5022889691555,
5.0882746237623));
#453468=CARTESIAN_POINT('Ctrl Pts',(-4.36502559631504,25.450589982931,6.13675122222029));
#453469=CARTESIAN_POINT('Ctrl Pts',(-4.69148744470697,25.4227186869378,
6.51790892062316));
#453470=CARTESIAN_POINT('Ctrl Pts',(-4.74334636410459,25.418675081176,6.56885365284802));
#453471=CARTESIAN_POINT('Ctrl Pts',(-4.7445060113485,25.906324918824,6.56704169373441));
#453472=CARTESIAN_POINT('Ctrl Pts',(-4.9557394479142,25.8898945654199,6.77506586643251));
#453473=CARTESIAN_POINT('Ctrl Pts',(-5.64807137163849,25.8496365217844,
7.11639071403833));
#453474=CARTESIAN_POINT('Ctrl Pts',(-6.8522203629011,25.7855507879174,6.60321033464885));
#453475=CARTESIAN_POINT('Ctrl Pts',(-7.1004834147237,25.7140677172233,5.16550356767203));
#453476=CARTESIAN_POINT('Ctrl Pts',(-6.02596364157129,25.6425846465291,
4.17707919799326));
#453477=CARTESIAN_POINT('Ctrl Pts',(-4.61334644908231,25.5711015758349,
4.5448553014618));
#453478=CARTESIAN_POINT('Ctrl Pts',(-4.21675923787011,25.5090149999332,
5.74896333949311));
#453479=CARTESIAN_POINT('Ctrl Pts',(-4.5629353888518,25.4707561142629,6.3830054663296));
#453480=CARTESIAN_POINT('Ctrl Pts',(-4.74640124271564,25.456324918824,6.56829321884323));
#453481=CARTESIAN_POINT('Ctrl Pts',(-6.69274404704181,26.,5.59475217632212));
#453482=CARTESIAN_POINT('Ctrl Pts',(-6.67208297724159,25.9761723097686,
5.25011429538726));
#453483=CARTESIAN_POINT('Ctrl Pts',(-6.25991935236784,25.9285169293058,
4.58904744425369));
#453484=CARTESIAN_POINT('Ctrl Pts',(-5.08408179813166,25.8570338586116,
4.57111450891619));
#453485=CARTESIAN_POINT('Ctrl Pts',(-4.43501771280631,25.7855507879175,
5.55001366141289));
#453486=CARTESIAN_POINT('Ctrl Pts',(-4.90440858615388,25.7140677172233,
6.62575617389683));
#453487=CARTESIAN_POINT('Ctrl Pts',(-6.06367191307887,25.6425846465291,
6.81433291744693));
#453488=CARTESIAN_POINT('Ctrl Pts',(-6.8499634587037,25.5711015758349,5.94217367437589));
#453489=CARTESIAN_POINT('Ctrl Pts',(-6.54327224197424,25.4996185051408,
4.80874583886255));
#453490=CARTESIAN_POINT('Ctrl Pts',(-5.42439156223909,25.4281354344466,
4.45227280794999));
#453491=CARTESIAN_POINT('Ctrl Pts',(-4.51852288527076,25.3566523637524,
5.19945610983427));
#453492=CARTESIAN_POINT('Ctrl Pts',(-4.65556044151952,25.2851692930583,
6.36568271985868));
#453493=CARTESIAN_POINT('Ctrl Pts',(-5.70997789504277,25.213686222364,6.88249940298929));
#453494=CARTESIAN_POINT('Ctrl Pts',(-6.71571945020394,25.1422031516699,
6.27639179734011));
#453495=CARTESIAN_POINT('Ctrl Pts',(-6.7513451989237,25.0707200809757,5.10267450019953));
#453496=CARTESIAN_POINT('Ctrl Pts',(-5.78421192833874,24.9992370102815,
4.43668748453226));
#453497=CARTESIAN_POINT('Ctrl Pts',(-4.7003955508837,24.9277539395873,4.88860074260097));
#453498=CARTESIAN_POINT('Ctrl Pts',(-4.49287282235237,24.8562708688931,
6.04437662247732));
#453499=CARTESIAN_POINT('Ctrl Pts',(-5.35177365831406,24.784787798199,6.84510966506768));
#453500=CARTESIAN_POINT('Ctrl Pts',(-6.49018471285717,24.7133047275048,
6.55717903824976));
#453501=CARTESIAN_POINT('Ctrl Pts',(-6.86510957377001,24.6418216568106,
5.44438294256281));
#453502=CARTESIAN_POINT('Ctrl Pts',(-6.13304718756447,24.5703385861164,
4.52624977050191));
#453503=CARTESIAN_POINT('Ctrl Pts',(-4.96470306042394,24.4988555154223,
4.64396052187117));
#453504=CARTESIAN_POINT('Ctrl Pts',(-4.43049797487471,24.4273724447281,
5.68967021074952));
#453505=CARTESIAN_POINT('Ctrl Pts',(-5.01986328076134,24.3558893740339,
6.70531403099034));
#453506=CARTESIAN_POINT('Ctrl Pts',(-6.19283059794665,24.2844063033397,
6.76037309820141));
#453507=CARTESIAN_POINT('Ctrl Pts',(-6.87474342740735,24.2129232326455,
5.80440305573226));
#453508=CARTESIAN_POINT('Ctrl Pts',(-6.44084262551864,24.1414401619514,
4.71325048867858));
#453509=CARTESIAN_POINT('Ctrl Pts',(-5.28866213152759,24.0699570912572,
4.48661435222159));
#453510=CARTESIAN_POINT('Ctrl Pts',(-4.47381384511066,23.9984740205631,
5.33213555135881));
#453511=CARTESIAN_POINT('Ctrl Pts',(-4.74285054378755,23.9269909498688,
6.47515921171813));
#453512=CARTESIAN_POINT('Ctrl Pts',(-5.84928450947304,23.8555078791747,
6.86846279219781));
#453513=CARTESIAN_POINT('Ctrl Pts',(-6.77941618151556,23.7840248084805,
6.15170698086798));
#453514=CARTESIAN_POINT('Ctrl Pts',(-6.68107173221035,23.7125417377863,
4.98157355760958));
#453515=CARTESIAN_POINT('Ctrl Pts',(-5.64435299191054,23.6410586670921,
4.43012269359922));
#453516=CARTESIAN_POINT('Ctrl Pts',(-4.61908739135743,23.569575596398,5.00258598787076));
#453517=CARTESIAN_POINT('Ctrl Pts',(-4.54460915448657,23.4980925257038,
6.17448062637044));
#453518=CARTESIAN_POINT('Ctrl Pts',(-5.48915421344717,23.4266094550096,
6.87213254456038));
#453519=CARTESIAN_POINT('Ctrl Pts',(-6.5873433994568,23.3551263843154,6.45636332421143));
#453520=CARTESIAN_POINT('Ctrl Pts',(-6.8330308949199,23.2836433136213,5.30809370313679));
#453521=CARTESIAN_POINT('Ctrl Pts',(-6.00112122066856,23.212160242927,4.47935503415496));
#453522=CARTESIAN_POINT('Ctrl Pts',(-4.85379852261456,23.1406771722329,
4.72942128924326));
#453523=CARTESIAN_POINT('Ctrl Pts',(-4.44222413342345,23.0691941015387,
5.82919498069919));
#453524=CARTESIAN_POINT('Ctrl Pts',(-5.14347668616413,22.9977110308445,
6.77105943752211));
#453525=CARTESIAN_POINT('Ctrl Pts',(-6.31507855179966,22.9262279601504,
6.69212899367236));
#453526=CARTESIAN_POINT('Ctrl Pts',(-6.88362364563197,22.8547448894562,
5.66464494341573));
#453527=CARTESIAN_POINT('Ctrl Pts',(-6.32821994284799,22.783261818762,4.63011853598606));
#453528=CARTESIAN_POINT('Ctrl Pts',(-5.15771839492687,22.7117787480678,
4.53608521045973));
#453529=CARTESIAN_POINT('Ctrl Pts',(-4.4445208236608,22.6402956773736,5.46925286619012));
#453530=CARTESIAN_POINT('Ctrl Pts',(-4.84204067651847,22.5688126066795,
6.57357515235991));
#453531=CARTESIAN_POINT('Ctrl Pts',(-5.98608844956735,22.4973295359852,
6.8394368280484));
#453532=CARTESIAN_POINT('Ctrl Pts',(-6.82851835303725,22.4258464652911,
6.01893246982621));
#453533=CARTESIAN_POINT('Ctrl Pts',(-6.67416374956871,22.3781910848283,
5.25534692011694));
#453534=CARTESIAN_POINT('Ctrl Pts',(-6.45251384441992,22.3543633945969,
4.99063298333217));
#453535=CARTESIAN_POINT('Ctrl Pts',(-6.77667668816907,26.0485455351344,
5.58972040746333));
#453536=CARTESIAN_POINT('Ctrl Pts',(-6.75434156236399,26.024717844903,5.21715836192049));
#453537=CARTESIAN_POINT('Ctrl Pts',(-6.30878252293169,25.9770624644402,
4.50252879876621));
#453538=CARTESIAN_POINT('Ctrl Pts',(-5.03767313923882,25.905579393746,4.4831428535712));
#453539=CARTESIAN_POINT('Ctrl Pts',(-4.33601886182374,25.8340963230518,
5.54135696992154));
#453540=CARTESIAN_POINT('Ctrl Pts',(-4.84344196766209,25.7626132523576,
6.70426114586778));
#453541=CARTESIAN_POINT('Ctrl Pts',(-6.09663420303223,25.6911301816635,
6.90811725457023));
#453542=CARTESIAN_POINT('Ctrl Pts',(-6.94663474805762,25.6196471109693,
5.96529161173539));
#453543=CARTESIAN_POINT('Ctrl Pts',(-6.61509398200833,25.5481640402751,
4.7400281794957));
#453544=CARTESIAN_POINT('Ctrl Pts',(-5.40555638379146,25.4766809695809,
4.35467204505866));
#453545=CARTESIAN_POINT('Ctrl Pts',(-4.42629001188529,25.4051978988867,
5.16239561447694));
#453546=CARTESIAN_POINT('Ctrl Pts',(-4.57443098853515,25.3337148281926,
6.42311533054124));
#453547=CARTESIAN_POINT('Ctrl Pts',(-5.71428225002475,25.2622317574984,
6.98180690592903));
#453548=CARTESIAN_POINT('Ctrl Pts',(-6.80151366539291,25.1907486868042,
6.32658964203686));
#453549=CARTESIAN_POINT('Ctrl Pts',(-6.84002597802966,25.11926561611,5.05777230853438));
#453550=CARTESIAN_POINT('Ctrl Pts',(-5.79453107008661,25.0477825454159,
4.33782392622387));
#453551=CARTESIAN_POINT('Ctrl Pts',(-4.62289884706407,24.9762994747217,
4.82635329907546));
#453552=CARTESIAN_POINT('Ctrl Pts',(-4.39856166152736,24.9048164040275,
6.07577551821105));
#453553=CARTESIAN_POINT('Ctrl Pts',(-5.32705463942152,24.8333333333333,
6.94138767747801));
#453554=CARTESIAN_POINT('Ctrl Pts',(-6.55770505428216,24.7618502626391,
6.63012757162215));
#453555=CARTESIAN_POINT('Ctrl Pts',(-6.96300807183686,24.690367191945,5.42716755876279));
#453556=CARTESIAN_POINT('Ctrl Pts',(-6.17163058503857,24.6188841212508,
4.4346429653087));
#453557=CARTESIAN_POINT('Ctrl Pts',(-4.90862178076926,24.5474010505566,
4.56189118942602));
#453558=CARTESIAN_POINT('Ctrl Pts',(-4.33113291369596,24.4759179798625,
5.69232914266462));
#453559=CARTESIAN_POINT('Ctrl Pts',(-4.96825133880203,24.4044349091683,
6.79026515070139));
#453560=CARTESIAN_POINT('Ctrl Pts',(-6.23625792548383,24.3329518384741,
6.84978535971091));
#453561=CARTESIAN_POINT('Ctrl Pts',(-6.97342250511928,24.2614687677799,
5.81635817656469));
#453562=CARTESIAN_POINT('Ctrl Pts',(-6.50436504145382,24.1899856970857,
4.63679535172919));
#453563=CARTESIAN_POINT('Ctrl Pts',(-5.2588295230962,24.1185026263916,4.39179610102783));
#453564=CARTESIAN_POINT('Ctrl Pts',(-4.37795843727393,24.0470195556974,
5.30582536167067));
#453565=CARTESIAN_POINT('Ctrl Pts',(-4.66879374102307,23.9755364850032,
6.54146211713177));
#453566=CARTESIAN_POINT('Ctrl Pts',(-5.86487613450725,23.904053414309,6.96663298362319));
#453567=CARTESIAN_POINT('Ctrl Pts',(-6.8703714022368,23.8325703436148,6.19180228161384));
#453568=CARTESIAN_POINT('Ctrl Pts',(-6.76405862808226,23.7610872729207,
4.92685920413015));
#453569=CARTESIAN_POINT('Ctrl Pts',(-5.64334011190815,23.6896042022265,
4.33072722538547));
#453570=CARTESIAN_POINT('Ctrl Pts',(-4.53500272215098,23.6181211315323,
4.94957415925549));
#453571=CARTESIAN_POINT('Ctrl Pts',(-4.45448991200439,23.5466380608381,
6.21642115383373));
#453572=CARTESIAN_POINT('Ctrl Pts',(-5.47556640632123,23.475154990144,6.97060007639641));
#453573=CARTESIAN_POINT('Ctrl Pts',(-6.66273598971974,23.4036719194498,
6.52114329936776));
#453574=CARTESIAN_POINT('Ctrl Pts',(-6.92833022917403,23.3321888487556,
5.27983553104633));
#453575=CARTESIAN_POINT('Ctrl Pts',(-6.02901536249358,23.2607057780614,
4.38394859923605));
#453576=CARTESIAN_POINT('Ctrl Pts',(-4.78873124130167,23.1892227073672,
4.6542763857934));
#453577=CARTESIAN_POINT('Ctrl Pts',(-4.34380918016856,23.1177396366731,
5.84315885864169));
#453578=CARTESIAN_POINT('Ctrl Pts',(-5.1018804774459,23.0462565659789,6.86133755596364));
#453579=CARTESIAN_POINT('Ctrl Pts',(-6.36841097734037,22.9747734952847,
6.77601180031397));
#453580=CARTESIAN_POINT('Ctrl Pts',(-6.98302223994139,22.9032904245905,
5.66527621173653));
#453581=CARTESIAN_POINT('Ctrl Pts',(-6.3826171450343,22.8318073538963,4.54692766144197));
#453582=CARTESIAN_POINT('Ctrl Pts',(-5.11727611571493,22.7603242832022,
4.4452753183732));
#453583=CARTESIAN_POINT('Ctrl Pts',(-4.34629195893472,22.688841212508,5.45405255931453));
#453584=CARTESIAN_POINT('Ctrl Pts',(-4.77602071980922,22.6173581418138,
6.64785217518362));
#453585=CARTESIAN_POINT('Ctrl Pts',(-6.01276456633487,22.5458750711197,
6.93525520080945));
#453586=CARTESIAN_POINT('Ctrl Pts',(-6.92345206015257,22.4743920004254,
6.04826976192828));
#453587=CARTESIAN_POINT('Ctrl Pts',(-6.75659092854625,22.4267366199627,
5.22281495825156));
#453588=CARTESIAN_POINT('Ctrl Pts',(-6.5169819168131,22.4029089297313,4.93665266667552));
#453589=CARTESIAN_POINT('Ctrl Pts',(-6.86060932929632,26.0970910702687,
5.58468863860454));
#453590=CARTESIAN_POINT('Ctrl Pts',(-6.83660014748639,26.0732633800373,
5.18420242845371));
#453591=CARTESIAN_POINT('Ctrl Pts',(-6.35764569349554,26.0256079995746,
4.41601015327873));
#453592=CARTESIAN_POINT('Ctrl Pts',(-4.99126448034597,25.9541249288803,
4.39517119822623));
#453593=CARTESIAN_POINT('Ctrl Pts',(-4.23702001084117,25.8826418581862,
5.53270027843017));
#453594=CARTESIAN_POINT('Ctrl Pts',(-4.7824753491703,25.811158787492,6.78276611783875));
#453595=CARTESIAN_POINT('Ctrl Pts',(-6.12959649298558,25.7396757167979,
7.00190159169352));
#453596=CARTESIAN_POINT('Ctrl Pts',(-7.04330603741155,25.6681926461036,
5.98840954909488));
#453597=CARTESIAN_POINT('Ctrl Pts',(-6.68691572204241,25.5967095754095,
4.67131052012887));
#453598=CARTESIAN_POINT('Ctrl Pts',(-5.38672120534384,25.5252265047153,
4.2570712821673));
#453599=CARTESIAN_POINT('Ctrl Pts',(-4.33405713849982,25.4537434340211,
5.12533511911963));
#453600=CARTESIAN_POINT('Ctrl Pts',(-4.49330153555078,25.382260363327,6.48054794122378));
#453601=CARTESIAN_POINT('Ctrl Pts',(-5.71858660500674,25.3107772926328,
7.0811144088688));
#453602=CARTESIAN_POINT('Ctrl Pts',(-6.88730788058188,25.2392942219386,
6.37678748673361));
#453603=CARTESIAN_POINT('Ctrl Pts',(-6.92870675713562,25.1678111512444,
5.01287011686923));
#453604=CARTESIAN_POINT('Ctrl Pts',(-5.80485021183448,25.0963280805502,
4.23896036791547));
#453605=CARTESIAN_POINT('Ctrl Pts',(-4.54540214324445,25.0248450098561,
4.76410585554996));
#453606=CARTESIAN_POINT('Ctrl Pts',(-4.30425050070234,24.9533619391619,
6.10717441394477));
#453607=CARTESIAN_POINT('Ctrl Pts',(-5.302335620529,24.8818788684677,7.03766568988833));
#453608=CARTESIAN_POINT('Ctrl Pts',(-6.62522539570715,24.8103957977735,
6.70307610499455));
#453609=CARTESIAN_POINT('Ctrl Pts',(-7.06090656990369,24.7389127270793,
5.40995217496278));
#453610=CARTESIAN_POINT('Ctrl Pts',(-6.21021398251268,24.6674296563851,
4.34303616011548));
#453611=CARTESIAN_POINT('Ctrl Pts',(-4.85254050111457,24.595946585691,4.47982185698087));
#453612=CARTESIAN_POINT('Ctrl Pts',(-4.23176785251722,24.5244635149968,
5.69498807457971));
#453613=CARTESIAN_POINT('Ctrl Pts',(-4.91663939684271,24.4529804443027,
6.87521627041245));
#453614=CARTESIAN_POINT('Ctrl Pts',(-6.27968525302103,24.3814973736084,
6.93919762122039));
#453615=CARTESIAN_POINT('Ctrl Pts',(-7.07210158283119,24.3100143029143,
5.82831329739714));
#453616=CARTESIAN_POINT('Ctrl Pts',(-6.567887457389,24.2385312322201,4.56034021477979));
#453617=CARTESIAN_POINT('Ctrl Pts',(-5.2289969146648,24.1670481615259,4.29697784983407));
#453618=CARTESIAN_POINT('Ctrl Pts',(-4.28210302943719,24.0955650908318,
5.27951517198252));
#453619=CARTESIAN_POINT('Ctrl Pts',(-4.59473693825861,24.0240820201375,
6.60776502254541));
#453620=CARTESIAN_POINT('Ctrl Pts',(-5.88046775954144,23.9525989494434,
7.06480317504856));
#453621=CARTESIAN_POINT('Ctrl Pts',(-6.96132662295805,23.8811158787492,
6.2318975823597));
#453622=CARTESIAN_POINT('Ctrl Pts',(-6.84704552395415,23.809632808055,4.87214485065071));
#453623=CARTESIAN_POINT('Ctrl Pts',(-5.64232723190575,23.7381497373609,
4.23133175717171));
#453624=CARTESIAN_POINT('Ctrl Pts',(-4.45091805294455,23.6666666666667,
4.89656233064023));
#453625=CARTESIAN_POINT('Ctrl Pts',(-4.3643706695222,23.5951835959725,6.258361681297));
#453626=CARTESIAN_POINT('Ctrl Pts',(-5.46197859919531,23.5237005252783,
7.06906760823243));
#453627=CARTESIAN_POINT('Ctrl Pts',(-6.73812857998267,23.4522174545842,
6.58592327452408));
#453628=CARTESIAN_POINT('Ctrl Pts',(-7.02362956342815,23.3807343838899,
5.25157735895588));
#453629=CARTESIAN_POINT('Ctrl Pts',(-6.05690950431861,23.3092513131958,
4.28854216431713));
#453630=CARTESIAN_POINT('Ctrl Pts',(-4.72366395998878,23.2377682425016,
4.57913148234355));
#453631=CARTESIAN_POINT('Ctrl Pts',(-4.24539422691366,23.1662851718074,
5.85712273658419));
#453632=CARTESIAN_POINT('Ctrl Pts',(-5.06028426872769,23.0948021011132,
6.95161567440517));
#453633=CARTESIAN_POINT('Ctrl Pts',(-6.42174340288107,23.0233190304191,
6.85989460695557));
#453634=CARTESIAN_POINT('Ctrl Pts',(-7.0824208342508,22.9518359597249,5.66590748005734));
#453635=CARTESIAN_POINT('Ctrl Pts',(-6.43701434722061,22.8803528890307,
4.46373678689787));
#453636=CARTESIAN_POINT('Ctrl Pts',(-5.07683383650298,22.8088698183366,
4.35446542628666));
#453637=CARTESIAN_POINT('Ctrl Pts',(-4.24806309420865,22.7373867476423,
5.43885225243895));
#453638=CARTESIAN_POINT('Ctrl Pts',(-4.71000076309996,22.6659036769482,
6.72212919800732));
#453639=CARTESIAN_POINT('Ctrl Pts',(-6.0394406831024,22.594420606254,7.03107357357049));
#453640=CARTESIAN_POINT('Ctrl Pts',(-7.01838576726789,22.5229375355598,
6.07760705403035));
#453641=CARTESIAN_POINT('Ctrl Pts',(-6.83901810752379,22.475282155097,5.19028299638618));
#453642=CARTESIAN_POINT('Ctrl Pts',(-6.58144998920627,22.4514544648656,
4.88267235001886));
#453643=CARTESIAN_POINT('Ctrl Pts',(-6.94454197042357,26.1456366054031,
5.57965686974575));
#453644=CARTESIAN_POINT('Ctrl Pts',(-6.91885873260879,26.1218089151717,
5.15124649498693));
#453645=CARTESIAN_POINT('Ctrl Pts',(-6.40650886405939,26.0741535347089,
4.32949150779126));
#453646=CARTESIAN_POINT('Ctrl Pts',(-4.94485582145312,26.0026704640147,
4.30719954288124));
#453647=CARTESIAN_POINT('Ctrl Pts',(-4.1380211598586,25.9311873933206,5.52404358693882));
#453648=CARTESIAN_POINT('Ctrl Pts',(-4.7215087306785,25.8597043226263,6.86127108980971));
#453649=CARTESIAN_POINT('Ctrl Pts',(-6.16255878293893,25.7882212519322,
7.09568592881682));
#453650=CARTESIAN_POINT('Ctrl Pts',(-7.13997732676548,25.716738181238,6.01152748645437));
#453651=CARTESIAN_POINT('Ctrl Pts',(-6.75873746207651,25.6452551105438,
4.60259286076204));
#453652=CARTESIAN_POINT('Ctrl Pts',(-5.36788602689621,25.5737720398497,
4.15947051927595));
#453653=CARTESIAN_POINT('Ctrl Pts',(-4.24182426511434,25.5022889691555,
5.0882746237623));
#453654=CARTESIAN_POINT('Ctrl Pts',(-4.41217208256641,25.4308058984613,
6.53798055190634));
#453655=CARTESIAN_POINT('Ctrl Pts',(-5.72289095998872,25.3593228277671,
7.18042191180854));
#453656=CARTESIAN_POINT('Ctrl Pts',(-6.97310209577086,25.287839757073,6.42698533143036));
#453657=CARTESIAN_POINT('Ctrl Pts',(-7.01738753624157,25.2163566863788,
4.96796792520407));
#453658=CARTESIAN_POINT('Ctrl Pts',(-5.81516935358237,25.1448736156846,
4.14009680960707));
#453659=CARTESIAN_POINT('Ctrl Pts',(-4.4679054394248,25.0733905449904,4.70185841202445));
#453660=CARTESIAN_POINT('Ctrl Pts',(-4.20993933987732,25.0019074742962,
6.13857330967851));
#453661=CARTESIAN_POINT('Ctrl Pts',(-5.27761660163647,24.930424403602,7.13394370229865));
#453662=CARTESIAN_POINT('Ctrl Pts',(-6.69274573713214,24.8589413329079,
6.77602463836695));
#453663=CARTESIAN_POINT('Ctrl Pts',(-7.15880506797054,24.7874582622137,
5.39273679116275));
#453664=CARTESIAN_POINT('Ctrl Pts',(-6.24879737998678,24.7159751915195,
4.25142935492228));
#453665=CARTESIAN_POINT('Ctrl Pts',(-4.79645922145989,24.6444921208253,
4.39775252453571));
#453666=CARTESIAN_POINT('Ctrl Pts',(-4.13240279133847,24.5730090501312,
5.69764700649482));
#453667=CARTESIAN_POINT('Ctrl Pts',(-4.86502745488341,24.501525979437,6.9601673901235));
#453668=CARTESIAN_POINT('Ctrl Pts',(-6.32311258055822,24.4300429087428,
7.0286098827299));
#453669=CARTESIAN_POINT('Ctrl Pts',(-7.17078066054311,24.3585598380486,
5.84026841822956));
#453670=CARTESIAN_POINT('Ctrl Pts',(-6.63140987332417,24.2870767673545,
4.4838850778304));
#453671=CARTESIAN_POINT('Ctrl Pts',(-5.19916430623342,24.2155936966603,
4.2021595986403));
#453672=CARTESIAN_POINT('Ctrl Pts',(-4.18624762160046,24.1441106259661,
5.25320498229437));
#453673=CARTESIAN_POINT('Ctrl Pts',(-4.52068013549415,24.0726275552719,
6.67406792795905));
#453674=CARTESIAN_POINT('Ctrl Pts',(-5.89605938457563,24.0011444845777,
7.16297336647392));
#453675=CARTESIAN_POINT('Ctrl Pts',(-7.0522818436793,23.9296614138836,6.27199288310558));
#453676=CARTESIAN_POINT('Ctrl Pts',(-6.93003241982605,23.8581783431894,
4.81743049717126));
#453677=CARTESIAN_POINT('Ctrl Pts',(-5.64131435190337,23.7866952724952,
4.13193628895796));
#453678=CARTESIAN_POINT('Ctrl Pts',(-4.3668333837381,23.715212201801,4.84355050202496));
#453679=CARTESIAN_POINT('Ctrl Pts',(-4.27425142704003,23.6437291311069,
6.30030220876029));
#453680=CARTESIAN_POINT('Ctrl Pts',(-5.44839079206937,23.5722460604127,
7.16753514006844));
#453681=CARTESIAN_POINT('Ctrl Pts',(-6.81352117024561,23.5007629897185,
6.65070324968042));
#453682=CARTESIAN_POINT('Ctrl Pts',(-7.11892889768229,23.4292799190243,
5.22331918686542));
#453683=CARTESIAN_POINT('Ctrl Pts',(-6.08480364614363,23.3577968483302,
4.19313572939823));
#453684=CARTESIAN_POINT('Ctrl Pts',(-4.65859667867589,23.2863137776359,
4.50398657889369));
#453685=CARTESIAN_POINT('Ctrl Pts',(-4.14697927365876,23.2148307069418,
5.8710866145267));
#453686=CARTESIAN_POINT('Ctrl Pts',(-5.01868806000948,23.1433476362476,
7.04189379284668));
#453687=CARTESIAN_POINT('Ctrl Pts',(-6.47507582842176,23.0718645655535,
6.94377741359718));
#453688=CARTESIAN_POINT('Ctrl Pts',(-7.18181942856023,23.0003814948592,
5.66653874837814));
#453689=CARTESIAN_POINT('Ctrl Pts',(-6.49141154940691,22.9288984241651,
4.38054591235378));
#453690=CARTESIAN_POINT('Ctrl Pts',(-5.03639155729104,22.8574153534709,
4.26365553420012));
#453691=CARTESIAN_POINT('Ctrl Pts',(-4.14983422948258,22.7859322827767,
5.42365194556336));
#453692=CARTESIAN_POINT('Ctrl Pts',(-4.6439808063907,22.7144492120825,6.79640622083105));
#453693=CARTESIAN_POINT('Ctrl Pts',(-6.06611679986992,22.6429661413884,
7.12689194633153));
#453694=CARTESIAN_POINT('Ctrl Pts',(-7.11331947438321,22.5714830706942,
6.10694434613243));
#453695=CARTESIAN_POINT('Ctrl Pts',(-6.92144528650133,22.5238276902314,
5.15775103452081));
#453696=CARTESIAN_POINT('Ctrl Pts',(-6.64591806159944,22.5,4.8286920333622));
#453697=CARTESIAN_POINT('Ctrl Pts',(-4.92197603118329,25.2730384757729,
6.39051881327128));
#453698=CARTESIAN_POINT('Ctrl Pts',(-4.8802577415671,25.2770820815347,6.34953594825859));
#453699=CARTESIAN_POINT('Ctrl Pts',(-4.84215579969383,25.2811256872965,
6.3050503566324));
#453700=CARTESIAN_POINT('Ctrl Pts',(-4.80845709106527,25.2851692930582,
6.25744773204304));
#453701=CARTESIAN_POINT('Ctrl Pts',(-4.60988125610327,25.3089969832896,
5.97694051651721));
#453702=CARTESIAN_POINT('Ctrl Pts',(-4.56420207068701,25.332824673521,5.58819831317574));
#453703=CARTESIAN_POINT('Ctrl Pts',(-4.69234059080694,25.3566523637524,
5.26929666119096));
#453704=CARTESIAN_POINT('Ctrl Pts',(-4.82047911092687,25.3804800539838,
4.95039500920618));
#453705=CARTESIAN_POINT('Ctrl Pts',(-5.12243533658298,25.4043077442152,
4.70133390857808));
#453706=CARTESIAN_POINT('Ctrl Pts',(-5.45989356270023,25.4281354344466,
4.6362155300828));
#453707=CARTESIAN_POINT('Ctrl Pts',(-5.79735178881747,25.451963124678,4.57109715158751));
#453708=CARTESIAN_POINT('Ctrl Pts',(-6.17031201539585,25.4757908149094,
4.68992149522503));
#453709=CARTESIAN_POINT('Ctrl Pts',(-6.40790733147329,25.4996185051408,
4.93823830629601));
#453710=CARTESIAN_POINT('Ctrl Pts',(-6.64550264755072,25.5234461953722,
5.186555117367));
#453711=CARTESIAN_POINT('Ctrl Pts',(-6.74773305312721,25.5472738856035,
5.56436439587144));
#453712=CARTESIAN_POINT('Ctrl Pts',(-6.66779966497798,25.5711015758349,
5.89862890896884));
#453713=CARTESIAN_POINT('Ctrl Pts',(-6.58786627682875,25.5949292660663,
6.23289342206624));
#453714=CARTESIAN_POINT('Ctrl Pts',(-6.32576909495381,25.6187569562977,
6.52361316975658));
#453715=CARTESIAN_POINT('Ctrl Pts',(-6.00150994952884,25.6425846465291,
6.63754358634341));
#453716=CARTESIAN_POINT('Ctrl Pts',(-5.67725080410387,25.6664123367605,
6.75147400293023));
#453717=CARTESIAN_POINT('Ctrl Pts',(-5.29082969512888,25.6902400269919,
6.68861508841353));
#453718=CARTESIAN_POINT('Ctrl Pts',(-5.01938732841678,25.7140677172233,
6.47789521240786));
#453719=CARTESIAN_POINT('Ctrl Pts',(-4.98532270432787,25.7170579700732,
6.45145094929911));
#453720=CARTESIAN_POINT('Ctrl Pts',(-4.95306887608107,25.720048222923,6.42267802952733));
#453721=CARTESIAN_POINT('Ctrl Pts',(-4.92276701974739,25.7230384757729,
6.39190058798136));
#453722=CARTESIAN_POINT('Ctrl Pts',(-4.53900700771688,26.,5.01302286563431));
#453723=CARTESIAN_POINT('Ctrl Pts',(-4.32480615636363,25.9761723097686,
5.38492752167559));
#453724=CARTESIAN_POINT('Ctrl Pts',(-4.30067277954968,25.9285169293058,
6.35301914505848));
#453725=CARTESIAN_POINT('Ctrl Pts',(-5.50907794609548,25.8570338586117,
7.17562648915451));
#453726=CARTESIAN_POINT('Ctrl Pts',(-6.8522203629011,25.7855507879174,6.60321033464885));
#453727=CARTESIAN_POINT('Ctrl Pts',(-7.1004834147237,25.7140677172233,5.16550356767203));
#453728=CARTESIAN_POINT('Ctrl Pts',(-6.02596364157129,25.6425846465291,
4.17707919799326));
#453729=CARTESIAN_POINT('Ctrl Pts',(-4.61334644908231,25.5711015758349,
4.5448553014618));
#453730=CARTESIAN_POINT('Ctrl Pts',(-4.15673773385264,25.4996185051408,
5.93119910857215));
#453731=CARTESIAN_POINT('Ctrl Pts',(-5.07453447980768,25.4281354344466,
7.06630891143689));
#453732=CARTESIAN_POINT('Ctrl Pts',(-6.5258341885166,25.3566523637524,6.91003560334641));
#453733=CARTESIAN_POINT('Ctrl Pts',(-7.18099123031483,25.2851692930582,
5.60564496305));
#453734=CARTESIAN_POINT('Ctrl Pts',(-6.43975200870338,25.213686222364,4.34815567114859));
#453735=CARTESIAN_POINT('Ctrl Pts',(-4.98123363545819,25.1422031516699,
4.28968558428151));
#453736=CARTESIAN_POINT('Ctrl Pts',(-4.14170854437417,25.0707200809757,
5.48379221455872));
#453737=CARTESIAN_POINT('Ctrl Pts',(-4.69033908735646,24.9992370102815,
6.83645762028281));
#453738=CARTESIAN_POINT('Ctrl Pts',(-6.12447699388038,24.9277539395873,
7.10838527255516));
#453739=CARTESIAN_POINT('Ctrl Pts',(-7.13018513270865,24.8562708688931,
6.05044038944422));
#453740=CARTESIAN_POINT('Ctrl Pts',(-6.78604742232836,24.784787798199,4.63189669239788));
#453741=CARTESIAN_POINT('Ctrl Pts',(-5.40735816264999,24.7133047275048,
4.15240479236238));
#453742=CARTESIAN_POINT('Ctrl Pts',(-4.25725342975252,24.6418216568106,
5.05126835371239));
#453743=CARTESIAN_POINT('Ctrl Pts',(-4.38944335790392,24.5703385861164,
6.50496106867921));
#453744=CARTESIAN_POINT('Ctrl Pts',(-5.68281734635597,24.4988555154223,
7.18162963832199));
#453745=CARTESIAN_POINT('Ctrl Pts',(-6.95240396480877,24.4273724447281,
6.4613196666284));
#453746=CARTESIAN_POINT('Ctrl Pts',(-7.03502543671246,24.3558893740339,
5.00396921476326));
#453747=CARTESIAN_POINT('Ctrl Pts',(-5.85498510857851,24.2844063033397,
4.14478270244581));
#453748=CARTESIAN_POINT('Ctrl Pts',(-4.49341967622111,24.2129232326456,
4.67093497503136));
#453749=CARTESIAN_POINT('Ctrl Pts',(-4.19777663638434,24.1414401619514,
6.10037256921808));
#453750=CARTESIAN_POINT('Ctrl Pts',(-5.23892007073304,24.0699570912572,
7.12346444664167));
#453751=CARTESIAN_POINT('Ctrl Pts',(-6.662968703113,23.998474020563,6.80286792203874));
#453752=CARTESIAN_POINT('Ctrl Pts',(-7.16522879152533,23.9269909498688,
5.43230911237055));
#453753=CARTESIAN_POINT('Ctrl Pts',(-6.2855365564656,23.8555078791747,4.26747512907024));
#453754=CARTESIAN_POINT('Ctrl Pts',(-4.82985391579145,23.7840248084805,
4.37557081254884));
#453755=CARTESIAN_POINT('Ctrl Pts',(-4.13185724083954,23.7125417377863,
5.6575604101698));
#453756=CARTESIAN_POINT('Ctrl Pts',(-4.83104150205929,23.6410586670921,
6.93890266242659));
#453757=CARTESIAN_POINT('Ctrl Pts',(-6.28682364983266,23.569575596398,7.04564953674368));
#453758=CARTESIAN_POINT('Ctrl Pts',(-7.16543624640093,23.4980925257038,
5.88000083782648));
#453759=CARTESIAN_POINT('Ctrl Pts',(-6.66190630419616,23.4266094550096,
4.50990820099156));
#453760=CARTESIAN_POINT('Ctrl Pts',(-5.23756146736659,23.3551263843154,
4.19063094092434));
#453761=CARTESIAN_POINT('Ctrl Pts',(-4.19736598356862,23.2836433136212,
5.21468783779196));
#453762=CARTESIAN_POINT('Ctrl Pts',(-4.49433434427902,23.2121602429271,
6.64384941569999));
#453763=CARTESIAN_POINT('Ctrl Pts',(-5.85638486317849,23.1406771722329,
7.16874271925581));
#453764=CARTESIAN_POINT('Ctrl Pts',(-7.03563221165043,23.0691941015387,
6.3084575374563));
#453765=CARTESIAN_POINT('Ctrl Pts',(-6.95165327175697,22.9977110308445,
4.85119529970875));
#453766=CARTESIAN_POINT('Ctrl Pts',(-5.68141376558384,22.9262279601503,
4.13204038713623));
#453767=CARTESIAN_POINT('Ctrl Pts',(-4.38863987327371,22.8547448894562,
4.80994952176022));
#453768=CARTESIAN_POINT('Ctrl Pts',(-4.25785081625158,22.783261818762,6.26368089065206));
#453769=CARTESIAN_POINT('Ctrl Pts',(-5.40868234342554,22.7117787480678,
7.16164157512573));
#453770=CARTESIAN_POINT('Ctrl Pts',(-6.78713386963137,22.6402956773736,
6.6805523241845));
#453771=CARTESIAN_POINT('Ctrl Pts',(-7.12954990426925,22.5688126066795,
5.26231872215201));
#453772=CARTESIAN_POINT('Ctrl Pts',(-6.12366999440581,22.4973295359852,
4.20406666678212));
#453773=CARTESIAN_POINT('Ctrl Pts',(-4.68809392709695,22.4258464652911,
4.47983331463011));
#453774=CARTESIAN_POINT('Ctrl Pts',(-4.32622391325397,22.3781910848283,
5.37807265034296));
#453775=CARTESIAN_POINT('Ctrl Pts',(-4.37532354240196,22.3543633945969,
5.80443435631943));
#453776=CARTESIAN_POINT('Ctrl Pts',(-4.61186924884874,26.0485455351344,
5.05498833669907));
#453777=CARTESIAN_POINT('Ctrl Pts',(-4.41163019717349,26.024717844903,5.40265192052163));
#453778=CARTESIAN_POINT('Ctrl Pts',(-4.38906985506273,25.9770624644402,
6.30764248137266));
#453779=CARTESIAN_POINT('Ctrl Pts',(-5.51871011120511,25.905579393746,7.07663155607638));
#453780=CARTESIAN_POINT('Ctrl Pts',(-6.77430532526158,25.8340963230518,
6.54152598941931));
#453781=CARTESIAN_POINT('Ctrl Pts',(-7.00638637325414,25.7626132523577,
5.1975302126156));
#453782=CARTESIAN_POINT('Ctrl Pts',(-6.00190474293836,25.6911301816635,
4.27353221173564));
#453783=CARTESIAN_POINT('Ctrl Pts',(-4.68136318011483,25.6196471109693,
4.61733634566934));
#453784=CARTESIAN_POINT('Ctrl Pts',(-4.25451662209878,25.5481640402751,
5.91331704545575));
#453785=CARTESIAN_POINT('Ctrl Pts',(-5.11249056981941,25.4766809695809,
6.97443939411569));
#453786=CARTESIAN_POINT('Ctrl Pts',(-6.46919328847102,25.4051978988868,
6.82835211754091));
#453787=CARTESIAN_POINT('Ctrl Pts',(-7.08164661869466,25.3337148281926,
5.60898280515531));
#453788=CARTESIAN_POINT('Ctrl Pts',(-6.38872202076577,25.2622317574984,
4.43345777007097));
#453789=CARTESIAN_POINT('Ctrl Pts',(-5.02527115647435,25.1907486868042,
4.37879881483496));
#453790=CARTESIAN_POINT('Ctrl Pts',(-4.24046704839446,25.1192656161101,
5.49507252586478));
#453791=CARTESIAN_POINT('Ctrl Pts',(-4.75333737058416,25.0477825454159,
6.75957001205556));
#453792=CARTESIAN_POINT('Ctrl Pts',(-6.09399690839474,24.9762994747217,
7.01377318104996));
#453793=CARTESIAN_POINT('Ctrl Pts',(-7.03415210716631,24.9048164040275,
6.0247860748808));
#453794=CARTESIAN_POINT('Ctrl Pts',(-6.71244559509181,24.8333333333333,
4.69870430227372));
#453795=CARTESIAN_POINT('Ctrl Pts',(-5.42362051261082,24.7618502626392,
4.25046610554157));
#453796=CARTESIAN_POINT('Ctrl Pts',(-4.34848061663154,24.6903671919449,
5.09074095026354));
#453797=CARTESIAN_POINT('Ctrl Pts',(-4.47205428913018,24.6188841212508,
6.44968069692277));
#453798=CARTESIAN_POINT('Ctrl Pts',(-5.68112502471735,24.5474010505566,
7.08224341470704));
#453799=CARTESIAN_POINT('Ctrl Pts',(-6.86795887198032,24.4759179798625,
6.40888387979891));
#453800=CARTESIAN_POINT('Ctrl Pts',(-6.94519500375797,24.4044349091682,
5.04652481074591));
#453801=CARTESIAN_POINT('Ctrl Pts',(-5.84207074093975,24.3329518384741,
4.24334083014216));
#453802=CARTESIAN_POINT('Ctrl Pts',(-4.56925333967074,24.2614687677799,
4.73519803534796));
#453803=CARTESIAN_POINT('Ctrl Pts',(-4.29288057290861,24.1899856970857,
6.07146363130893));
#453804=CARTESIAN_POINT('Ctrl Pts',(-5.2661613635068,24.1185026263916,7.02786948132164));
#453805=CARTESIAN_POINT('Ctrl Pts',(-6.59738925492609,24.0470195556973,
6.72816971985337));
#453806=CARTESIAN_POINT('Ctrl Pts',(-7.0669115895136,23.9755364850032,5.44694513750786));
#453807=CARTESIAN_POINT('Ctrl Pts',(-6.2445584671913,23.904053414309,4.35803605660743));
#453808=CARTESIAN_POINT('Ctrl Pts',(-4.88375849993059,23.8325703436148,
4.4590859684691));
#453809=CARTESIAN_POINT('Ctrl Pts',(-4.23125786147911,23.7610872729207,
5.65751435782136));
#453810=CARTESIAN_POINT('Ctrl Pts',(-4.88486867828213,23.6896042022265,
6.85533759634902));
#453811=CARTESIAN_POINT('Ctrl Pts',(-6.24576166668191,23.6181211315323,
6.95512661561532));
#453812=CARTESIAN_POINT('Ctrl Pts',(-7.06710552229816,23.5466380608381,
5.86545592297768));
#453813=CARTESIAN_POINT('Ctrl Pts',(-6.59639610410402,23.475154990144,4.58466712791061));
#453814=CARTESIAN_POINT('Ctrl Pts',(-5.26489131510139,23.4036719194498,
4.28620064015657));
#453815=CARTESIAN_POINT('Ctrl Pts',(-4.29249668680419,23.3321888487556,
5.24350860879812));
#453816=CARTESIAN_POINT('Ctrl Pts',(-4.57010838886107,23.2607057780614,
6.57951617946397));
#453817=CARTESIAN_POINT('Ctrl Pts',(-5.84337925830513,23.1892227073672,
7.07019647634744));
#453818=CARTESIAN_POINT('Ctrl Pts',(-6.94576222857241,23.1177396366731,
6.26598543850372));
#453819=CARTESIAN_POINT('Ctrl Pts',(-6.86725710976116,23.0462565659789,
4.90370883369462));
#453820=CARTESIAN_POINT('Ctrl Pts',(-5.67981293057308,22.9747734952847,
4.23142907013928));
#453821=CARTESIAN_POINT('Ctrl Pts',(-4.47130317633407,22.9032904245905,
4.86515149178938));
#453822=CARTESIAN_POINT('Ctrl Pts',(-4.34903906495375,22.8318073538964,
6.22412737287685));
#453823=CARTESIAN_POINT('Ctrl Pts',(-5.42485838212006,22.7603242832022,
7.06355819103049));
#453824=CARTESIAN_POINT('Ctrl Pts',(-6.7134612268051,22.688841212508,6.613826760128));
#453825=CARTESIAN_POINT('Ctrl Pts',(-7.03355828347467,22.6173581418138,
5.28803487026933));
#453826=CARTESIAN_POINT('Ctrl Pts',(-6.0932425098549,22.5458750711196,4.29876061359894));
#453827=CARTESIAN_POINT('Ctrl Pts',(-4.75123855184286,22.4743920004255,
4.55655254906459));
#453828=CARTESIAN_POINT('Ctrl Pts',(-4.41295554342414,22.4267366199627,
5.39624385572484));
#453829=CARTESIAN_POINT('Ctrl Pts',(-4.45885481560765,22.4029089297313,
5.79481493112442));
#453830=CARTESIAN_POINT('Ctrl Pts',(-4.6847314899806,26.0970910702687,5.09695380776383));
#453831=CARTESIAN_POINT('Ctrl Pts',(-4.49845423798335,26.0732633800373,
5.42037631936769));
#453832=CARTESIAN_POINT('Ctrl Pts',(-4.47746693057576,26.0256079995745,
6.26226581768684));
#453833=CARTESIAN_POINT('Ctrl Pts',(-5.52834227631476,25.9541249288804,
6.97763662299825));
#453834=CARTESIAN_POINT('Ctrl Pts',(-6.69639028762206,25.8826418581862,
6.47984164418979));
#453835=CARTESIAN_POINT('Ctrl Pts',(-6.91228933178459,25.811158787492,5.22955685755916));
#453836=CARTESIAN_POINT('Ctrl Pts',(-5.97784584430541,25.7396757167978,
4.36998522547805));
#453837=CARTESIAN_POINT('Ctrl Pts',(-4.74937991114736,25.6681926461037,
4.68981738987686));
#453838=CARTESIAN_POINT('Ctrl Pts',(-4.35229551034491,25.5967095754095,
5.89543498233936));
#453839=CARTESIAN_POINT('Ctrl Pts',(-5.15044665983114,25.5252265047153,
6.88256987679448));
#453840=CARTESIAN_POINT('Ctrl Pts',(-6.41255238842542,25.4537434340211,
6.74666863173542));
#453841=CARTESIAN_POINT('Ctrl Pts',(-6.9823020070745,25.3822603633269,5.61232064726061));
#453842=CARTESIAN_POINT('Ctrl Pts',(-6.33769203282816,25.3107772926328,
4.51875986899336));
#453843=CARTESIAN_POINT('Ctrl Pts',(-5.06930867749051,25.2392942219386,
4.46791204538842));
#453844=CARTESIAN_POINT('Ctrl Pts',(-4.33922555241473,25.1678111512444,
5.50635283717083));
#453845=CARTESIAN_POINT('Ctrl Pts',(-4.81633565381188,25.0963280805502,
6.68268240382831));
#453846=CARTESIAN_POINT('Ctrl Pts',(-6.06351682290909,25.0248450098561,
6.91916108954474));
#453847=CARTESIAN_POINT('Ctrl Pts',(-6.93811908162397,24.9533619391618,
5.99913176031738));
#453848=CARTESIAN_POINT('Ctrl Pts',(-6.63884376785526,24.8818788684677,
4.76551191214957));
#453849=CARTESIAN_POINT('Ctrl Pts',(-5.43988286257165,24.8103957977735,
4.34852741872076));
#453850=CARTESIAN_POINT('Ctrl Pts',(-4.43970780351055,24.7389127270793,
5.13021354681469));
#453851=CARTESIAN_POINT('Ctrl Pts',(-4.55466522035644,24.6674296563852,
6.39440032516631));
#453852=CARTESIAN_POINT('Ctrl Pts',(-5.67943270307874,24.595946585691,6.9828571910921));
#453853=CARTESIAN_POINT('Ctrl Pts',(-6.78351377915185,24.5244635149968,
6.35644809296942));
#453854=CARTESIAN_POINT('Ctrl Pts',(-6.85536457080349,24.4529804443026,
5.08908040672856));
#453855=CARTESIAN_POINT('Ctrl Pts',(-5.82915637330098,24.3814973736085,
4.34189895783853));
#453856=CARTESIAN_POINT('Ctrl Pts',(-4.64508700312038,24.3100143029143,
4.79946109566455));
#453857=CARTESIAN_POINT('Ctrl Pts',(-4.38798450943289,24.2385312322201,
6.0425546933998));
#453858=CARTESIAN_POINT('Ctrl Pts',(-5.29340265628057,24.1670481615259,
6.93227451600161));
#453859=CARTESIAN_POINT('Ctrl Pts',(-6.53180980673917,24.0955650908317,
6.65347151766801));
#453860=CARTESIAN_POINT('Ctrl Pts',(-6.96859438750187,24.0240820201376,
5.46158116264517));
#453861=CARTESIAN_POINT('Ctrl Pts',(-6.20358037791699,23.9525989494434,
4.44859698414461));
#453862=CARTESIAN_POINT('Ctrl Pts',(-4.93766308406974,23.8811158787492,
4.54260112438938));
#453863=CARTESIAN_POINT('Ctrl Pts',(-4.33065848211867,23.809632808055,5.65746830547292));
#453864=CARTESIAN_POINT('Ctrl Pts',(-4.93869585450498,23.7381497373608,
6.77177253027144));
#453865=CARTESIAN_POINT('Ctrl Pts',(-6.20469968353116,23.6666666666667,
6.86460369448697));
#453866=CARTESIAN_POINT('Ctrl Pts',(-6.96877479819537,23.5951835959725,
5.85091100812889));
#453867=CARTESIAN_POINT('Ctrl Pts',(-6.53088590401187,23.5237005252783,
4.65942605482967));
#453868=CARTESIAN_POINT('Ctrl Pts',(-5.29222116283617,23.4522174545841,
4.3817703393888));
#453869=CARTESIAN_POINT('Ctrl Pts',(-4.38762739003978,23.38073438389,5.27232937980428));
#453870=CARTESIAN_POINT('Ctrl Pts',(-4.6458824334431,23.3092513131958,6.51518294322794));
#453871=CARTESIAN_POINT('Ctrl Pts',(-5.83037365343178,23.2377682425016,
6.97165023343906));
#453872=CARTESIAN_POINT('Ctrl Pts',(-6.85589224549438,23.1662851718074,
6.22351333955115));
#453873=CARTESIAN_POINT('Ctrl Pts',(-6.78286094776533,23.0948021011132,
4.9562223676805));
#453874=CARTESIAN_POINT('Ctrl Pts',(-5.67821209556232,23.0233190304191,
4.33081775314232));
#453875=CARTESIAN_POINT('Ctrl Pts',(-4.55396647939442,22.9518359597249,
4.92035346181854));
#453876=CARTESIAN_POINT('Ctrl Pts',(-4.44022731365593,22.8803528890307,
6.18457385510163));
#453877=CARTESIAN_POINT('Ctrl Pts',(-5.44103442081457,22.8088698183366,
6.96547480693525));
#453878=CARTESIAN_POINT('Ctrl Pts',(-6.63978858397884,22.7373867476423,
6.5471011960715));
#453879=CARTESIAN_POINT('Ctrl Pts',(-6.93756666268008,22.6659036769482,
5.31375101838666));
#453880=CARTESIAN_POINT('Ctrl Pts',(-6.06281502530401,22.594420606254,4.39345456041576));
#453881=CARTESIAN_POINT('Ctrl Pts',(-4.81438317658877,22.5229375355598,
4.63327178349907));
#453882=CARTESIAN_POINT('Ctrl Pts',(-4.49968717359432,22.475282155097,5.41441506110672));
#453883=CARTESIAN_POINT('Ctrl Pts',(-4.54238608881333,22.4514544648656,
5.78519550592941));
#453884=CARTESIAN_POINT('Ctrl Pts',(-4.75759373111246,26.1456366054031,
5.13891927882859));
#453885=CARTESIAN_POINT('Ctrl Pts',(-4.58527827879321,26.1218089151717,
5.43810071821374));
#453886=CARTESIAN_POINT('Ctrl Pts',(-4.5658640060888,26.0741535347089,6.21688915400102));
#453887=CARTESIAN_POINT('Ctrl Pts',(-5.53797444142439,26.0026704640147,
6.87864168992013));
#453888=CARTESIAN_POINT('Ctrl Pts',(-6.61847524998255,25.9311873933205,
6.41815729896025));
#453889=CARTESIAN_POINT('Ctrl Pts',(-6.81819229031504,25.8597043226264,
5.26158350250274));
#453890=CARTESIAN_POINT('Ctrl Pts',(-5.95378694567247,25.7882212519322,
4.46643823922044));
#453891=CARTESIAN_POINT('Ctrl Pts',(-4.81739664217988,25.716738181238,4.76229843408439));
#453892=CARTESIAN_POINT('Ctrl Pts',(-4.45007439859105,25.6452551105439,
5.87755291922296));
#453893=CARTESIAN_POINT('Ctrl Pts',(-5.18840274984287,25.5737720398496,
6.79070035947327));
#453894=CARTESIAN_POINT('Ctrl Pts',(-6.35591148837984,25.5022889691555,
6.66498514592993));
#453895=CARTESIAN_POINT('Ctrl Pts',(-6.88295739545434,25.4308058984613,
5.61565848936591));
#453896=CARTESIAN_POINT('Ctrl Pts',(-6.28666204489054,25.3593228277671,
4.60406196791575));
#453897=CARTESIAN_POINT('Ctrl Pts',(-5.11334619850669,25.2878397570729,
4.55702527594187));
#453898=CARTESIAN_POINT('Ctrl Pts',(-4.43798405643501,25.2163566863788,
5.5176331484769));
#453899=CARTESIAN_POINT('Ctrl Pts',(-4.87933393703958,25.1448736156846,
6.60579479560105));
#453900=CARTESIAN_POINT('Ctrl Pts',(-6.03303673742344,25.0733905449905,
6.82454899803953));
#453901=CARTESIAN_POINT('Ctrl Pts',(-6.84208605608162,25.0019074742962,
5.97347744575396));
#453902=CARTESIAN_POINT('Ctrl Pts',(-6.56524194061871,24.9304244036021,
4.83231952202541));
#453903=CARTESIAN_POINT('Ctrl Pts',(-5.45614521253248,24.8589413329079,
4.44658873189996));
#453904=CARTESIAN_POINT('Ctrl Pts',(-4.53093499038958,24.7874582622137,
5.16968614336582));
#453905=CARTESIAN_POINT('Ctrl Pts',(-4.63727615158269,24.7159751915195,
6.33911995340987));
#453906=CARTESIAN_POINT('Ctrl Pts',(-5.67774038144014,24.6444921208253,
6.88347096747714));
#453907=CARTESIAN_POINT('Ctrl Pts',(-6.6990686863234,24.5730090501312,6.30401230613993));
#453908=CARTESIAN_POINT('Ctrl Pts',(-6.76553413784902,24.501525979437,5.13163600271121));
#453909=CARTESIAN_POINT('Ctrl Pts',(-5.81624200566219,24.4300429087428,
4.44045708553489));
#453910=CARTESIAN_POINT('Ctrl Pts',(-4.72092066657003,24.3585598380486,
4.86372415598115));
#453911=CARTESIAN_POINT('Ctrl Pts',(-4.48308844595715,24.2870767673544,
6.01364575549064));
#453912=CARTESIAN_POINT('Ctrl Pts',(-5.32064394905434,24.2155936966603,
6.83667955068161));
#453913=CARTESIAN_POINT('Ctrl Pts',(-6.46623035855224,24.1441106259661,
6.57877331548262));
#453914=CARTESIAN_POINT('Ctrl Pts',(-6.87027718549015,24.0726275552719,
5.4762171877825));
#453915=CARTESIAN_POINT('Ctrl Pts',(-6.16260228864268,24.0011444845777,
4.53915791168179));
#453916=CARTESIAN_POINT('Ctrl Pts',(-4.99156766820889,23.9296614138836,
4.62611628030965));
#453917=CARTESIAN_POINT('Ctrl Pts',(-4.43005910275823,23.8581783431894,
5.65742225312448));
#453918=CARTESIAN_POINT('Ctrl Pts',(-4.99252303072782,23.7866952724952,
6.68820746419386));
#453919=CARTESIAN_POINT('Ctrl Pts',(-6.16363770038041,23.715212201801,6.77408077335862));
#453920=CARTESIAN_POINT('Ctrl Pts',(-6.87044407409259,23.6437291311068,
5.83636609328008));
#453921=CARTESIAN_POINT('Ctrl Pts',(-6.46537570391973,23.5722460604127,
4.73418498174874));
#453922=CARTESIAN_POINT('Ctrl Pts',(-5.31955101057096,23.5007629897185,
4.47734003862102));
#453923=CARTESIAN_POINT('Ctrl Pts',(-4.48275809327536,23.4292799190243,
5.30115015081045));
#453924=CARTESIAN_POINT('Ctrl Pts',(-4.72165647802514,23.3577968483301,
6.4508497069919));
#453925=CARTESIAN_POINT('Ctrl Pts',(-5.81736804855842,23.286313777636,6.87310399053069));
#453926=CARTESIAN_POINT('Ctrl Pts',(-6.76602226241636,23.2148307069418,
6.18104124059857));
#453927=CARTESIAN_POINT('Ctrl Pts',(-6.69846478576951,23.1433476362476,
5.00873590166637));
#453928=CARTESIAN_POINT('Ctrl Pts',(-5.67661126055156,23.0718645655534,
4.43020643614536));
#453929=CARTESIAN_POINT('Ctrl Pts',(-4.63662978245478,23.0003814948593,
4.97555543184771));
#453930=CARTESIAN_POINT('Ctrl Pts',(-4.53141556235811,22.928898424165,6.1450203373264));
#453931=CARTESIAN_POINT('Ctrl Pts',(-5.4572104595091,22.8574153534709,6.86739142284002));
#453932=CARTESIAN_POINT('Ctrl Pts',(-6.56611594115258,22.7859322827767,
6.48037563201499));
#453933=CARTESIAN_POINT('Ctrl Pts',(-6.8415750418855,22.7144492120825,5.33946716650399));
#453934=CARTESIAN_POINT('Ctrl Pts',(-6.0323875407531,22.6429661413883,4.48814850723257));
#453935=CARTESIAN_POINT('Ctrl Pts',(-4.87752780133468,22.5714830706942,
4.70999101793355));
#453936=CARTESIAN_POINT('Ctrl Pts',(-4.58641880376449,22.5238276902314,
5.4325862664886));
#453937=CARTESIAN_POINT('Ctrl Pts',(-4.62591736201901,22.5,5.7755760807344));
#453938=CARTESIAN_POINT('Ctrl Pts',(-4.92443355077908,25.6019615242271,
6.39006796800886));
#453939=CARTESIAN_POINT('Ctrl Pts',(-5.02053320993752,25.5925650294346,
6.48712194011206));
#453940=CARTESIAN_POINT('Ctrl Pts',(-5.13467106978717,25.5831685346421,
6.56580235206401));
#453941=CARTESIAN_POINT('Ctrl Pts',(-5.25993281439039,25.5737720398497,
6.617556583841));
#453942=CARTESIAN_POINT('Ctrl Pts',(-5.57757232935519,25.5499443496183,
6.74879528829216));
#453943=CARTESIAN_POINT('Ctrl Pts',(-5.96674190886751,25.5261166593869,
6.70689021711104));
#453944=CARTESIAN_POINT('Ctrl Pts',(-6.24916768313609,25.5022889691555,
6.51104990542648));
#453945=CARTESIAN_POINT('Ctrl Pts',(-6.53159345740467,25.4784612789241,
6.31520959374192));
#453946=CARTESIAN_POINT('Ctrl Pts',(-6.7072754264295,25.4546335886927,5.96543404155391));
#453947=CARTESIAN_POINT('Ctrl Pts',(-6.69573385251462,25.4308058984613,
5.62194684521822));
#453948=CARTESIAN_POINT('Ctrl Pts',(-6.68419227859974,25.4069782082299,
5.27845964888252));
#453949=CARTESIAN_POINT('Ctrl Pts',(-6.48542716174514,25.3831505179985,
4.94126080839914));
#453950=CARTESIAN_POINT('Ctrl Pts',(-6.19049196225386,25.3593228277671,
4.76482193949513));
#453951=CARTESIAN_POINT('Ctrl Pts',(-5.89555676276259,25.3354951375357,
4.58838307059113));
#453952=CARTESIAN_POINT('Ctrl Pts',(-5.50445148063464,25.3116674473043,
4.5727041732665));
#453953=CARTESIAN_POINT('Ctrl Pts',(-5.19633848255872,25.2878397570729,
4.72496603669335));
#453954=CARTESIAN_POINT('Ctrl Pts',(-4.8882254844828,25.2640120668416,4.87722790012021));
#453955=CARTESIAN_POINT('Ctrl Pts',(-4.66310477045891,25.2401843766102,
5.19743052429855));
#453956=CARTESIAN_POINT('Ctrl Pts',(-4.62410272688105,25.2163566863788,
5.53889211090842));
#453957=CARTESIAN_POINT('Ctrl Pts',(-4.58896793348097,25.1948916323282,
5.84649605160076));
#453958=CARTESIAN_POINT('Ctrl Pts',(-4.70487246063661,25.1734265782776,
6.17135209942283));
#453959=CARTESIAN_POINT('Ctrl Pts',(-4.92254817630007,25.1519615242271,
6.39198798715976));
#453960=CARTESIAN_POINT('Origin',(-5.65685387860011,26.,5.65685387860011));
#453961=CARTESIAN_POINT('Origin',(-5.65685387860012,26.993675081176,-5.65685387860011));
#453962=CARTESIAN_POINT('Ctrl Pts',(-6.57057130100612,25.868675081176,-4.74432962138981));
#453963=CARTESIAN_POINT('Ctrl Pts',(-6.60882993708832,25.8656848283261,
-4.78199706987976));
#453964=CARTESIAN_POINT('Ctrl Pts',(-6.92960341635463,25.8388668852448,
-5.14157728587623));
#453965=CARTESIAN_POINT('Ctrl Pts',(-7.09568592881682,25.7882212519322,
-6.16255878293893));
#453966=CARTESIAN_POINT('Ctrl Pts',(-6.01152748645437,25.716738181238,-7.13997732676548));
#453967=CARTESIAN_POINT('Ctrl Pts',(-4.60259286076204,25.6452551105438,
-6.7587374620765));
#453968=CARTESIAN_POINT('Ctrl Pts',(-4.15947051927595,25.5737720398497,
-5.36788602689621));
#453969=CARTESIAN_POINT('Ctrl Pts',(-5.08827462376231,25.5022889691555,
-4.24182426511434));
#453970=CARTESIAN_POINT('Ctrl Pts',(-6.13675122222029,25.450589982931,-4.36502559631504));
#453971=CARTESIAN_POINT('Ctrl Pts',(-6.51790892062316,25.4227186869378,
-4.69148744470697));
#453972=CARTESIAN_POINT('Ctrl Pts',(-6.56885365284802,25.418675081176,-4.74334636410459));
#453973=CARTESIAN_POINT('Ctrl Pts',(-6.56704169373441,25.906324918824,-4.74450601134849));
#453974=CARTESIAN_POINT('Ctrl Pts',(-6.7750658664325,25.8898945654199,-4.95573944791419));
#453975=CARTESIAN_POINT('Ctrl Pts',(-7.11639071403833,25.8496365217844,
-5.64807137163848));
#453976=CARTESIAN_POINT('Ctrl Pts',(-6.60321033464885,25.7855507879174,
-6.8522203629011));
#453977=CARTESIAN_POINT('Ctrl Pts',(-5.16550356767203,25.7140677172233,
-7.1004834147237));
#453978=CARTESIAN_POINT('Ctrl Pts',(-4.17707919799325,25.6425846465291,
-6.02596364157129));
#453979=CARTESIAN_POINT('Ctrl Pts',(-4.5448553014618,25.5711015758349,-4.61334644908231));
#453980=CARTESIAN_POINT('Ctrl Pts',(-5.74896333949311,25.5090149999332,
-4.21675923787011));
#453981=CARTESIAN_POINT('Ctrl Pts',(-6.3830054663296,25.4707561142629,-4.5629353888518));
#453982=CARTESIAN_POINT('Ctrl Pts',(-6.56829321884323,25.456324918824,-4.74640124271564));
#453983=CARTESIAN_POINT('Ctrl Pts',(-5.59475217632212,26.,-6.69274404704181));
#453984=CARTESIAN_POINT('Ctrl Pts',(-5.25011429538726,25.9761723097686,
-6.67208297724159));
#453985=CARTESIAN_POINT('Ctrl Pts',(-4.58904744425369,25.9285169293058,
-6.25991935236784));
#453986=CARTESIAN_POINT('Ctrl Pts',(-4.5711145089162,25.8570338586116,-5.08408179813166));
#453987=CARTESIAN_POINT('Ctrl Pts',(-5.55001366141289,25.7855507879175,
-4.43501771280631));
#453988=CARTESIAN_POINT('Ctrl Pts',(-6.62575617389683,25.7140677172233,
-4.90440858615388));
#453989=CARTESIAN_POINT('Ctrl Pts',(-6.81433291744693,25.6425846465291,
-6.06367191307887));
#453990=CARTESIAN_POINT('Ctrl Pts',(-5.94217367437589,25.5711015758349,
-6.84996345870369));
#453991=CARTESIAN_POINT('Ctrl Pts',(-4.80874583886255,25.4996185051408,
-6.54327224197424));
#453992=CARTESIAN_POINT('Ctrl Pts',(-4.45227280795,25.4281354344466,-5.42439156223909));
#453993=CARTESIAN_POINT('Ctrl Pts',(-5.19945610983427,25.3566523637524,
-4.51852288527076));
#453994=CARTESIAN_POINT('Ctrl Pts',(-6.36568271985868,25.2851692930583,
-4.65556044151951));
#453995=CARTESIAN_POINT('Ctrl Pts',(-6.88249940298929,25.213686222364,-5.70997789504277));
#453996=CARTESIAN_POINT('Ctrl Pts',(-6.27639179734011,25.1422031516699,
-6.71571945020394));
#453997=CARTESIAN_POINT('Ctrl Pts',(-5.10267450019954,25.0707200809757,
-6.7513451989237));
#453998=CARTESIAN_POINT('Ctrl Pts',(-4.43668748453226,24.9992370102815,
-5.78421192833873));
#453999=CARTESIAN_POINT('Ctrl Pts',(-4.88860074260098,24.9277539395873,
-4.7003955508837));
#454000=CARTESIAN_POINT('Ctrl Pts',(-6.04437662247731,24.8562708688931,
-4.49287282235238));
#454001=CARTESIAN_POINT('Ctrl Pts',(-6.84510966506768,24.784787798199,-5.35177365831405));
#454002=CARTESIAN_POINT('Ctrl Pts',(-6.55717903824976,24.7133047275048,
-6.49018471285718));
#454003=CARTESIAN_POINT('Ctrl Pts',(-5.44438294256282,24.6418216568106,
-6.86510957377));
#454004=CARTESIAN_POINT('Ctrl Pts',(-4.52624977050191,24.5703385861164,
-6.13304718756448));
#454005=CARTESIAN_POINT('Ctrl Pts',(-4.64396052187118,24.4988555154223,
-4.96470306042393));
#454006=CARTESIAN_POINT('Ctrl Pts',(-5.68967021074952,24.4273724447281,
-4.43049797487471));
#454007=CARTESIAN_POINT('Ctrl Pts',(-6.70531403099034,24.3558893740339,
-5.01986328076133));
#454008=CARTESIAN_POINT('Ctrl Pts',(-6.76037309820141,24.2844063033397,
-6.19283059794665));
#454009=CARTESIAN_POINT('Ctrl Pts',(-5.80440305573226,24.2129232326455,
-6.87474342740734));
#454010=CARTESIAN_POINT('Ctrl Pts',(-4.71325048867858,24.1414401619514,
-6.44084262551865));
#454011=CARTESIAN_POINT('Ctrl Pts',(-4.4866143522216,24.0699570912572,-5.28866213152759));
#454012=CARTESIAN_POINT('Ctrl Pts',(-5.3321355513588,23.9984740205631,-4.47381384511066));
#454013=CARTESIAN_POINT('Ctrl Pts',(-6.47515921171814,23.9269909498688,
-4.74285054378755));
#454014=CARTESIAN_POINT('Ctrl Pts',(-6.86846279219781,23.8555078791747,
-5.84928450947304));
#454015=CARTESIAN_POINT('Ctrl Pts',(-6.15170698086798,23.7840248084805,
-6.77941618151556));
#454016=CARTESIAN_POINT('Ctrl Pts',(-4.98157355760958,23.7125417377863,
-6.68107173221035));
#454017=CARTESIAN_POINT('Ctrl Pts',(-4.43012269359923,23.6410586670921,
-5.64435299191054));
#454018=CARTESIAN_POINT('Ctrl Pts',(-5.00258598787076,23.569575596398,-4.61908739135743));
#454019=CARTESIAN_POINT('Ctrl Pts',(-6.17448062637044,23.4980925257038,
-4.54460915448656));
#454020=CARTESIAN_POINT('Ctrl Pts',(-6.87213254456039,23.4266094550096,
-5.48915421344718));
#454021=CARTESIAN_POINT('Ctrl Pts',(-6.45636332421143,23.3551263843154,
-6.58734339945679));
#454022=CARTESIAN_POINT('Ctrl Pts',(-5.30809370313679,23.2836433136213,
-6.8330308949199));
#454023=CARTESIAN_POINT('Ctrl Pts',(-4.47935503415496,23.212160242927,-6.00112122066856));
#454024=CARTESIAN_POINT('Ctrl Pts',(-4.72942128924326,23.1406771722329,
-4.85379852261455));
#454025=CARTESIAN_POINT('Ctrl Pts',(-5.82919498069919,23.0691941015387,
-4.44222413342346));
#454026=CARTESIAN_POINT('Ctrl Pts',(-6.77105943752212,22.9977110308445,
-5.14347668616411));
#454027=CARTESIAN_POINT('Ctrl Pts',(-6.69212899367236,22.9262279601504,
-6.31507855179967));
#454028=CARTESIAN_POINT('Ctrl Pts',(-5.66464494341573,22.8547448894562,
-6.88362364563197));
#454029=CARTESIAN_POINT('Ctrl Pts',(-4.63011853598606,22.783261818762,-6.32821994284799));
#454030=CARTESIAN_POINT('Ctrl Pts',(-4.53608521045973,22.7117787480678,
-5.15771839492686));
#454031=CARTESIAN_POINT('Ctrl Pts',(-5.46925286619013,22.6402956773736,
-4.4445208236608));
#454032=CARTESIAN_POINT('Ctrl Pts',(-6.57357515235991,22.5688126066795,
-4.84204067651847));
#454033=CARTESIAN_POINT('Ctrl Pts',(-6.8394368280484,22.4973295359852,-5.98608844956735));
#454034=CARTESIAN_POINT('Ctrl Pts',(-6.01893246982621,22.4258464652911,
-6.82851835303725));
#454035=CARTESIAN_POINT('Ctrl Pts',(-5.25534692011694,22.3781910848283,
-6.67416374956871));
#454036=CARTESIAN_POINT('Ctrl Pts',(-4.99063298333217,22.3543633945969,
-6.45251384441992));
#454037=CARTESIAN_POINT('Ctrl Pts',(-5.58972040746333,26.0485455351344,
-6.77667668816906));
#454038=CARTESIAN_POINT('Ctrl Pts',(-5.21715836192049,26.024717844903,-6.75434156236399));
#454039=CARTESIAN_POINT('Ctrl Pts',(-4.50252879876621,25.9770624644402,
-6.30878252293169));
#454040=CARTESIAN_POINT('Ctrl Pts',(-4.48314285357121,25.905579393746,-5.03767313923882));
#454041=CARTESIAN_POINT('Ctrl Pts',(-5.54135696992153,25.8340963230518,
-4.33601886182374));
#454042=CARTESIAN_POINT('Ctrl Pts',(-6.70426114586779,25.7626132523576,
-4.84344196766208));
#454043=CARTESIAN_POINT('Ctrl Pts',(-6.90811725457023,25.6911301816635,
-6.09663420303223));
#454044=CARTESIAN_POINT('Ctrl Pts',(-5.96529161173539,25.6196471109693,
-6.94663474805762));
#454045=CARTESIAN_POINT('Ctrl Pts',(-4.74002817949571,25.5481640402751,
-6.61509398200833));
#454046=CARTESIAN_POINT('Ctrl Pts',(-4.35467204505865,25.4766809695809,
-5.40555638379146));
#454047=CARTESIAN_POINT('Ctrl Pts',(-5.16239561447694,25.4051978988867,
-4.42629001188529));
#454048=CARTESIAN_POINT('Ctrl Pts',(-6.42311533054124,25.3337148281926,
-4.57443098853514));
#454049=CARTESIAN_POINT('Ctrl Pts',(-6.98180690592904,25.2622317574984,
-5.71428225002476));
#454050=CARTESIAN_POINT('Ctrl Pts',(-6.32658964203687,25.1907486868042,
-6.80151366539291));
#454051=CARTESIAN_POINT('Ctrl Pts',(-5.05777230853438,25.11926561611,-6.84002597802966));
#454052=CARTESIAN_POINT('Ctrl Pts',(-4.33782392622387,25.0477825454159,
-5.79453107008661));
#454053=CARTESIAN_POINT('Ctrl Pts',(-4.82635329907546,24.9762994747217,
-4.62289884706407));
#454054=CARTESIAN_POINT('Ctrl Pts',(-6.07577551821105,24.9048164040275,
-4.39856166152736));
#454055=CARTESIAN_POINT('Ctrl Pts',(-6.941387677478,24.8333333333333,-5.32705463942152));
#454056=CARTESIAN_POINT('Ctrl Pts',(-6.63012757162216,24.7618502626391,
-6.55770505428216));
#454057=CARTESIAN_POINT('Ctrl Pts',(-5.42716755876279,24.690367191945,-6.96300807183685));
#454058=CARTESIAN_POINT('Ctrl Pts',(-4.4346429653087,24.6188841212508,-6.17163058503857));
#454059=CARTESIAN_POINT('Ctrl Pts',(-4.56189118942603,24.5474010505566,
-4.90862178076926));
#454060=CARTESIAN_POINT('Ctrl Pts',(-5.69232914266461,24.4759179798625,
-4.33113291369596));
#454061=CARTESIAN_POINT('Ctrl Pts',(-6.7902651507014,24.4044349091683,-4.96825133880203));
#454062=CARTESIAN_POINT('Ctrl Pts',(-6.8497853597109,24.3329518384741,-6.23625792548383));
#454063=CARTESIAN_POINT('Ctrl Pts',(-5.8163581765647,24.2614687677799,-6.97342250511928));
#454064=CARTESIAN_POINT('Ctrl Pts',(-4.63679535172919,24.1899856970857,
-6.50436504145381));
#454065=CARTESIAN_POINT('Ctrl Pts',(-4.39179610102783,24.1185026263916,
-5.25882952309621));
#454066=CARTESIAN_POINT('Ctrl Pts',(-5.30582536167066,24.0470195556974,
-4.37795843727392));
#454067=CARTESIAN_POINT('Ctrl Pts',(-6.54146211713177,23.9755364850032,
-4.66879374102308));
#454068=CARTESIAN_POINT('Ctrl Pts',(-6.96663298362319,23.904053414309,-5.86487613450724));
#454069=CARTESIAN_POINT('Ctrl Pts',(-6.19180228161384,23.8325703436148,
-6.87037140223681));
#454070=CARTESIAN_POINT('Ctrl Pts',(-4.92685920413014,23.7610872729207,
-6.76405862808224));
#454071=CARTESIAN_POINT('Ctrl Pts',(-4.33072722538547,23.6896042022265,
-5.64334011190815));
#454072=CARTESIAN_POINT('Ctrl Pts',(-4.94957415925549,23.6181211315323,
-4.53500272215098));
#454073=CARTESIAN_POINT('Ctrl Pts',(-6.21642115383373,23.5466380608381,
-4.45448991200439));
#454074=CARTESIAN_POINT('Ctrl Pts',(-6.9706000763964,23.475154990144,-5.47556640632124));
#454075=CARTESIAN_POINT('Ctrl Pts',(-6.52114329936776,23.4036719194498,
-6.66273598971973));
#454076=CARTESIAN_POINT('Ctrl Pts',(-5.27983553104633,23.3321888487556,
-6.92833022917403));
#454077=CARTESIAN_POINT('Ctrl Pts',(-4.38394859923605,23.2607057780614,
-6.02901536249358));
#454078=CARTESIAN_POINT('Ctrl Pts',(-4.6542763857934,23.1892227073672,-4.78873124130167));
#454079=CARTESIAN_POINT('Ctrl Pts',(-5.8431588586417,23.1177396366731,-4.34380918016856));
#454080=CARTESIAN_POINT('Ctrl Pts',(-6.86133755596364,23.0462565659789,
-5.1018804774459));
#454081=CARTESIAN_POINT('Ctrl Pts',(-6.77601180031397,22.9747734952847,
-6.36841097734037));
#454082=CARTESIAN_POINT('Ctrl Pts',(-5.66527621173653,22.9032904245905,
-6.98302223994139));
#454083=CARTESIAN_POINT('Ctrl Pts',(-4.54692766144197,22.8318073538963,
-6.3826171450343));
#454084=CARTESIAN_POINT('Ctrl Pts',(-4.4452753183732,22.7603242832022,-5.11727611571493));
#454085=CARTESIAN_POINT('Ctrl Pts',(-5.45405255931454,22.688841212508,-4.34629195893472));
#454086=CARTESIAN_POINT('Ctrl Pts',(-6.64785217518362,22.6173581418138,
-4.77602071980922));
#454087=CARTESIAN_POINT('Ctrl Pts',(-6.93525520080945,22.5458750711197,
-6.01276456633487));
#454088=CARTESIAN_POINT('Ctrl Pts',(-6.04826976192828,22.4743920004254,
-6.92345206015257));
#454089=CARTESIAN_POINT('Ctrl Pts',(-5.22281495825156,22.4267366199627,
-6.75659092854625));
#454090=CARTESIAN_POINT('Ctrl Pts',(-4.93665266667552,22.4029089297313,
-6.5169819168131));
#454091=CARTESIAN_POINT('Ctrl Pts',(-5.58468863860454,26.0970910702687,
-6.86060932929632));
#454092=CARTESIAN_POINT('Ctrl Pts',(-5.18420242845371,26.0732633800373,
-6.83660014748639));
#454093=CARTESIAN_POINT('Ctrl Pts',(-4.41601015327874,26.0256079995746,
-6.35764569349554));
#454094=CARTESIAN_POINT('Ctrl Pts',(-4.39517119822623,25.9541249288803,
-4.99126448034597));
#454095=CARTESIAN_POINT('Ctrl Pts',(-5.53270027843018,25.8826418581862,
-4.23702001084117));
#454096=CARTESIAN_POINT('Ctrl Pts',(-6.78276611783875,25.811158787492,-4.7824753491703));
#454097=CARTESIAN_POINT('Ctrl Pts',(-7.00190159169353,25.7396757167979,
-6.12959649298558));
#454098=CARTESIAN_POINT('Ctrl Pts',(-5.98840954909488,25.6681926461036,
-7.04330603741155));
#454099=CARTESIAN_POINT('Ctrl Pts',(-4.67131052012888,25.5967095754095,
-6.68691572204242));
#454100=CARTESIAN_POINT('Ctrl Pts',(-4.2570712821673,25.5252265047153,-5.38672120534383));
#454101=CARTESIAN_POINT('Ctrl Pts',(-5.12533511911963,25.4537434340211,
-4.33405713849982));
#454102=CARTESIAN_POINT('Ctrl Pts',(-6.48054794122378,25.382260363327,-4.49330153555078));
#454103=CARTESIAN_POINT('Ctrl Pts',(-7.0811144088688,25.3107772926328,-5.71858660500674));
#454104=CARTESIAN_POINT('Ctrl Pts',(-6.37678748673361,25.2392942219386,
-6.88730788058188));
#454105=CARTESIAN_POINT('Ctrl Pts',(-5.01287011686923,25.1678111512444,
-6.92870675713562));
#454106=CARTESIAN_POINT('Ctrl Pts',(-4.23896036791547,25.0963280805502,
-5.80485021183448));
#454107=CARTESIAN_POINT('Ctrl Pts',(-4.76410585554996,25.0248450098561,
-4.54540214324444));
#454108=CARTESIAN_POINT('Ctrl Pts',(-6.10717441394478,24.9533619391619,
-4.30425050070234));
#454109=CARTESIAN_POINT('Ctrl Pts',(-7.03766568988833,24.8818788684677,
-5.302335620529));
#454110=CARTESIAN_POINT('Ctrl Pts',(-6.70307610499455,24.8103957977735,
-6.62522539570715));
#454111=CARTESIAN_POINT('Ctrl Pts',(-5.40995217496277,24.7389127270793,
-7.0609065699037));
#454112=CARTESIAN_POINT('Ctrl Pts',(-4.34303616011549,24.6674296563851,
-6.21021398251267));
#454113=CARTESIAN_POINT('Ctrl Pts',(-4.47982185698087,24.595946585691,-4.85254050111458));
#454114=CARTESIAN_POINT('Ctrl Pts',(-5.69498807457972,24.5244635149968,
-4.23176785251722));
#454115=CARTESIAN_POINT('Ctrl Pts',(-6.87521627041245,24.4529804443027,
-4.91663939684271));
#454116=CARTESIAN_POINT('Ctrl Pts',(-6.93919762122039,24.3814973736084,
-6.27968525302103));
#454117=CARTESIAN_POINT('Ctrl Pts',(-5.82831329739714,24.3100143029143,
-7.07210158283119));
#454118=CARTESIAN_POINT('Ctrl Pts',(-4.5603402147798,24.2385312322201,-6.567887457389));
#454119=CARTESIAN_POINT('Ctrl Pts',(-4.29697784983407,24.1670481615259,
-5.22899691466481));
#454120=CARTESIAN_POINT('Ctrl Pts',(-5.27951517198252,24.0955650908318,
-4.28210302943719));
#454121=CARTESIAN_POINT('Ctrl Pts',(-6.60776502254541,24.0240820201375,
-4.59473693825861));
#454122=CARTESIAN_POINT('Ctrl Pts',(-7.06480317504856,23.9525989494434,
-5.88046775954143));
#454123=CARTESIAN_POINT('Ctrl Pts',(-6.2318975823597,23.8811158787492,-6.96132662295805));
#454124=CARTESIAN_POINT('Ctrl Pts',(-4.87214485065071,23.809632808055,-6.84704552395415));
#454125=CARTESIAN_POINT('Ctrl Pts',(-4.23133175717171,23.7381497373609,
-5.64232723190575));
#454126=CARTESIAN_POINT('Ctrl Pts',(-4.89656233064023,23.6666666666667,
-4.45091805294454));
#454127=CARTESIAN_POINT('Ctrl Pts',(-6.258361681297,23.5951835959725,-4.3643706695222));
#454128=CARTESIAN_POINT('Ctrl Pts',(-7.06906760823243,23.5237005252783,
-5.4619785991953));
#454129=CARTESIAN_POINT('Ctrl Pts',(-6.58592327452408,23.4522174545842,
-6.73812857998267));
#454130=CARTESIAN_POINT('Ctrl Pts',(-5.25157735895588,23.3807343838899,
-7.02362956342815));
#454131=CARTESIAN_POINT('Ctrl Pts',(-4.28854216431714,23.3092513131958,
-6.05690950431861));
#454132=CARTESIAN_POINT('Ctrl Pts',(-4.57913148234355,23.2377682425016,
-4.72366395998878));
#454133=CARTESIAN_POINT('Ctrl Pts',(-5.85712273658419,23.1662851718074,
-4.24539422691366));
#454134=CARTESIAN_POINT('Ctrl Pts',(-6.95161567440516,23.0948021011132,
-5.06028426872769));
#454135=CARTESIAN_POINT('Ctrl Pts',(-6.85989460695557,23.0233190304191,
-6.42174340288106));
#454136=CARTESIAN_POINT('Ctrl Pts',(-5.66590748005734,22.9518359597249,
-7.08242083425081));
#454137=CARTESIAN_POINT('Ctrl Pts',(-4.46373678689788,22.8803528890307,
-6.4370143472206));
#454138=CARTESIAN_POINT('Ctrl Pts',(-4.35446542628666,22.8088698183366,
-5.07683383650299));
#454139=CARTESIAN_POINT('Ctrl Pts',(-5.43885225243895,22.7373867476423,
-4.24806309420865));
#454140=CARTESIAN_POINT('Ctrl Pts',(-6.72212919800733,22.6659036769482,
-4.71000076309996));
#454141=CARTESIAN_POINT('Ctrl Pts',(-7.03107357357049,22.594420606254,-6.03944068310239));
#454142=CARTESIAN_POINT('Ctrl Pts',(-6.07760705403035,22.5229375355598,
-7.01838576726789));
#454143=CARTESIAN_POINT('Ctrl Pts',(-5.19028299638619,22.475282155097,-6.83901810752379));
#454144=CARTESIAN_POINT('Ctrl Pts',(-4.88267235001886,22.4514544648656,
-6.58144998920627));
#454145=CARTESIAN_POINT('Ctrl Pts',(-5.57965686974575,26.1456366054031,
-6.94454197042357));
#454146=CARTESIAN_POINT('Ctrl Pts',(-5.15124649498693,26.1218089151717,
-6.91885873260879));
#454147=CARTESIAN_POINT('Ctrl Pts',(-4.32949150779126,26.0741535347089,
-6.4065088640594));
#454148=CARTESIAN_POINT('Ctrl Pts',(-4.30719954288124,26.0026704640147,
-4.94485582145311));
#454149=CARTESIAN_POINT('Ctrl Pts',(-5.52404358693881,25.9311873933206,
-4.1380211598586));
#454150=CARTESIAN_POINT('Ctrl Pts',(-6.86127108980971,25.8597043226263,
-4.7215087306785));
#454151=CARTESIAN_POINT('Ctrl Pts',(-7.09568592881682,25.7882212519322,
-6.16255878293893));
#454152=CARTESIAN_POINT('Ctrl Pts',(-6.01152748645437,25.716738181238,-7.13997732676548));
#454153=CARTESIAN_POINT('Ctrl Pts',(-4.60259286076204,25.6452551105438,
-6.7587374620765));
#454154=CARTESIAN_POINT('Ctrl Pts',(-4.15947051927595,25.5737720398497,
-5.36788602689621));
#454155=CARTESIAN_POINT('Ctrl Pts',(-5.08827462376231,25.5022889691555,
-4.24182426511434));
#454156=CARTESIAN_POINT('Ctrl Pts',(-6.53798055190634,25.4308058984613,
-4.41217208256641));
#454157=CARTESIAN_POINT('Ctrl Pts',(-7.18042191180854,25.3593228277671,
-5.72289095998872));
#454158=CARTESIAN_POINT('Ctrl Pts',(-6.42698533143036,25.287839757073,-6.97310209577086));
#454159=CARTESIAN_POINT('Ctrl Pts',(-4.96796792520408,25.2163566863788,
-7.01738753624157));
#454160=CARTESIAN_POINT('Ctrl Pts',(-4.14009680960707,25.1448736156846,
-5.81516935358236));
#454161=CARTESIAN_POINT('Ctrl Pts',(-4.70185841202445,25.0733905449904,
-4.46790543942481));
#454162=CARTESIAN_POINT('Ctrl Pts',(-6.1385733096785,25.0019074742962,-4.20993933987732));
#454163=CARTESIAN_POINT('Ctrl Pts',(-7.13394370229866,24.930424403602,-5.27761660163647));
#454164=CARTESIAN_POINT('Ctrl Pts',(-6.77602463836695,24.8589413329079,
-6.69274573713214));
#454165=CARTESIAN_POINT('Ctrl Pts',(-5.39273679116276,24.7874582622137,
-7.15880506797054));
#454166=CARTESIAN_POINT('Ctrl Pts',(-4.25142935492228,24.7159751915195,
-6.24879737998679));
#454167=CARTESIAN_POINT('Ctrl Pts',(-4.39775252453572,24.6444921208253,
-4.79645922145989));
#454168=CARTESIAN_POINT('Ctrl Pts',(-5.69764700649481,24.5730090501312,
-4.13240279133847));
#454169=CARTESIAN_POINT('Ctrl Pts',(-6.9601673901235,24.501525979437,-4.86502745488341));
#454170=CARTESIAN_POINT('Ctrl Pts',(-7.02860988272989,24.4300429087428,
-6.32311258055821));
#454171=CARTESIAN_POINT('Ctrl Pts',(-5.84026841822957,24.3585598380486,
-7.17078066054311));
#454172=CARTESIAN_POINT('Ctrl Pts',(-4.4838850778304,24.2870767673545,-6.63140987332417));
#454173=CARTESIAN_POINT('Ctrl Pts',(-4.2021595986403,24.2155936966603,-5.19916430623342));
#454174=CARTESIAN_POINT('Ctrl Pts',(-5.25320498229437,24.1441106259661,
-4.18624762160045));
#454175=CARTESIAN_POINT('Ctrl Pts',(-6.67406792795906,24.0726275552719,
-4.52068013549415));
#454176=CARTESIAN_POINT('Ctrl Pts',(-7.16297336647392,24.0011444845777,
-5.89605938457563));
#454177=CARTESIAN_POINT('Ctrl Pts',(-6.27199288310558,23.9296614138836,
-7.0522818436793));
#454178=CARTESIAN_POINT('Ctrl Pts',(-4.81743049717126,23.8581783431894,
-6.93003241982605));
#454179=CARTESIAN_POINT('Ctrl Pts',(-4.13193628895796,23.7866952724952,
-5.64131435190337));
#454180=CARTESIAN_POINT('Ctrl Pts',(-4.84355050202496,23.715212201801,-4.3668333837381));
#454181=CARTESIAN_POINT('Ctrl Pts',(-6.30030220876029,23.6437291311069,
-4.27425142704003));
#454182=CARTESIAN_POINT('Ctrl Pts',(-7.16753514006844,23.5722460604127,
-5.44839079206936));
#454183=CARTESIAN_POINT('Ctrl Pts',(-6.65070324968042,23.5007629897185,
-6.81352117024561));
#454184=CARTESIAN_POINT('Ctrl Pts',(-5.22331918686542,23.4292799190243,
-7.11892889768229));
#454185=CARTESIAN_POINT('Ctrl Pts',(-4.19313572939823,23.3577968483302,
-6.08480364614364));
#454186=CARTESIAN_POINT('Ctrl Pts',(-4.50398657889369,23.2863137776359,
-4.65859667867589));
#454187=CARTESIAN_POINT('Ctrl Pts',(-5.8710866145267,23.2148307069418,-4.14697927365876));
#454188=CARTESIAN_POINT('Ctrl Pts',(-7.04189379284668,23.1433476362476,
-5.01868806000948));
#454189=CARTESIAN_POINT('Ctrl Pts',(-6.94377741359719,23.0718645655535,
-6.47507582842176));
#454190=CARTESIAN_POINT('Ctrl Pts',(-5.66653874837813,23.0003814948592,
-7.18181942856023));
#454191=CARTESIAN_POINT('Ctrl Pts',(-4.38054591235379,22.9288984241651,
-6.49141154940691));
#454192=CARTESIAN_POINT('Ctrl Pts',(-4.26365553420012,22.8574153534709,
-5.03639155729104));
#454193=CARTESIAN_POINT('Ctrl Pts',(-5.42365194556336,22.7859322827767,
-4.14983422948258));
#454194=CARTESIAN_POINT('Ctrl Pts',(-6.79640622083105,22.7144492120825,
-4.6439808063907));
#454195=CARTESIAN_POINT('Ctrl Pts',(-7.12689194633153,22.6429661413884,
-6.06611679986992));
#454196=CARTESIAN_POINT('Ctrl Pts',(-6.10694434613243,22.5714830706942,
-7.11331947438321));
#454197=CARTESIAN_POINT('Ctrl Pts',(-5.15775103452081,22.5238276902314,
-6.92144528650133));
#454198=CARTESIAN_POINT('Ctrl Pts',(-4.8286920333622,22.5,-6.64591806159944));
#454199=CARTESIAN_POINT('Ctrl Pts',(-6.39051881327128,25.2730384757729,
-4.92197603118329));
#454200=CARTESIAN_POINT('Ctrl Pts',(-6.34953594825859,25.2770820815347,
-4.8802577415671));
#454201=CARTESIAN_POINT('Ctrl Pts',(-6.3050503566324,25.2811256872965,-4.84215579969382));
#454202=CARTESIAN_POINT('Ctrl Pts',(-6.25744773204304,25.2851692930582,
-4.80845709106527));
#454203=CARTESIAN_POINT('Ctrl Pts',(-5.97694051651721,25.3089969832896,
-4.60988125610326));
#454204=CARTESIAN_POINT('Ctrl Pts',(-5.58819831317574,25.332824673521,-4.56420207068701));
#454205=CARTESIAN_POINT('Ctrl Pts',(-5.26929666119096,25.3566523637524,
-4.69234059080694));
#454206=CARTESIAN_POINT('Ctrl Pts',(-4.95039500920618,25.3804800539838,
-4.82047911092687));
#454207=CARTESIAN_POINT('Ctrl Pts',(-4.70133390857809,25.4043077442152,
-5.12243533658298));
#454208=CARTESIAN_POINT('Ctrl Pts',(-4.6362155300828,25.4281354344466,-5.45989356270023));
#454209=CARTESIAN_POINT('Ctrl Pts',(-4.57109715158752,25.451963124678,-5.79735178881747));
#454210=CARTESIAN_POINT('Ctrl Pts',(-4.68992149522503,25.4757908149094,
-6.17031201539585));
#454211=CARTESIAN_POINT('Ctrl Pts',(-4.93823830629602,25.4996185051408,
-6.40790733147329));
#454212=CARTESIAN_POINT('Ctrl Pts',(-5.186555117367,25.5234461953722,-6.64550264755072));
#454213=CARTESIAN_POINT('Ctrl Pts',(-5.56436439587145,25.5472738856035,
-6.74773305312721));
#454214=CARTESIAN_POINT('Ctrl Pts',(-5.89862890896884,25.5711015758349,
-6.66779966497798));
#454215=CARTESIAN_POINT('Ctrl Pts',(-6.23289342206624,25.5949292660663,
-6.58786627682875));
#454216=CARTESIAN_POINT('Ctrl Pts',(-6.52361316975658,25.6187569562977,
-6.32576909495381));
#454217=CARTESIAN_POINT('Ctrl Pts',(-6.63754358634341,25.6425846465291,
-6.00150994952884));
#454218=CARTESIAN_POINT('Ctrl Pts',(-6.75147400293023,25.6664123367605,
-5.67725080410387));
#454219=CARTESIAN_POINT('Ctrl Pts',(-6.68861508841353,25.6902400269919,
-5.29082969512888));
#454220=CARTESIAN_POINT('Ctrl Pts',(-6.47789521240786,25.7140677172233,
-5.01938732841678));
#454221=CARTESIAN_POINT('Ctrl Pts',(-6.45145094929911,25.7170579700732,
-4.98532270432787));
#454222=CARTESIAN_POINT('Ctrl Pts',(-6.42267802952734,25.720048222923,-4.95306887608107));
#454223=CARTESIAN_POINT('Ctrl Pts',(-6.39190058798136,25.7230384757729,
-4.92276701974739));
#454224=CARTESIAN_POINT('Ctrl Pts',(-5.01302286563431,26.,-4.53900700771688));
#454225=CARTESIAN_POINT('Ctrl Pts',(-5.38492752167559,25.9761723097686,
-4.32480615636363));
#454226=CARTESIAN_POINT('Ctrl Pts',(-6.35301914505848,25.9285169293058,
-4.30067277954968));
#454227=CARTESIAN_POINT('Ctrl Pts',(-7.1756264891545,25.8570338586117,-5.50907794609547));
#454228=CARTESIAN_POINT('Ctrl Pts',(-6.60321033464885,25.7855507879174,
-6.8522203629011));
#454229=CARTESIAN_POINT('Ctrl Pts',(-5.16550356767203,25.7140677172233,
-7.1004834147237));
#454230=CARTESIAN_POINT('Ctrl Pts',(-4.17707919799325,25.6425846465291,
-6.02596364157129));
#454231=CARTESIAN_POINT('Ctrl Pts',(-4.5448553014618,25.5711015758349,-4.61334644908231));
#454232=CARTESIAN_POINT('Ctrl Pts',(-5.93119910857215,25.4996185051408,
-4.15673773385264));
#454233=CARTESIAN_POINT('Ctrl Pts',(-7.0663089114369,25.4281354344466,-5.07453447980768));
#454234=CARTESIAN_POINT('Ctrl Pts',(-6.9100356033464,25.3566523637524,-6.5258341885166));
#454235=CARTESIAN_POINT('Ctrl Pts',(-5.60564496305001,25.2851692930582,
-7.18099123031483));
#454236=CARTESIAN_POINT('Ctrl Pts',(-4.34815567114858,25.213686222364,-6.43975200870338));
#454237=CARTESIAN_POINT('Ctrl Pts',(-4.2896855842815,25.1422031516699,-4.98123363545819));
#454238=CARTESIAN_POINT('Ctrl Pts',(-5.48379221455872,25.0707200809757,
-4.14170854437417));
#454239=CARTESIAN_POINT('Ctrl Pts',(-6.83645762028281,24.9992370102815,
-4.69033908735646));
#454240=CARTESIAN_POINT('Ctrl Pts',(-7.10838527255516,24.9277539395874,
-6.12447699388038));
#454241=CARTESIAN_POINT('Ctrl Pts',(-6.05044038944422,24.8562708688931,
-7.13018513270865));
#454242=CARTESIAN_POINT('Ctrl Pts',(-4.63189669239788,24.784787798199,-6.78604742232836));
#454243=CARTESIAN_POINT('Ctrl Pts',(-4.15240479236239,24.7133047275048,
-5.40735816264999));
#454244=CARTESIAN_POINT('Ctrl Pts',(-5.0512683537124,24.6418216568106,-4.25725342975252));
#454245=CARTESIAN_POINT('Ctrl Pts',(-6.50496106867921,24.5703385861164,
-4.38944335790391));
#454246=CARTESIAN_POINT('Ctrl Pts',(-7.18162963832198,24.4988555154223,
-5.68281734635597));
#454247=CARTESIAN_POINT('Ctrl Pts',(-6.46131966662841,24.4273724447281,
-6.95240396480877));
#454248=CARTESIAN_POINT('Ctrl Pts',(-5.00396921476326,24.3558893740339,
-7.03502543671246));
#454249=CARTESIAN_POINT('Ctrl Pts',(-4.14478270244581,24.2844063033397,
-5.85498510857852));
#454250=CARTESIAN_POINT('Ctrl Pts',(-4.67093497503137,24.2129232326456,
-4.49341967622111));
#454251=CARTESIAN_POINT('Ctrl Pts',(-6.10037256921808,24.1414401619514,
-4.19777663638434));
#454252=CARTESIAN_POINT('Ctrl Pts',(-7.12346444664167,24.0699570912572,
-5.23892007073304));
#454253=CARTESIAN_POINT('Ctrl Pts',(-6.80286792203874,23.998474020563,-6.662968703113));
#454254=CARTESIAN_POINT('Ctrl Pts',(-5.43230911237055,23.9269909498688,
-7.16522879152533));
#454255=CARTESIAN_POINT('Ctrl Pts',(-4.26747512907024,23.8555078791747,
-6.2855365564656));
#454256=CARTESIAN_POINT('Ctrl Pts',(-4.37557081254884,23.7840248084805,
-4.82985391579145));
#454257=CARTESIAN_POINT('Ctrl Pts',(-5.6575604101698,23.7125417377863,-4.13185724083954));
#454258=CARTESIAN_POINT('Ctrl Pts',(-6.93890266242659,23.6410586670921,
-4.83104150205928));
#454259=CARTESIAN_POINT('Ctrl Pts',(-7.04564953674368,23.569575596398,-6.28682364983267));
#454260=CARTESIAN_POINT('Ctrl Pts',(-5.88000083782647,23.4980925257038,
-7.16543624640093));
#454261=CARTESIAN_POINT('Ctrl Pts',(-4.50990820099157,23.4266094550096,
-6.66190630419616));
#454262=CARTESIAN_POINT('Ctrl Pts',(-4.19063094092434,23.3551263843154,
-5.23756146736659));
#454263=CARTESIAN_POINT('Ctrl Pts',(-5.21468783779197,23.2836433136212,
-4.19736598356861));
#454264=CARTESIAN_POINT('Ctrl Pts',(-6.64384941569999,23.2121602429271,
-4.49433434427903));
#454265=CARTESIAN_POINT('Ctrl Pts',(-7.16874271925581,23.1406771722328,
-5.85638486317849));
#454266=CARTESIAN_POINT('Ctrl Pts',(-6.3084575374563,23.0691941015387,-7.03563221165043));
#454267=CARTESIAN_POINT('Ctrl Pts',(-4.85119529970874,22.9977110308445,
-6.95165327175697));
#454268=CARTESIAN_POINT('Ctrl Pts',(-4.13204038713624,22.9262279601503,
-5.68141376558385));
#454269=CARTESIAN_POINT('Ctrl Pts',(-4.80994952176022,22.8547448894562,
-4.38863987327371));
#454270=CARTESIAN_POINT('Ctrl Pts',(-6.26368089065207,22.783261818762,-4.25785081625157));
#454271=CARTESIAN_POINT('Ctrl Pts',(-7.16164157512573,22.7117787480678,
-5.40868234342555));
#454272=CARTESIAN_POINT('Ctrl Pts',(-6.68055232418451,22.6402956773736,
-6.78713386963136));
#454273=CARTESIAN_POINT('Ctrl Pts',(-5.26231872215201,22.5688126066795,
-7.12954990426926));
#454274=CARTESIAN_POINT('Ctrl Pts',(-4.20406666678213,22.4973295359853,
-6.1236699944058));
#454275=CARTESIAN_POINT('Ctrl Pts',(-4.4798333146301,22.4258464652911,-4.68809392709695));
#454276=CARTESIAN_POINT('Ctrl Pts',(-5.37807265034296,22.3781910848283,
-4.32622391325397));
#454277=CARTESIAN_POINT('Ctrl Pts',(-5.80443435631943,22.3543633945969,
-4.37532354240196));
#454278=CARTESIAN_POINT('Ctrl Pts',(-5.05498833669907,26.0485455351344,
-4.61186924884874));
#454279=CARTESIAN_POINT('Ctrl Pts',(-5.40265192052164,26.024717844903,-4.41163019717349));
#454280=CARTESIAN_POINT('Ctrl Pts',(-6.30764248137266,25.9770624644402,
-4.38906985506272));
#454281=CARTESIAN_POINT('Ctrl Pts',(-7.07663155607638,25.905579393746,-5.51871011120511));
#454282=CARTESIAN_POINT('Ctrl Pts',(-6.54152598941931,25.8340963230518,
-6.77430532526158));
#454283=CARTESIAN_POINT('Ctrl Pts',(-5.1975302126156,25.7626132523576,-7.00638637325414));
#454284=CARTESIAN_POINT('Ctrl Pts',(-4.27353221173565,25.6911301816635,
-6.00190474293836));
#454285=CARTESIAN_POINT('Ctrl Pts',(-4.61733634566933,25.6196471109693,
-4.68136318011483));
#454286=CARTESIAN_POINT('Ctrl Pts',(-5.91331704545576,25.5481640402751,
-4.25451662209878));
#454287=CARTESIAN_POINT('Ctrl Pts',(-6.97443939411568,25.4766809695809,
-5.11249056981941));
#454288=CARTESIAN_POINT('Ctrl Pts',(-6.82835211754092,25.4051978988868,
-6.46919328847102));
#454289=CARTESIAN_POINT('Ctrl Pts',(-5.60898280515531,25.3337148281926,
-7.08164661869466));
#454290=CARTESIAN_POINT('Ctrl Pts',(-4.43345777007097,25.2622317574984,
-6.38872202076577));
#454291=CARTESIAN_POINT('Ctrl Pts',(-4.37879881483497,25.1907486868042,
-5.02527115647435));
#454292=CARTESIAN_POINT('Ctrl Pts',(-5.49507252586477,25.1192656161101,
-4.24046704839444));
#454293=CARTESIAN_POINT('Ctrl Pts',(-6.75957001205557,25.0477825454159,
-4.75333737058418));
#454294=CARTESIAN_POINT('Ctrl Pts',(-7.01377318104995,24.9762994747217,
-6.09399690839473));
#454295=CARTESIAN_POINT('Ctrl Pts',(-6.0247860748808,24.9048164040275,-7.03415210716631));
#454296=CARTESIAN_POINT('Ctrl Pts',(-4.69870430227373,24.8333333333333,
-6.71244559509181));
#454297=CARTESIAN_POINT('Ctrl Pts',(-4.25046610554157,24.7618502626392,
-5.42362051261083));
#454298=CARTESIAN_POINT('Ctrl Pts',(-5.09074095026355,24.690367191945,-4.34848061663153));
#454299=CARTESIAN_POINT('Ctrl Pts',(-6.44968069692276,24.6188841212508,
-4.47205428913018));
#454300=CARTESIAN_POINT('Ctrl Pts',(-7.08224341470705,24.5474010505566,
-5.68112502471735));
#454301=CARTESIAN_POINT('Ctrl Pts',(-6.40888387979891,24.4759179798625,
-6.86795887198031));
#454302=CARTESIAN_POINT('Ctrl Pts',(-5.04652481074592,24.4044349091682,
-6.94519500375798));
#454303=CARTESIAN_POINT('Ctrl Pts',(-4.24334083014217,24.3329518384741,
-5.84207074093974));
#454304=CARTESIAN_POINT('Ctrl Pts',(-4.73519803534797,24.2614687677799,
-4.56925333967074));
#454305=CARTESIAN_POINT('Ctrl Pts',(-6.07146363130893,24.1899856970857,
-4.29288057290861));
#454306=CARTESIAN_POINT('Ctrl Pts',(-7.02786948132165,24.1185026263916,
-5.2661613635068));
#454307=CARTESIAN_POINT('Ctrl Pts',(-6.72816971985337,24.0470195556973,
-6.59738925492608));
#454308=CARTESIAN_POINT('Ctrl Pts',(-5.44694513750787,23.9755364850032,
-7.0669115895136));
#454309=CARTESIAN_POINT('Ctrl Pts',(-4.35803605660742,23.904053414309,-6.24455846719129));
#454310=CARTESIAN_POINT('Ctrl Pts',(-4.45908596846911,23.8325703436148,
-4.8837584999306));
#454311=CARTESIAN_POINT('Ctrl Pts',(-5.65751435782136,23.7610872729207,
-4.2312578614791));
#454312=CARTESIAN_POINT('Ctrl Pts',(-6.85533759634902,23.6896042022265,
-4.88486867828213));
#454313=CARTESIAN_POINT('Ctrl Pts',(-6.95512661561532,23.6181211315323,
-6.24576166668191));
#454314=CARTESIAN_POINT('Ctrl Pts',(-5.86545592297769,23.5466380608381,
-7.06710552229815));
#454315=CARTESIAN_POINT('Ctrl Pts',(-4.58466712791061,23.475154990144,-6.59639610410402));
#454316=CARTESIAN_POINT('Ctrl Pts',(-4.28620064015658,23.4036719194498,
-5.26489131510138));
#454317=CARTESIAN_POINT('Ctrl Pts',(-5.24350860879812,23.3321888487556,
-4.2924966868042));
#454318=CARTESIAN_POINT('Ctrl Pts',(-6.57951617946397,23.2607057780614,
-4.57010838886106));
#454319=CARTESIAN_POINT('Ctrl Pts',(-7.07019647634743,23.1892227073672,
-5.84337925830513));
#454320=CARTESIAN_POINT('Ctrl Pts',(-6.26598543850373,23.1177396366731,
-6.94576222857241));
#454321=CARTESIAN_POINT('Ctrl Pts',(-4.90370883369462,23.0462565659789,
-6.86725710976114));
#454322=CARTESIAN_POINT('Ctrl Pts',(-4.23142907013928,22.9747734952847,
-5.67981293057309));
#454323=CARTESIAN_POINT('Ctrl Pts',(-4.86515149178938,22.9032904245905,
-4.47130317633407));
#454324=CARTESIAN_POINT('Ctrl Pts',(-6.22412737287685,22.8318073538963,
-4.34903906495375));
#454325=CARTESIAN_POINT('Ctrl Pts',(-7.06355819103049,22.7603242832022,
-5.42485838212006));
#454326=CARTESIAN_POINT('Ctrl Pts',(-6.613826760128,22.688841212508,-6.7134612268051));
#454327=CARTESIAN_POINT('Ctrl Pts',(-5.28803487026933,22.6173581418138,
-7.03355828347467));
#454328=CARTESIAN_POINT('Ctrl Pts',(-4.29876061359894,22.5458750711196,
-6.0932425098549));
#454329=CARTESIAN_POINT('Ctrl Pts',(-4.55655254906459,22.4743920004255,
-4.75123855184285));
#454330=CARTESIAN_POINT('Ctrl Pts',(-5.39624385572484,22.4267366199627,
-4.41295554342414));
#454331=CARTESIAN_POINT('Ctrl Pts',(-5.79481493112442,22.4029089297313,
-4.45885481560764));
#454332=CARTESIAN_POINT('Ctrl Pts',(-5.09695380776383,26.0970910702687,
-4.6847314899806));
#454333=CARTESIAN_POINT('Ctrl Pts',(-5.42037631936769,26.0732633800373,
-4.49845423798335));
#454334=CARTESIAN_POINT('Ctrl Pts',(-6.26226581768684,26.0256079995745,
-4.47746693057576));
#454335=CARTESIAN_POINT('Ctrl Pts',(-6.97763662299825,25.9541249288804,
-5.52834227631475));
#454336=CARTESIAN_POINT('Ctrl Pts',(-6.47984164418979,25.8826418581862,
-6.69639028762207));
#454337=CARTESIAN_POINT('Ctrl Pts',(-5.22955685755916,25.811158787492,-6.91228933178459));
#454338=CARTESIAN_POINT('Ctrl Pts',(-4.36998522547805,25.7396757167978,
-5.97784584430541));
#454339=CARTESIAN_POINT('Ctrl Pts',(-4.68981738987686,25.6681926461037,
-4.74937991114735));
#454340=CARTESIAN_POINT('Ctrl Pts',(-5.89543498233936,25.5967095754095,
-4.35229551034492));
#454341=CARTESIAN_POINT('Ctrl Pts',(-6.88256987679449,25.5252265047153,
-5.15044665983114));
#454342=CARTESIAN_POINT('Ctrl Pts',(-6.74666863173542,25.4537434340211,
-6.41255238842542));
#454343=CARTESIAN_POINT('Ctrl Pts',(-5.61232064726062,25.3822603633269,
-6.9823020070745));
#454344=CARTESIAN_POINT('Ctrl Pts',(-4.51875986899335,25.3107772926328,
-6.33769203282816));
#454345=CARTESIAN_POINT('Ctrl Pts',(-4.46791204538843,25.2392942219386,
-5.06930867749052));
#454346=CARTESIAN_POINT('Ctrl Pts',(-5.50635283717082,25.1678111512444,
-4.33922555241473));
#454347=CARTESIAN_POINT('Ctrl Pts',(-6.68268240382832,25.0963280805502,
-4.81633565381187));
#454348=CARTESIAN_POINT('Ctrl Pts',(-6.91916108954474,25.0248450098561,
-6.06351682290909));
#454349=CARTESIAN_POINT('Ctrl Pts',(-5.99913176031739,24.9533619391618,
-6.93811908162396));
#454350=CARTESIAN_POINT('Ctrl Pts',(-4.76551191214956,24.8818788684677,
-6.63884376785526));
#454351=CARTESIAN_POINT('Ctrl Pts',(-4.34852741872077,24.8103957977735,
-5.43988286257166));
#454352=CARTESIAN_POINT('Ctrl Pts',(-5.13021354681468,24.7389127270794,
-4.43970780351055));
#454353=CARTESIAN_POINT('Ctrl Pts',(-6.39440032516632,24.6674296563851,
-4.55466522035644));
#454354=CARTESIAN_POINT('Ctrl Pts',(-6.98285719109209,24.595946585691,-5.67943270307874));
#454355=CARTESIAN_POINT('Ctrl Pts',(-6.35644809296943,24.5244635149968,
-6.78351377915186));
#454356=CARTESIAN_POINT('Ctrl Pts',(-5.08908040672856,24.4529804443026,
-6.85536457080349));
#454357=CARTESIAN_POINT('Ctrl Pts',(-4.34189895783853,24.3814973736085,
-5.82915637330097));
#454358=CARTESIAN_POINT('Ctrl Pts',(-4.79946109566455,24.3100143029142,
-4.64508700312038));
#454359=CARTESIAN_POINT('Ctrl Pts',(-6.04255469339979,24.2385312322201,
-4.38798450943288));
#454360=CARTESIAN_POINT('Ctrl Pts',(-6.93227451600163,24.1670481615259,
-5.29340265628057));
#454361=CARTESIAN_POINT('Ctrl Pts',(-6.653471517668,24.0955650908317,-6.53180980673916));
#454362=CARTESIAN_POINT('Ctrl Pts',(-5.46158116264518,24.0240820201376,
-6.96859438750187));
#454363=CARTESIAN_POINT('Ctrl Pts',(-4.44859698414461,23.9525989494434,
-6.20358037791699));
#454364=CARTESIAN_POINT('Ctrl Pts',(-4.54260112438938,23.8811158787492,
-4.93766308406974));
#454365=CARTESIAN_POINT('Ctrl Pts',(-5.65746830547292,23.809632808055,-4.33065848211866));
#454366=CARTESIAN_POINT('Ctrl Pts',(-6.77177253027144,23.7381497373608,
-4.93869585450499));
#454367=CARTESIAN_POINT('Ctrl Pts',(-6.86460369448698,23.6666666666667,
-6.20469968353115));
#454368=CARTESIAN_POINT('Ctrl Pts',(-5.85091100812889,23.5951835959725,
-6.96877479819537));
#454369=CARTESIAN_POINT('Ctrl Pts',(-4.65942605482967,23.5237005252783,
-6.53088590401188));
#454370=CARTESIAN_POINT('Ctrl Pts',(-4.3817703393888,23.4522174545841,-5.29222116283617));
#454371=CARTESIAN_POINT('Ctrl Pts',(-5.27232937980428,23.38073438389,-4.38762739003978));
#454372=CARTESIAN_POINT('Ctrl Pts',(-6.51518294322794,23.3092513131958,
-4.6458824334431));
#454373=CARTESIAN_POINT('Ctrl Pts',(-6.97165023343906,23.2377682425016,
-5.83037365343178));
#454374=CARTESIAN_POINT('Ctrl Pts',(-6.22351333955115,23.1662851718074,
-6.85589224549438));
#454375=CARTESIAN_POINT('Ctrl Pts',(-4.9562223676805,23.0948021011132,-6.78286094776533));
#454376=CARTESIAN_POINT('Ctrl Pts',(-4.33081775314232,23.0233190304191,
-5.67821209556232));
#454377=CARTESIAN_POINT('Ctrl Pts',(-4.92035346181854,22.9518359597249,
-4.55396647939442));
#454378=CARTESIAN_POINT('Ctrl Pts',(-6.18457385510163,22.8803528890307,
-4.44022731365593));
#454379=CARTESIAN_POINT('Ctrl Pts',(-6.96547480693525,22.8088698183366,
-5.44103442081458));
#454380=CARTESIAN_POINT('Ctrl Pts',(-6.54710119607151,22.7373867476423,
-6.63978858397884));
#454381=CARTESIAN_POINT('Ctrl Pts',(-5.31375101838665,22.6659036769482,
-6.93756666268009));
#454382=CARTESIAN_POINT('Ctrl Pts',(-4.39345456041576,22.594420606254,-6.062815025304));
#454383=CARTESIAN_POINT('Ctrl Pts',(-4.63327178349906,22.5229375355598,
-4.81438317658877));
#454384=CARTESIAN_POINT('Ctrl Pts',(-5.41441506110672,22.475282155097,-4.49968717359432));
#454385=CARTESIAN_POINT('Ctrl Pts',(-5.78519550592941,22.4514544648656,
-4.54238608881333));
#454386=CARTESIAN_POINT('Ctrl Pts',(-5.13891927882859,26.1456366054031,
-4.75759373111246));
#454387=CARTESIAN_POINT('Ctrl Pts',(-5.43810071821374,26.1218089151717,
-4.58527827879321));
#454388=CARTESIAN_POINT('Ctrl Pts',(-6.21688915400102,26.0741535347089,
-4.5658640060888));
#454389=CARTESIAN_POINT('Ctrl Pts',(-6.87864168992013,26.0026704640147,
-5.53797444142439));
#454390=CARTESIAN_POINT('Ctrl Pts',(-6.41815729896024,25.9311873933205,
-6.61847524998255));
#454391=CARTESIAN_POINT('Ctrl Pts',(-5.26158350250274,25.8597043226264,
-6.81819229031504));
#454392=CARTESIAN_POINT('Ctrl Pts',(-4.46643823922044,25.7882212519322,
-5.95378694567247));
#454393=CARTESIAN_POINT('Ctrl Pts',(-4.7622984340844,25.716738181238,-4.81739664217988));
#454394=CARTESIAN_POINT('Ctrl Pts',(-5.87755291922296,25.6452551105439,
-4.45007439859105));
#454395=CARTESIAN_POINT('Ctrl Pts',(-6.79070035947327,25.5737720398496,
-5.18840274984286));
#454396=CARTESIAN_POINT('Ctrl Pts',(-6.66498514592993,25.5022889691555,
-6.35591148837984));
#454397=CARTESIAN_POINT('Ctrl Pts',(-5.61565848936591,25.4308058984613,
-6.88295739545433));
#454398=CARTESIAN_POINT('Ctrl Pts',(-4.60406196791575,25.3593228277671,
-6.28666204489055));
#454399=CARTESIAN_POINT('Ctrl Pts',(-4.55702527594187,25.2878397570729,
-5.11334619850668));
#454400=CARTESIAN_POINT('Ctrl Pts',(-5.51763314847689,25.2163566863788,
-4.43798405643501));
#454401=CARTESIAN_POINT('Ctrl Pts',(-6.60579479560106,25.1448736156846,
-4.87933393703958));
#454402=CARTESIAN_POINT('Ctrl Pts',(-6.82454899803953,25.0733905449905,
-6.03303673742344));
#454403=CARTESIAN_POINT('Ctrl Pts',(-5.97347744575397,25.0019074742962,
-6.84208605608162));
#454404=CARTESIAN_POINT('Ctrl Pts',(-4.83231952202541,24.9304244036021,
-6.56524194061871));
#454405=CARTESIAN_POINT('Ctrl Pts',(-4.44658873189996,24.8589413329078,
-5.45614521253248));
#454406=CARTESIAN_POINT('Ctrl Pts',(-5.16968614336583,24.7874582622137,
-4.53093499038958));
#454407=CARTESIAN_POINT('Ctrl Pts',(-6.33911995340987,24.7159751915195,
-4.63727615158268));
#454408=CARTESIAN_POINT('Ctrl Pts',(-6.88347096747714,24.6444921208254,
-5.67774038144015));
#454409=CARTESIAN_POINT('Ctrl Pts',(-6.30401230613993,24.5730090501312,
-6.69906868632339));
#454410=CARTESIAN_POINT('Ctrl Pts',(-5.1316360027112,24.501525979437,-6.76553413784902));
#454411=CARTESIAN_POINT('Ctrl Pts',(-4.4404570855349,24.4300429087428,-5.8162420056622));
#454412=CARTESIAN_POINT('Ctrl Pts',(-4.86372415598114,24.3585598380486,
-4.72092066657002));
#454413=CARTESIAN_POINT('Ctrl Pts',(-6.01364575549065,24.2870767673545,
-4.48308844595715));
#454414=CARTESIAN_POINT('Ctrl Pts',(-6.83667955068161,24.2155936966602,
-5.32064394905434));
#454415=CARTESIAN_POINT('Ctrl Pts',(-6.57877331548262,24.1441106259661,
-6.46623035855224));
#454416=CARTESIAN_POINT('Ctrl Pts',(-5.4762171877825,24.0726275552719,-6.87027718549015));
#454417=CARTESIAN_POINT('Ctrl Pts',(-4.5391579116818,24.0011444845778,-6.16260228864267));
#454418=CARTESIAN_POINT('Ctrl Pts',(-4.62611628030964,23.9296614138835,
-4.99156766820889));
#454419=CARTESIAN_POINT('Ctrl Pts',(-5.65742225312448,23.8581783431894,
-4.43005910275823));
#454420=CARTESIAN_POINT('Ctrl Pts',(-6.68820746419386,23.7866952724952,
-4.99252303072782));
#454421=CARTESIAN_POINT('Ctrl Pts',(-6.77408077335862,23.715212201801,-6.16363770038041));
#454422=CARTESIAN_POINT('Ctrl Pts',(-5.83636609328009,23.6437291311068,
-6.87044407409259));
#454423=CARTESIAN_POINT('Ctrl Pts',(-4.73418498174874,23.5722460604127,
-6.46537570391973));
#454424=CARTESIAN_POINT('Ctrl Pts',(-4.47734003862102,23.5007629897185,
-5.31955101057097));
#454425=CARTESIAN_POINT('Ctrl Pts',(-5.30115015081045,23.4292799190243,
-4.48275809327536));
#454426=CARTESIAN_POINT('Ctrl Pts',(-6.4508497069919,23.3577968483301,-4.72165647802515));
#454427=CARTESIAN_POINT('Ctrl Pts',(-6.8731039905307,23.286313777636,-5.81736804855842));
#454428=CARTESIAN_POINT('Ctrl Pts',(-6.18104124059857,23.2148307069418,
-6.76602226241636));
#454429=CARTESIAN_POINT('Ctrl Pts',(-5.00873590166638,23.1433476362476,
-6.69846478576951));
#454430=CARTESIAN_POINT('Ctrl Pts',(-4.43020643614536,23.0718645655534,
-5.67661126055156));
#454431=CARTESIAN_POINT('Ctrl Pts',(-4.97555543184771,23.0003814948593,
-4.63662978245479));
#454432=CARTESIAN_POINT('Ctrl Pts',(-6.1450203373264,22.9288984241651,-4.5314155623581));
#454433=CARTESIAN_POINT('Ctrl Pts',(-6.86739142284001,22.8574153534709,
-5.45721045950911));
#454434=CARTESIAN_POINT('Ctrl Pts',(-6.48037563201499,22.7859322827767,
-6.56611594115257));
#454435=CARTESIAN_POINT('Ctrl Pts',(-5.33946716650399,22.7144492120825,
-6.84157504188551));
#454436=CARTESIAN_POINT('Ctrl Pts',(-4.48814850723257,22.6429661413884,
-6.0323875407531));
#454437=CARTESIAN_POINT('Ctrl Pts',(-4.70999101793355,22.5714830706942,
-4.87752780133468));
#454438=CARTESIAN_POINT('Ctrl Pts',(-5.4325862664886,22.5238276902314,-4.58641880376449));
#454439=CARTESIAN_POINT('Ctrl Pts',(-5.7755760807344,22.5,-4.62591736201901));
#454440=CARTESIAN_POINT('Ctrl Pts',(-6.39006796800885,25.6019615242271,
-4.92443355077908));
#454441=CARTESIAN_POINT('Ctrl Pts',(-6.48712194011206,25.5925650294346,
-5.02053320993752));
#454442=CARTESIAN_POINT('Ctrl Pts',(-6.56580235206401,25.5831685346421,
-5.13467106978717));
#454443=CARTESIAN_POINT('Ctrl Pts',(-6.617556583841,25.5737720398497,-5.25993281439039));
#454444=CARTESIAN_POINT('Ctrl Pts',(-6.74879528829216,25.5499443496183,
-5.57757232935518));
#454445=CARTESIAN_POINT('Ctrl Pts',(-6.70689021711105,25.5261166593869,
-5.96674190886751));
#454446=CARTESIAN_POINT('Ctrl Pts',(-6.51104990542648,25.5022889691555,
-6.24916768313609));
#454447=CARTESIAN_POINT('Ctrl Pts',(-6.31520959374192,25.4784612789241,
-6.53159345740467));
#454448=CARTESIAN_POINT('Ctrl Pts',(-5.96543404155392,25.4546335886927,
-6.7072754264295));
#454449=CARTESIAN_POINT('Ctrl Pts',(-5.62194684521822,25.4308058984613,
-6.69573385251462));
#454450=CARTESIAN_POINT('Ctrl Pts',(-5.27845964888252,25.4069782082299,
-6.68419227859974));
#454451=CARTESIAN_POINT('Ctrl Pts',(-4.94126080839914,25.3831505179985,
-6.48542716174514));
#454452=CARTESIAN_POINT('Ctrl Pts',(-4.76482193949513,25.3593228277671,
-6.19049196225387));
#454453=CARTESIAN_POINT('Ctrl Pts',(-4.58838307059113,25.3354951375357,
-5.89555676276259));
#454454=CARTESIAN_POINT('Ctrl Pts',(-4.5727041732665,25.3116674473043,-5.50445148063464));
#454455=CARTESIAN_POINT('Ctrl Pts',(-4.72496603669335,25.2878397570729,
-5.19633848255872));
#454456=CARTESIAN_POINT('Ctrl Pts',(-4.87722790012021,25.2640120668416,
-4.8882254844828));
#454457=CARTESIAN_POINT('Ctrl Pts',(-5.19743052429855,25.2401843766102,
-4.6631047704589));
#454458=CARTESIAN_POINT('Ctrl Pts',(-5.53889211090841,25.2163566863788,
-4.62410272688105));
#454459=CARTESIAN_POINT('Ctrl Pts',(-5.84649605160076,25.1948916323282,
-4.58896793348097));
#454460=CARTESIAN_POINT('Ctrl Pts',(-6.17135209942283,25.1734265782776,
-4.70487246063661));
#454461=CARTESIAN_POINT('Ctrl Pts',(-6.39198798715976,25.1519615242271,
-4.92254817630007));
#454462=CARTESIAN_POINT('Origin',(-5.65685387860012,26.,-5.65685387860011));
#454463=CARTESIAN_POINT('Origin',(5.65685387860011,26.993675081176,-5.65685387860012));
#454464=CARTESIAN_POINT('Ctrl Pts',(4.74432962138981,25.868675081176,-6.57057130100612));
#454465=CARTESIAN_POINT('Ctrl Pts',(4.78199706987976,25.8656848283261,-6.60882993708831));
#454466=CARTESIAN_POINT('Ctrl Pts',(5.14157728587623,25.8388668852448,-6.92960341635463));
#454467=CARTESIAN_POINT('Ctrl Pts',(6.16255878293893,25.7882212519322,-7.09568592881682));
#454468=CARTESIAN_POINT('Ctrl Pts',(7.13997732676548,25.716738181238,-6.01152748645437));
#454469=CARTESIAN_POINT('Ctrl Pts',(6.7587374620765,25.6452551105438,-4.60259286076204));
#454470=CARTESIAN_POINT('Ctrl Pts',(5.36788602689621,25.5737720398497,-4.15947051927595));
#454471=CARTESIAN_POINT('Ctrl Pts',(4.24182426511434,25.5022889691555,-5.08827462376231));
#454472=CARTESIAN_POINT('Ctrl Pts',(4.36502559631504,25.450589982931,-6.13675122222029));
#454473=CARTESIAN_POINT('Ctrl Pts',(4.69148744470697,25.4227186869378,-6.51790892062316));
#454474=CARTESIAN_POINT('Ctrl Pts',(4.74334636410459,25.418675081176,-6.56885365284802));
#454475=CARTESIAN_POINT('Ctrl Pts',(4.74450601134849,25.906324918824,-6.56704169373441));
#454476=CARTESIAN_POINT('Ctrl Pts',(4.95573944791419,25.8898945654199,-6.7750658664325));
#454477=CARTESIAN_POINT('Ctrl Pts',(5.64807137163848,25.8496365217844,-7.11639071403833));
#454478=CARTESIAN_POINT('Ctrl Pts',(6.8522203629011,25.7855507879174,-6.60321033464885));
#454479=CARTESIAN_POINT('Ctrl Pts',(7.1004834147237,25.7140677172233,-5.16550356767203));
#454480=CARTESIAN_POINT('Ctrl Pts',(6.02596364157129,25.6425846465291,-4.17707919799325));
#454481=CARTESIAN_POINT('Ctrl Pts',(4.61334644908231,25.5711015758349,-4.5448553014618));
#454482=CARTESIAN_POINT('Ctrl Pts',(4.21675923787011,25.5090149999332,-5.74896333949311));
#454483=CARTESIAN_POINT('Ctrl Pts',(4.5629353888518,25.4707561142629,-6.3830054663296));
#454484=CARTESIAN_POINT('Ctrl Pts',(4.74640124271564,25.456324918824,-6.56829321884323));
#454485=CARTESIAN_POINT('Ctrl Pts',(6.69274404704181,26.,-5.59475217632212));
#454486=CARTESIAN_POINT('Ctrl Pts',(6.67208297724159,25.9761723097686,-5.25011429538726));
#454487=CARTESIAN_POINT('Ctrl Pts',(6.25991935236784,25.9285169293058,-4.58904744425369));
#454488=CARTESIAN_POINT('Ctrl Pts',(5.08408179813166,25.8570338586116,-4.5711145089162));
#454489=CARTESIAN_POINT('Ctrl Pts',(4.43501771280631,25.7855507879175,-5.55001366141289));
#454490=CARTESIAN_POINT('Ctrl Pts',(4.90440858615388,25.7140677172233,-6.62575617389683));
#454491=CARTESIAN_POINT('Ctrl Pts',(6.06367191307887,25.6425846465291,-6.81433291744693));
#454492=CARTESIAN_POINT('Ctrl Pts',(6.84996345870369,25.5711015758349,-5.94217367437589));
#454493=CARTESIAN_POINT('Ctrl Pts',(6.54327224197424,25.4996185051408,-4.80874583886255));
#454494=CARTESIAN_POINT('Ctrl Pts',(5.42439156223908,25.4281354344466,-4.45227280795));
#454495=CARTESIAN_POINT('Ctrl Pts',(4.51852288527077,25.3566523637524,-5.19945610983427));
#454496=CARTESIAN_POINT('Ctrl Pts',(4.65556044151951,25.2851692930583,-6.36568271985867));
#454497=CARTESIAN_POINT('Ctrl Pts',(5.70997789504277,25.213686222364,-6.88249940298929));
#454498=CARTESIAN_POINT('Ctrl Pts',(6.71571945020394,25.1422031516699,-6.27639179734011));
#454499=CARTESIAN_POINT('Ctrl Pts',(6.7513451989237,25.0707200809757,-5.10267450019954));
#454500=CARTESIAN_POINT('Ctrl Pts',(5.78421192833873,24.9992370102815,-4.43668748453226));
#454501=CARTESIAN_POINT('Ctrl Pts',(4.7003955508837,24.9277539395873,-4.88860074260098));
#454502=CARTESIAN_POINT('Ctrl Pts',(4.49287282235238,24.8562708688931,-6.04437662247731));
#454503=CARTESIAN_POINT('Ctrl Pts',(5.35177365831405,24.784787798199,-6.84510966506768));
#454504=CARTESIAN_POINT('Ctrl Pts',(6.49018471285718,24.7133047275048,-6.55717903824976));
#454505=CARTESIAN_POINT('Ctrl Pts',(6.86510957377,24.6418216568106,-5.44438294256282));
#454506=CARTESIAN_POINT('Ctrl Pts',(6.13304718756448,24.5703385861164,-4.52624977050191));
#454507=CARTESIAN_POINT('Ctrl Pts',(4.96470306042393,24.4988555154223,-4.64396052187118));
#454508=CARTESIAN_POINT('Ctrl Pts',(4.43049797487471,24.4273724447281,-5.68967021074952));
#454509=CARTESIAN_POINT('Ctrl Pts',(5.01986328076133,24.3558893740339,-6.70531403099034));
#454510=CARTESIAN_POINT('Ctrl Pts',(6.19283059794665,24.2844063033397,-6.76037309820141));
#454511=CARTESIAN_POINT('Ctrl Pts',(6.87474342740734,24.2129232326455,-5.80440305573226));
#454512=CARTESIAN_POINT('Ctrl Pts',(6.44084262551865,24.1414401619514,-4.71325048867858));
#454513=CARTESIAN_POINT('Ctrl Pts',(5.28866213152759,24.0699570912572,-4.4866143522216));
#454514=CARTESIAN_POINT('Ctrl Pts',(4.47381384511066,23.9984740205631,-5.3321355513588));
#454515=CARTESIAN_POINT('Ctrl Pts',(4.74285054378755,23.9269909498688,-6.47515921171814));
#454516=CARTESIAN_POINT('Ctrl Pts',(5.84928450947304,23.8555078791747,-6.86846279219781));
#454517=CARTESIAN_POINT('Ctrl Pts',(6.77941618151556,23.7840248084805,-6.15170698086798));
#454518=CARTESIAN_POINT('Ctrl Pts',(6.68107173221035,23.7125417377863,-4.98157355760958));
#454519=CARTESIAN_POINT('Ctrl Pts',(5.64435299191054,23.6410586670921,-4.43012269359923));
#454520=CARTESIAN_POINT('Ctrl Pts',(4.61908739135743,23.569575596398,-5.00258598787076));
#454521=CARTESIAN_POINT('Ctrl Pts',(4.54460915448657,23.4980925257038,-6.17448062637044));
#454522=CARTESIAN_POINT('Ctrl Pts',(5.48915421344718,23.4266094550096,-6.87213254456039));
#454523=CARTESIAN_POINT('Ctrl Pts',(6.58734339945679,23.3551263843154,-6.45636332421143));
#454524=CARTESIAN_POINT('Ctrl Pts',(6.8330308949199,23.2836433136213,-5.30809370313679));
#454525=CARTESIAN_POINT('Ctrl Pts',(6.00112122066856,23.212160242927,-4.47935503415497));
#454526=CARTESIAN_POINT('Ctrl Pts',(4.85379852261455,23.1406771722329,-4.72942128924326));
#454527=CARTESIAN_POINT('Ctrl Pts',(4.44222413342346,23.0691941015387,-5.82919498069919));
#454528=CARTESIAN_POINT('Ctrl Pts',(5.14347668616412,22.9977110308445,-6.77105943752212));
#454529=CARTESIAN_POINT('Ctrl Pts',(6.31507855179967,22.9262279601504,-6.69212899367236));
#454530=CARTESIAN_POINT('Ctrl Pts',(6.88362364563197,22.8547448894562,-5.66464494341573));
#454531=CARTESIAN_POINT('Ctrl Pts',(6.32821994284799,22.783261818762,-4.63011853598606));
#454532=CARTESIAN_POINT('Ctrl Pts',(5.15771839492686,22.7117787480678,-4.53608521045973));
#454533=CARTESIAN_POINT('Ctrl Pts',(4.44452082366079,22.6402956773736,-5.46925286619013));
#454534=CARTESIAN_POINT('Ctrl Pts',(4.84204067651847,22.5688126066795,-6.57357515235991));
#454535=CARTESIAN_POINT('Ctrl Pts',(5.98608844956735,22.4973295359852,-6.8394368280484));
#454536=CARTESIAN_POINT('Ctrl Pts',(6.82851835303725,22.4258464652911,-6.01893246982621));
#454537=CARTESIAN_POINT('Ctrl Pts',(6.67416374956871,22.3781910848283,-5.25534692011694));
#454538=CARTESIAN_POINT('Ctrl Pts',(6.45251384441992,22.3543633945969,-4.99063298333217));
#454539=CARTESIAN_POINT('Ctrl Pts',(6.77667668816906,26.0485455351344,-5.58972040746333));
#454540=CARTESIAN_POINT('Ctrl Pts',(6.75434156236399,26.024717844903,-5.21715836192049));
#454541=CARTESIAN_POINT('Ctrl Pts',(6.30878252293169,25.9770624644402,-4.50252879876621));
#454542=CARTESIAN_POINT('Ctrl Pts',(5.03767313923882,25.905579393746,-4.48314285357121));
#454543=CARTESIAN_POINT('Ctrl Pts',(4.33601886182374,25.8340963230518,-5.54135696992153));
#454544=CARTESIAN_POINT('Ctrl Pts',(4.84344196766208,25.7626132523576,-6.70426114586779));
#454545=CARTESIAN_POINT('Ctrl Pts',(6.09663420303223,25.6911301816635,-6.90811725457023));
#454546=CARTESIAN_POINT('Ctrl Pts',(6.94663474805762,25.6196471109693,-5.96529161173539));
#454547=CARTESIAN_POINT('Ctrl Pts',(6.61509398200833,25.5481640402751,-4.74002817949571));
#454548=CARTESIAN_POINT('Ctrl Pts',(5.40555638379146,25.4766809695809,-4.35467204505865));
#454549=CARTESIAN_POINT('Ctrl Pts',(4.42629001188529,25.4051978988867,-5.16239561447694));
#454550=CARTESIAN_POINT('Ctrl Pts',(4.57443098853514,25.3337148281926,-6.42311533054124));
#454551=CARTESIAN_POINT('Ctrl Pts',(5.71428225002476,25.2622317574984,-6.98180690592904));
#454552=CARTESIAN_POINT('Ctrl Pts',(6.80151366539291,25.1907486868042,-6.32658964203687));
#454553=CARTESIAN_POINT('Ctrl Pts',(6.84002597802966,25.11926561611,-5.05777230853438));
#454554=CARTESIAN_POINT('Ctrl Pts',(5.79453107008661,25.0477825454159,-4.33782392622387));
#454555=CARTESIAN_POINT('Ctrl Pts',(4.62289884706407,24.9762994747217,-4.82635329907546));
#454556=CARTESIAN_POINT('Ctrl Pts',(4.39856166152736,24.9048164040275,-6.07577551821105));
#454557=CARTESIAN_POINT('Ctrl Pts',(5.32705463942152,24.8333333333333,-6.941387677478));
#454558=CARTESIAN_POINT('Ctrl Pts',(6.55770505428216,24.7618502626391,-6.63012757162216));
#454559=CARTESIAN_POINT('Ctrl Pts',(6.96300807183685,24.690367191945,-5.42716755876279));
#454560=CARTESIAN_POINT('Ctrl Pts',(6.17163058503857,24.6188841212508,-4.4346429653087));
#454561=CARTESIAN_POINT('Ctrl Pts',(4.90862178076926,24.5474010505566,-4.56189118942603));
#454562=CARTESIAN_POINT('Ctrl Pts',(4.33113291369596,24.4759179798625,-5.69232914266461));
#454563=CARTESIAN_POINT('Ctrl Pts',(4.96825133880203,24.4044349091683,-6.7902651507014));
#454564=CARTESIAN_POINT('Ctrl Pts',(6.23625792548383,24.3329518384741,-6.84978535971091));
#454565=CARTESIAN_POINT('Ctrl Pts',(6.97342250511928,24.2614687677799,-5.8163581765647));
#454566=CARTESIAN_POINT('Ctrl Pts',(6.50436504145381,24.1899856970857,-4.6367953517292));
#454567=CARTESIAN_POINT('Ctrl Pts',(5.25882952309621,24.1185026263916,-4.39179610102783));
#454568=CARTESIAN_POINT('Ctrl Pts',(4.37795843727392,24.0470195556974,-5.30582536167067));
#454569=CARTESIAN_POINT('Ctrl Pts',(4.66879374102308,23.9755364850032,-6.54146211713177));
#454570=CARTESIAN_POINT('Ctrl Pts',(5.86487613450724,23.904053414309,-6.96663298362319));
#454571=CARTESIAN_POINT('Ctrl Pts',(6.8703714022368,23.8325703436148,-6.19180228161384));
#454572=CARTESIAN_POINT('Ctrl Pts',(6.76405862808225,23.7610872729207,-4.92685920413014));
#454573=CARTESIAN_POINT('Ctrl Pts',(5.64334011190815,23.6896042022265,-4.33072722538547));
#454574=CARTESIAN_POINT('Ctrl Pts',(4.53500272215099,23.6181211315323,-4.94957415925549));
#454575=CARTESIAN_POINT('Ctrl Pts',(4.45448991200439,23.5466380608381,-6.21642115383373));
#454576=CARTESIAN_POINT('Ctrl Pts',(5.47556640632124,23.475154990144,-6.9706000763964));
#454577=CARTESIAN_POINT('Ctrl Pts',(6.66273598971973,23.4036719194498,-6.52114329936776));
#454578=CARTESIAN_POINT('Ctrl Pts',(6.92833022917403,23.3321888487556,-5.27983553104633));
#454579=CARTESIAN_POINT('Ctrl Pts',(6.02901536249358,23.2607057780614,-4.38394859923605));
#454580=CARTESIAN_POINT('Ctrl Pts',(4.78873124130167,23.1892227073672,-4.6542763857934));
#454581=CARTESIAN_POINT('Ctrl Pts',(4.34380918016856,23.1177396366731,-5.8431588586417));
#454582=CARTESIAN_POINT('Ctrl Pts',(5.1018804774459,23.0462565659789,-6.86133755596363));
#454583=CARTESIAN_POINT('Ctrl Pts',(6.36841097734036,22.9747734952847,-6.77601180031397));
#454584=CARTESIAN_POINT('Ctrl Pts',(6.98302223994139,22.9032904245905,-5.66527621173653));
#454585=CARTESIAN_POINT('Ctrl Pts',(6.3826171450343,22.8318073538963,-4.54692766144198));
#454586=CARTESIAN_POINT('Ctrl Pts',(5.11727611571492,22.7603242832022,-4.4452753183732));
#454587=CARTESIAN_POINT('Ctrl Pts',(4.34629195893472,22.688841212508,-5.45405255931454));
#454588=CARTESIAN_POINT('Ctrl Pts',(4.77602071980922,22.6173581418138,-6.64785217518362));
#454589=CARTESIAN_POINT('Ctrl Pts',(6.01276456633487,22.5458750711197,-6.93525520080945));
#454590=CARTESIAN_POINT('Ctrl Pts',(6.92345206015258,22.4743920004254,-6.04826976192828));
#454591=CARTESIAN_POINT('Ctrl Pts',(6.75659092854625,22.4267366199627,-5.22281495825156));
#454592=CARTESIAN_POINT('Ctrl Pts',(6.5169819168131,22.4029089297313,-4.93665266667552));
#454593=CARTESIAN_POINT('Ctrl Pts',(6.86060932929632,26.0970910702687,-5.58468863860454));
#454594=CARTESIAN_POINT('Ctrl Pts',(6.83660014748639,26.0732633800373,-5.18420242845371));
#454595=CARTESIAN_POINT('Ctrl Pts',(6.35764569349554,26.0256079995746,-4.41601015327873));
#454596=CARTESIAN_POINT('Ctrl Pts',(4.99126448034597,25.9541249288803,-4.39517119822623));
#454597=CARTESIAN_POINT('Ctrl Pts',(4.23702001084117,25.8826418581862,-5.53270027843017));
#454598=CARTESIAN_POINT('Ctrl Pts',(4.7824753491703,25.811158787492,-6.78276611783875));
#454599=CARTESIAN_POINT('Ctrl Pts',(6.12959649298558,25.7396757167979,-7.00190159169352));
#454600=CARTESIAN_POINT('Ctrl Pts',(7.04330603741155,25.6681926461036,-5.98840954909488));
#454601=CARTESIAN_POINT('Ctrl Pts',(6.68691572204242,25.5967095754095,-4.67131052012888));
#454602=CARTESIAN_POINT('Ctrl Pts',(5.38672120534383,25.5252265047153,-4.2570712821673));
#454603=CARTESIAN_POINT('Ctrl Pts',(4.33405713849982,25.4537434340211,-5.12533511911963));
#454604=CARTESIAN_POINT('Ctrl Pts',(4.49330153555078,25.382260363327,-6.48054794122378));
#454605=CARTESIAN_POINT('Ctrl Pts',(5.71858660500674,25.3107772926328,-7.0811144088688));
#454606=CARTESIAN_POINT('Ctrl Pts',(6.88730788058188,25.2392942219386,-6.37678748673361));
#454607=CARTESIAN_POINT('Ctrl Pts',(6.92870675713562,25.1678111512444,-5.01287011686923));
#454608=CARTESIAN_POINT('Ctrl Pts',(5.80485021183448,25.0963280805502,-4.23896036791547));
#454609=CARTESIAN_POINT('Ctrl Pts',(4.54540214324444,25.0248450098561,-4.76410585554996));
#454610=CARTESIAN_POINT('Ctrl Pts',(4.30425050070234,24.9533619391619,-6.10717441394478));
#454611=CARTESIAN_POINT('Ctrl Pts',(5.302335620529,24.8818788684677,-7.03766568988833));
#454612=CARTESIAN_POINT('Ctrl Pts',(6.62522539570715,24.8103957977735,-6.70307610499455));
#454613=CARTESIAN_POINT('Ctrl Pts',(7.06090656990369,24.7389127270793,-5.40995217496277));
#454614=CARTESIAN_POINT('Ctrl Pts',(6.21021398251268,24.6674296563851,-4.34303616011549));
#454615=CARTESIAN_POINT('Ctrl Pts',(4.85254050111457,24.595946585691,-4.47982185698087));
#454616=CARTESIAN_POINT('Ctrl Pts',(4.23176785251722,24.5244635149968,-5.69498807457972));
#454617=CARTESIAN_POINT('Ctrl Pts',(4.91663939684271,24.4529804443027,-6.87521627041245));
#454618=CARTESIAN_POINT('Ctrl Pts',(6.27968525302103,24.3814973736084,-6.93919762122039));
#454619=CARTESIAN_POINT('Ctrl Pts',(7.07210158283119,24.3100143029143,-5.82831329739714));
#454620=CARTESIAN_POINT('Ctrl Pts',(6.567887457389,24.2385312322201,-4.5603402147798));
#454621=CARTESIAN_POINT('Ctrl Pts',(5.22899691466481,24.1670481615259,-4.29697784983407));
#454622=CARTESIAN_POINT('Ctrl Pts',(4.28210302943719,24.0955650908318,-5.27951517198252));
#454623=CARTESIAN_POINT('Ctrl Pts',(4.59473693825861,24.0240820201375,-6.60776502254541));
#454624=CARTESIAN_POINT('Ctrl Pts',(5.88046775954143,23.9525989494434,-7.06480317504856));
#454625=CARTESIAN_POINT('Ctrl Pts',(6.96132662295805,23.8811158787492,-6.2318975823597));
#454626=CARTESIAN_POINT('Ctrl Pts',(6.84704552395415,23.809632808055,-4.87214485065071));
#454627=CARTESIAN_POINT('Ctrl Pts',(5.64232723190576,23.7381497373609,-4.23133175717171));
#454628=CARTESIAN_POINT('Ctrl Pts',(4.45091805294454,23.6666666666667,-4.89656233064023));
#454629=CARTESIAN_POINT('Ctrl Pts',(4.36437066952221,23.5951835959725,-6.25836168129701));
#454630=CARTESIAN_POINT('Ctrl Pts',(5.4619785991953,23.5237005252783,-7.06906760823242));
#454631=CARTESIAN_POINT('Ctrl Pts',(6.73812857998268,23.4522174545842,-6.58592327452409));
#454632=CARTESIAN_POINT('Ctrl Pts',(7.02362956342815,23.3807343838899,-5.25157735895587));
#454633=CARTESIAN_POINT('Ctrl Pts',(6.05690950431861,23.3092513131958,-4.28854216431714));
#454634=CARTESIAN_POINT('Ctrl Pts',(4.72366395998878,23.2377682425016,-4.57913148234355));
#454635=CARTESIAN_POINT('Ctrl Pts',(4.24539422691366,23.1662851718074,-5.8571227365842));
#454636=CARTESIAN_POINT('Ctrl Pts',(5.06028426872769,23.0948021011132,-6.95161567440516));
#454637=CARTESIAN_POINT('Ctrl Pts',(6.42174340288106,23.0233190304191,-6.85989460695557));
#454638=CARTESIAN_POINT('Ctrl Pts',(7.08242083425081,22.9518359597249,-5.66590748005734));
#454639=CARTESIAN_POINT('Ctrl Pts',(6.4370143472206,22.8803528890307,-4.46373678689788));
#454640=CARTESIAN_POINT('Ctrl Pts',(5.07683383650299,22.8088698183366,-4.35446542628666));
#454641=CARTESIAN_POINT('Ctrl Pts',(4.24806309420865,22.7373867476423,-5.43885225243895));
#454642=CARTESIAN_POINT('Ctrl Pts',(4.71000076309996,22.6659036769482,-6.72212919800733));
#454643=CARTESIAN_POINT('Ctrl Pts',(6.03944068310239,22.594420606254,-7.03107357357049));
#454644=CARTESIAN_POINT('Ctrl Pts',(7.01838576726789,22.5229375355598,-6.07760705403036));
#454645=CARTESIAN_POINT('Ctrl Pts',(6.83901810752379,22.475282155097,-5.19028299638619));
#454646=CARTESIAN_POINT('Ctrl Pts',(6.58144998920627,22.4514544648656,-4.88267235001886));
#454647=CARTESIAN_POINT('Ctrl Pts',(6.94454197042357,26.1456366054031,-5.57965686974575));
#454648=CARTESIAN_POINT('Ctrl Pts',(6.91885873260879,26.1218089151717,-5.15124649498694));
#454649=CARTESIAN_POINT('Ctrl Pts',(6.4065088640594,26.0741535347089,-4.32949150779126));
#454650=CARTESIAN_POINT('Ctrl Pts',(4.94485582145311,26.0026704640147,-4.30719954288124));
#454651=CARTESIAN_POINT('Ctrl Pts',(4.1380211598586,25.9311873933206,-5.52404358693881));
#454652=CARTESIAN_POINT('Ctrl Pts',(4.7215087306785,25.8597043226263,-6.86127108980971));
#454653=CARTESIAN_POINT('Ctrl Pts',(6.16255878293893,25.7882212519322,-7.09568592881682));
#454654=CARTESIAN_POINT('Ctrl Pts',(7.13997732676548,25.716738181238,-6.01152748645437));
#454655=CARTESIAN_POINT('Ctrl Pts',(6.7587374620765,25.6452551105438,-4.60259286076204));
#454656=CARTESIAN_POINT('Ctrl Pts',(5.36788602689621,25.5737720398497,-4.15947051927595));
#454657=CARTESIAN_POINT('Ctrl Pts',(4.24182426511434,25.5022889691555,-5.08827462376231));
#454658=CARTESIAN_POINT('Ctrl Pts',(4.41217208256641,25.4308058984613,-6.53798055190634));
#454659=CARTESIAN_POINT('Ctrl Pts',(5.72289095998872,25.3593228277671,-7.18042191180854));
#454660=CARTESIAN_POINT('Ctrl Pts',(6.97310209577086,25.287839757073,-6.42698533143036));
#454661=CARTESIAN_POINT('Ctrl Pts',(7.01738753624157,25.2163566863788,-4.96796792520408));
#454662=CARTESIAN_POINT('Ctrl Pts',(5.81516935358236,25.1448736156846,-4.14009680960707));
#454663=CARTESIAN_POINT('Ctrl Pts',(4.46790543942481,25.0733905449904,-4.70185841202445));
#454664=CARTESIAN_POINT('Ctrl Pts',(4.20993933987732,25.0019074742962,-6.1385733096785));
#454665=CARTESIAN_POINT('Ctrl Pts',(5.27761660163647,24.930424403602,-7.13394370229866));
#454666=CARTESIAN_POINT('Ctrl Pts',(6.69274573713214,24.8589413329079,-6.77602463836695));
#454667=CARTESIAN_POINT('Ctrl Pts',(7.15880506797054,24.7874582622137,-5.39273679116275));
#454668=CARTESIAN_POINT('Ctrl Pts',(6.24879737998679,24.7159751915195,-4.25142935492228));
#454669=CARTESIAN_POINT('Ctrl Pts',(4.79645922145989,24.6444921208253,-4.39775252453571));
#454670=CARTESIAN_POINT('Ctrl Pts',(4.13240279133847,24.5730090501312,-5.69764700649481));
#454671=CARTESIAN_POINT('Ctrl Pts',(4.86502745488341,24.501525979437,-6.9601673901235));
#454672=CARTESIAN_POINT('Ctrl Pts',(6.32311258055821,24.4300429087428,-7.02860988272989));
#454673=CARTESIAN_POINT('Ctrl Pts',(7.17078066054311,24.3585598380486,-5.84026841822957));
#454674=CARTESIAN_POINT('Ctrl Pts',(6.63140987332417,24.2870767673545,-4.4838850778304));
#454675=CARTESIAN_POINT('Ctrl Pts',(5.19916430623342,24.2155936966603,-4.2021595986403));
#454676=CARTESIAN_POINT('Ctrl Pts',(4.18624762160045,24.1441106259661,-5.25320498229437));
#454677=CARTESIAN_POINT('Ctrl Pts',(4.52068013549415,24.0726275552719,-6.67406792795906));
#454678=CARTESIAN_POINT('Ctrl Pts',(5.89605938457563,24.0011444845777,-7.16297336647392));
#454679=CARTESIAN_POINT('Ctrl Pts',(7.0522818436793,23.9296614138836,-6.27199288310558));
#454680=CARTESIAN_POINT('Ctrl Pts',(6.93003241982605,23.8581783431894,-4.81743049717126));
#454681=CARTESIAN_POINT('Ctrl Pts',(5.64131435190337,23.7866952724952,-4.13193628895796));
#454682=CARTESIAN_POINT('Ctrl Pts',(4.3668333837381,23.715212201801,-4.84355050202496));
#454683=CARTESIAN_POINT('Ctrl Pts',(4.27425142704003,23.6437291311069,-6.30030220876029));
#454684=CARTESIAN_POINT('Ctrl Pts',(5.44839079206936,23.5722460604127,-7.16753514006844));
#454685=CARTESIAN_POINT('Ctrl Pts',(6.81352117024561,23.5007629897185,-6.65070324968042));
#454686=CARTESIAN_POINT('Ctrl Pts',(7.11892889768229,23.4292799190243,-5.22331918686542));
#454687=CARTESIAN_POINT('Ctrl Pts',(6.08480364614364,23.3577968483302,-4.19313572939824));
#454688=CARTESIAN_POINT('Ctrl Pts',(4.65859667867589,23.2863137776359,-4.50398657889369));
#454689=CARTESIAN_POINT('Ctrl Pts',(4.14697927365876,23.2148307069418,-5.8710866145267));
#454690=CARTESIAN_POINT('Ctrl Pts',(5.01868806000948,23.1433476362476,-7.04189379284668));
#454691=CARTESIAN_POINT('Ctrl Pts',(6.47507582842176,23.0718645655535,-6.94377741359719));
#454692=CARTESIAN_POINT('Ctrl Pts',(7.18181942856023,23.0003814948592,-5.66653874837813));
#454693=CARTESIAN_POINT('Ctrl Pts',(6.49141154940691,22.9288984241651,-4.38054591235379));
#454694=CARTESIAN_POINT('Ctrl Pts',(5.03639155729104,22.8574153534709,-4.26365553420012));
#454695=CARTESIAN_POINT('Ctrl Pts',(4.14983422948258,22.7859322827767,-5.42365194556336));
#454696=CARTESIAN_POINT('Ctrl Pts',(4.6439808063907,22.7144492120825,-6.79640622083105));
#454697=CARTESIAN_POINT('Ctrl Pts',(6.06611679986992,22.6429661413884,-7.12689194633153));
#454698=CARTESIAN_POINT('Ctrl Pts',(7.11331947438321,22.5714830706942,-6.10694434613243));
#454699=CARTESIAN_POINT('Ctrl Pts',(6.92144528650133,22.5238276902314,-5.15775103452081));
#454700=CARTESIAN_POINT('Ctrl Pts',(6.64591806159944,22.5,-4.8286920333622));
#454701=CARTESIAN_POINT('Ctrl Pts',(4.92197603118329,25.2730384757729,-6.39051881327128));
#454702=CARTESIAN_POINT('Ctrl Pts',(4.8802577415671,25.2770820815347,-6.34953594825859));
#454703=CARTESIAN_POINT('Ctrl Pts',(4.84215579969382,25.2811256872965,-6.3050503566324));
#454704=CARTESIAN_POINT('Ctrl Pts',(4.80845709106526,25.2851692930582,-6.25744773204304));
#454705=CARTESIAN_POINT('Ctrl Pts',(4.60988125610326,25.3089969832896,-5.97694051651721));
#454706=CARTESIAN_POINT('Ctrl Pts',(4.56420207068701,25.332824673521,-5.58819831317574));
#454707=CARTESIAN_POINT('Ctrl Pts',(4.69234059080694,25.3566523637524,-5.26929666119096));
#454708=CARTESIAN_POINT('Ctrl Pts',(4.82047911092687,25.3804800539838,-4.95039500920618));
#454709=CARTESIAN_POINT('Ctrl Pts',(5.12243533658298,25.4043077442152,-4.70133390857809));
#454710=CARTESIAN_POINT('Ctrl Pts',(5.45989356270023,25.4281354344466,-4.6362155300828));
#454711=CARTESIAN_POINT('Ctrl Pts',(5.79735178881747,25.451963124678,-4.57109715158752));
#454712=CARTESIAN_POINT('Ctrl Pts',(6.17031201539585,25.4757908149094,-4.68992149522503));
#454713=CARTESIAN_POINT('Ctrl Pts',(6.40790733147329,25.4996185051408,-4.93823830629602));
#454714=CARTESIAN_POINT('Ctrl Pts',(6.64550264755072,25.5234461953722,-5.186555117367));
#454715=CARTESIAN_POINT('Ctrl Pts',(6.74773305312721,25.5472738856035,-5.56436439587145));
#454716=CARTESIAN_POINT('Ctrl Pts',(6.66779966497798,25.5711015758349,-5.89862890896884));
#454717=CARTESIAN_POINT('Ctrl Pts',(6.58786627682875,25.5949292660663,-6.23289342206624));
#454718=CARTESIAN_POINT('Ctrl Pts',(6.32576909495381,25.6187569562977,-6.52361316975658));
#454719=CARTESIAN_POINT('Ctrl Pts',(6.00150994952884,25.6425846465291,-6.63754358634341));
#454720=CARTESIAN_POINT('Ctrl Pts',(5.67725080410387,25.6664123367605,-6.75147400293023));
#454721=CARTESIAN_POINT('Ctrl Pts',(5.29082969512888,25.6902400269919,-6.68861508841353));
#454722=CARTESIAN_POINT('Ctrl Pts',(5.01938732841678,25.7140677172233,-6.47789521240786));
#454723=CARTESIAN_POINT('Ctrl Pts',(4.98532270432787,25.7170579700732,-6.45145094929911));
#454724=CARTESIAN_POINT('Ctrl Pts',(4.95306887608107,25.720048222923,-6.42267802952734));
#454725=CARTESIAN_POINT('Ctrl Pts',(4.92276701974739,25.7230384757729,-6.39190058798136));
#454726=CARTESIAN_POINT('Ctrl Pts',(4.53900700771688,26.,-5.01302286563431));
#454727=CARTESIAN_POINT('Ctrl Pts',(4.32480615636363,25.9761723097686,-5.38492752167559));
#454728=CARTESIAN_POINT('Ctrl Pts',(4.30067277954968,25.9285169293058,-6.35301914505848));
#454729=CARTESIAN_POINT('Ctrl Pts',(5.50907794609547,25.8570338586117,-7.1756264891545));
#454730=CARTESIAN_POINT('Ctrl Pts',(6.8522203629011,25.7855507879174,-6.60321033464885));
#454731=CARTESIAN_POINT('Ctrl Pts',(7.1004834147237,25.7140677172233,-5.16550356767203));
#454732=CARTESIAN_POINT('Ctrl Pts',(6.02596364157129,25.6425846465291,-4.17707919799325));
#454733=CARTESIAN_POINT('Ctrl Pts',(4.61334644908231,25.5711015758349,-4.5448553014618));
#454734=CARTESIAN_POINT('Ctrl Pts',(4.15673773385264,25.4996185051408,-5.93119910857215));
#454735=CARTESIAN_POINT('Ctrl Pts',(5.07453447980768,25.4281354344466,-7.0663089114369));
#454736=CARTESIAN_POINT('Ctrl Pts',(6.5258341885166,25.3566523637524,-6.9100356033464));
#454737=CARTESIAN_POINT('Ctrl Pts',(7.18099123031483,25.2851692930582,-5.60564496305001));
#454738=CARTESIAN_POINT('Ctrl Pts',(6.43975200870338,25.213686222364,-4.34815567114858));
#454739=CARTESIAN_POINT('Ctrl Pts',(4.98123363545819,25.1422031516699,-4.2896855842815));
#454740=CARTESIAN_POINT('Ctrl Pts',(4.14170854437417,25.0707200809757,-5.48379221455872));
#454741=CARTESIAN_POINT('Ctrl Pts',(4.69033908735646,24.9992370102815,-6.83645762028281));
#454742=CARTESIAN_POINT('Ctrl Pts',(6.12447699388038,24.9277539395874,-7.10838527255516));
#454743=CARTESIAN_POINT('Ctrl Pts',(7.13018513270865,24.8562708688931,-6.05044038944422));
#454744=CARTESIAN_POINT('Ctrl Pts',(6.78604742232836,24.784787798199,-4.63189669239788));
#454745=CARTESIAN_POINT('Ctrl Pts',(5.40735816264999,24.7133047275048,-4.15240479236239));
#454746=CARTESIAN_POINT('Ctrl Pts',(4.25725342975252,24.6418216568106,-5.0512683537124));
#454747=CARTESIAN_POINT('Ctrl Pts',(4.38944335790391,24.5703385861164,-6.50496106867921));
#454748=CARTESIAN_POINT('Ctrl Pts',(5.68281734635597,24.4988555154223,-7.18162963832198));
#454749=CARTESIAN_POINT('Ctrl Pts',(6.95240396480877,24.4273724447281,-6.46131966662841));
#454750=CARTESIAN_POINT('Ctrl Pts',(7.03502543671246,24.3558893740339,-5.00396921476326));
#454751=CARTESIAN_POINT('Ctrl Pts',(5.85498510857852,24.2844063033397,-4.14478270244581));
#454752=CARTESIAN_POINT('Ctrl Pts',(4.49341967622111,24.2129232326456,-4.67093497503137));
#454753=CARTESIAN_POINT('Ctrl Pts',(4.19777663638434,24.1414401619514,-6.10037256921808));
#454754=CARTESIAN_POINT('Ctrl Pts',(5.23892007073304,24.0699570912572,-7.12346444664167));
#454755=CARTESIAN_POINT('Ctrl Pts',(6.662968703113,23.998474020563,-6.80286792203874));
#454756=CARTESIAN_POINT('Ctrl Pts',(7.16522879152533,23.9269909498688,-5.43230911237055));
#454757=CARTESIAN_POINT('Ctrl Pts',(6.2855365564656,23.8555078791747,-4.26747512907024));
#454758=CARTESIAN_POINT('Ctrl Pts',(4.82985391579145,23.7840248084805,-4.37557081254884));
#454759=CARTESIAN_POINT('Ctrl Pts',(4.13185724083954,23.7125417377863,-5.6575604101698));
#454760=CARTESIAN_POINT('Ctrl Pts',(4.83104150205928,23.6410586670921,-6.93890266242659));
#454761=CARTESIAN_POINT('Ctrl Pts',(6.28682364983267,23.569575596398,-7.04564953674368));
#454762=CARTESIAN_POINT('Ctrl Pts',(7.16543624640093,23.4980925257038,-5.88000083782647));
#454763=CARTESIAN_POINT('Ctrl Pts',(6.66190630419616,23.4266094550096,-4.50990820099157));
#454764=CARTESIAN_POINT('Ctrl Pts',(5.23756146736659,23.3551263843154,-4.19063094092434));
#454765=CARTESIAN_POINT('Ctrl Pts',(4.19736598356861,23.2836433136212,-5.21468783779197));
#454766=CARTESIAN_POINT('Ctrl Pts',(4.49433434427903,23.2121602429271,-6.64384941569999));
#454767=CARTESIAN_POINT('Ctrl Pts',(5.85638486317849,23.1406771722328,-7.16874271925581));
#454768=CARTESIAN_POINT('Ctrl Pts',(7.03563221165043,23.0691941015387,-6.3084575374563));
#454769=CARTESIAN_POINT('Ctrl Pts',(6.95165327175697,22.9977110308445,-4.85119529970874));
#454770=CARTESIAN_POINT('Ctrl Pts',(5.68141376558385,22.9262279601503,-4.13204038713624));
#454771=CARTESIAN_POINT('Ctrl Pts',(4.38863987327371,22.8547448894562,-4.80994952176022));
#454772=CARTESIAN_POINT('Ctrl Pts',(4.25785081625157,22.783261818762,-6.26368089065207));
#454773=CARTESIAN_POINT('Ctrl Pts',(5.40868234342555,22.7117787480678,-7.16164157512573));
#454774=CARTESIAN_POINT('Ctrl Pts',(6.78713386963136,22.6402956773736,-6.68055232418451));
#454775=CARTESIAN_POINT('Ctrl Pts',(7.12954990426926,22.5688126066795,-5.26231872215201));
#454776=CARTESIAN_POINT('Ctrl Pts',(6.1236699944058,22.4973295359853,-4.20406666678213));
#454777=CARTESIAN_POINT('Ctrl Pts',(4.68809392709695,22.4258464652911,-4.4798333146301));
#454778=CARTESIAN_POINT('Ctrl Pts',(4.32622391325397,22.3781910848283,-5.37807265034296));
#454779=CARTESIAN_POINT('Ctrl Pts',(4.37532354240196,22.3543633945969,-5.80443435631943));
#454780=CARTESIAN_POINT('Ctrl Pts',(4.61186924884874,26.0485455351344,-5.05498833669907));
#454781=CARTESIAN_POINT('Ctrl Pts',(4.41163019717349,26.024717844903,-5.40265192052164));
#454782=CARTESIAN_POINT('Ctrl Pts',(4.38906985506272,25.9770624644402,-6.30764248137266));
#454783=CARTESIAN_POINT('Ctrl Pts',(5.51871011120511,25.905579393746,-7.07663155607638));
#454784=CARTESIAN_POINT('Ctrl Pts',(6.77430532526158,25.8340963230518,-6.54152598941931));
#454785=CARTESIAN_POINT('Ctrl Pts',(7.00638637325414,25.7626132523576,-5.1975302126156));
#454786=CARTESIAN_POINT('Ctrl Pts',(6.00190474293836,25.6911301816635,-4.27353221173565));
#454787=CARTESIAN_POINT('Ctrl Pts',(4.68136318011483,25.6196471109693,-4.61733634566933));
#454788=CARTESIAN_POINT('Ctrl Pts',(4.25451662209878,25.5481640402751,-5.91331704545576));
#454789=CARTESIAN_POINT('Ctrl Pts',(5.11249056981941,25.4766809695809,-6.97443939411568));
#454790=CARTESIAN_POINT('Ctrl Pts',(6.46919328847102,25.4051978988868,-6.82835211754092));
#454791=CARTESIAN_POINT('Ctrl Pts',(7.08164661869466,25.3337148281926,-5.60898280515531));
#454792=CARTESIAN_POINT('Ctrl Pts',(6.38872202076577,25.2622317574984,-4.43345777007097));
#454793=CARTESIAN_POINT('Ctrl Pts',(5.02527115647435,25.1907486868042,-4.37879881483497));
#454794=CARTESIAN_POINT('Ctrl Pts',(4.24046704839444,25.1192656161101,-5.49507252586477));
#454795=CARTESIAN_POINT('Ctrl Pts',(4.75333737058418,25.0477825454159,-6.75957001205557));
#454796=CARTESIAN_POINT('Ctrl Pts',(6.09399690839473,24.9762994747217,-7.01377318104995));
#454797=CARTESIAN_POINT('Ctrl Pts',(7.03415210716631,24.9048164040275,-6.0247860748808));
#454798=CARTESIAN_POINT('Ctrl Pts',(6.71244559509181,24.8333333333333,-4.69870430227373));
#454799=CARTESIAN_POINT('Ctrl Pts',(5.42362051261083,24.7618502626392,-4.25046610554157));
#454800=CARTESIAN_POINT('Ctrl Pts',(4.34848061663153,24.690367191945,-5.09074095026355));
#454801=CARTESIAN_POINT('Ctrl Pts',(4.47205428913018,24.6188841212508,-6.44968069692276));
#454802=CARTESIAN_POINT('Ctrl Pts',(5.68112502471735,24.5474010505566,-7.08224341470705));
#454803=CARTESIAN_POINT('Ctrl Pts',(6.86795887198031,24.4759179798625,-6.40888387979891));
#454804=CARTESIAN_POINT('Ctrl Pts',(6.94519500375798,24.4044349091682,-5.04652481074592));
#454805=CARTESIAN_POINT('Ctrl Pts',(5.84207074093974,24.3329518384741,-4.24334083014217));
#454806=CARTESIAN_POINT('Ctrl Pts',(4.56925333967074,24.2614687677799,-4.73519803534797));
#454807=CARTESIAN_POINT('Ctrl Pts',(4.29288057290861,24.1899856970857,-6.07146363130893));
#454808=CARTESIAN_POINT('Ctrl Pts',(5.2661613635068,24.1185026263916,-7.02786948132165));
#454809=CARTESIAN_POINT('Ctrl Pts',(6.59738925492608,24.0470195556973,-6.72816971985337));
#454810=CARTESIAN_POINT('Ctrl Pts',(7.0669115895136,23.9755364850032,-5.44694513750787));
#454811=CARTESIAN_POINT('Ctrl Pts',(6.24455846719129,23.904053414309,-4.35803605660742));
#454812=CARTESIAN_POINT('Ctrl Pts',(4.8837584999306,23.8325703436148,-4.45908596846911));
#454813=CARTESIAN_POINT('Ctrl Pts',(4.2312578614791,23.7610872729207,-5.65751435782136));
#454814=CARTESIAN_POINT('Ctrl Pts',(4.88486867828213,23.6896042022265,-6.85533759634902));
#454815=CARTESIAN_POINT('Ctrl Pts',(6.24576166668191,23.6181211315323,-6.95512661561532));
#454816=CARTESIAN_POINT('Ctrl Pts',(7.06710552229815,23.5466380608381,-5.86545592297769));
#454817=CARTESIAN_POINT('Ctrl Pts',(6.59639610410402,23.475154990144,-4.58466712791061));
#454818=CARTESIAN_POINT('Ctrl Pts',(5.26489131510138,23.4036719194498,-4.28620064015658));
#454819=CARTESIAN_POINT('Ctrl Pts',(4.2924966868042,23.3321888487556,-5.24350860879812));
#454820=CARTESIAN_POINT('Ctrl Pts',(4.57010838886106,23.2607057780614,-6.57951617946397));
#454821=CARTESIAN_POINT('Ctrl Pts',(5.84337925830513,23.1892227073672,-7.07019647634743));
#454822=CARTESIAN_POINT('Ctrl Pts',(6.94576222857241,23.1177396366731,-6.26598543850373));
#454823=CARTESIAN_POINT('Ctrl Pts',(6.86725710976114,23.0462565659789,-4.90370883369462));
#454824=CARTESIAN_POINT('Ctrl Pts',(5.67981293057309,22.9747734952847,-4.23142907013928));
#454825=CARTESIAN_POINT('Ctrl Pts',(4.47130317633407,22.9032904245905,-4.86515149178938));
#454826=CARTESIAN_POINT('Ctrl Pts',(4.34903906495375,22.8318073538963,-6.22412737287685));
#454827=CARTESIAN_POINT('Ctrl Pts',(5.42485838212006,22.7603242832022,-7.06355819103049));
#454828=CARTESIAN_POINT('Ctrl Pts',(6.7134612268051,22.688841212508,-6.613826760128));
#454829=CARTESIAN_POINT('Ctrl Pts',(7.03355828347467,22.6173581418138,-5.28803487026933));
#454830=CARTESIAN_POINT('Ctrl Pts',(6.0932425098549,22.5458750711196,-4.29876061359894));
#454831=CARTESIAN_POINT('Ctrl Pts',(4.75123855184285,22.4743920004255,-4.55655254906459));
#454832=CARTESIAN_POINT('Ctrl Pts',(4.41295554342414,22.4267366199627,-5.39624385572484));
#454833=CARTESIAN_POINT('Ctrl Pts',(4.45885481560764,22.4029089297313,-5.79481493112442));
#454834=CARTESIAN_POINT('Ctrl Pts',(4.6847314899806,26.0970910702687,-5.09695380776383));
#454835=CARTESIAN_POINT('Ctrl Pts',(4.49845423798335,26.0732633800373,-5.42037631936769));
#454836=CARTESIAN_POINT('Ctrl Pts',(4.47746693057576,26.0256079995745,-6.26226581768684));
#454837=CARTESIAN_POINT('Ctrl Pts',(5.52834227631475,25.9541249288804,-6.97763662299825));
#454838=CARTESIAN_POINT('Ctrl Pts',(6.69639028762207,25.8826418581862,-6.47984164418979));
#454839=CARTESIAN_POINT('Ctrl Pts',(6.91228933178459,25.811158787492,-5.22955685755916));
#454840=CARTESIAN_POINT('Ctrl Pts',(5.97784584430541,25.7396757167978,-4.36998522547805));
#454841=CARTESIAN_POINT('Ctrl Pts',(4.74937991114735,25.6681926461037,-4.68981738987686));
#454842=CARTESIAN_POINT('Ctrl Pts',(4.35229551034492,25.5967095754095,-5.89543498233936));
#454843=CARTESIAN_POINT('Ctrl Pts',(5.15044665983114,25.5252265047153,-6.88256987679449));
#454844=CARTESIAN_POINT('Ctrl Pts',(6.41255238842542,25.4537434340211,-6.74666863173542));
#454845=CARTESIAN_POINT('Ctrl Pts',(6.9823020070745,25.3822603633269,-5.61232064726062));
#454846=CARTESIAN_POINT('Ctrl Pts',(6.33769203282816,25.3107772926328,-4.51875986899335));
#454847=CARTESIAN_POINT('Ctrl Pts',(5.06930867749052,25.2392942219386,-4.46791204538843));
#454848=CARTESIAN_POINT('Ctrl Pts',(4.33922555241473,25.1678111512444,-5.50635283717082));
#454849=CARTESIAN_POINT('Ctrl Pts',(4.81633565381187,25.0963280805502,-6.68268240382832));
#454850=CARTESIAN_POINT('Ctrl Pts',(6.06351682290909,25.0248450098561,-6.91916108954474));
#454851=CARTESIAN_POINT('Ctrl Pts',(6.93811908162396,24.9533619391618,-5.99913176031739));
#454852=CARTESIAN_POINT('Ctrl Pts',(6.63884376785526,24.8818788684677,-4.76551191214956));
#454853=CARTESIAN_POINT('Ctrl Pts',(5.43988286257166,24.8103957977735,-4.34852741872077));
#454854=CARTESIAN_POINT('Ctrl Pts',(4.43970780351055,24.7389127270794,-5.13021354681468));
#454855=CARTESIAN_POINT('Ctrl Pts',(4.55466522035644,24.6674296563851,-6.39440032516632));
#454856=CARTESIAN_POINT('Ctrl Pts',(5.67943270307874,24.595946585691,-6.98285719109209));
#454857=CARTESIAN_POINT('Ctrl Pts',(6.78351377915186,24.5244635149968,-6.35644809296943));
#454858=CARTESIAN_POINT('Ctrl Pts',(6.85536457080349,24.4529804443026,-5.08908040672856));
#454859=CARTESIAN_POINT('Ctrl Pts',(5.82915637330097,24.3814973736085,-4.34189895783853));
#454860=CARTESIAN_POINT('Ctrl Pts',(4.64508700312038,24.3100143029142,-4.79946109566455));
#454861=CARTESIAN_POINT('Ctrl Pts',(4.38798450943288,24.2385312322201,-6.04255469339979));
#454862=CARTESIAN_POINT('Ctrl Pts',(5.29340265628057,24.1670481615259,-6.93227451600163));
#454863=CARTESIAN_POINT('Ctrl Pts',(6.53180980673916,24.0955650908317,-6.653471517668));
#454864=CARTESIAN_POINT('Ctrl Pts',(6.96859438750187,24.0240820201376,-5.46158116264518));
#454865=CARTESIAN_POINT('Ctrl Pts',(6.20358037791699,23.9525989494434,-4.44859698414461));
#454866=CARTESIAN_POINT('Ctrl Pts',(4.93766308406974,23.8811158787492,-4.54260112438938));
#454867=CARTESIAN_POINT('Ctrl Pts',(4.33065848211866,23.809632808055,-5.65746830547292));
#454868=CARTESIAN_POINT('Ctrl Pts',(4.93869585450499,23.7381497373608,-6.77177253027144));
#454869=CARTESIAN_POINT('Ctrl Pts',(6.20469968353115,23.6666666666667,-6.86460369448698));
#454870=CARTESIAN_POINT('Ctrl Pts',(6.96877479819537,23.5951835959725,-5.85091100812889));
#454871=CARTESIAN_POINT('Ctrl Pts',(6.53088590401188,23.5237005252783,-4.65942605482967));
#454872=CARTESIAN_POINT('Ctrl Pts',(5.29222116283617,23.4522174545841,-4.3817703393888));
#454873=CARTESIAN_POINT('Ctrl Pts',(4.38762739003978,23.38073438389,-5.27232937980428));
#454874=CARTESIAN_POINT('Ctrl Pts',(4.6458824334431,23.3092513131958,-6.51518294322794));
#454875=CARTESIAN_POINT('Ctrl Pts',(5.83037365343178,23.2377682425016,-6.97165023343906));
#454876=CARTESIAN_POINT('Ctrl Pts',(6.85589224549438,23.1662851718074,-6.22351333955115));
#454877=CARTESIAN_POINT('Ctrl Pts',(6.78286094776533,23.0948021011132,-4.9562223676805));
#454878=CARTESIAN_POINT('Ctrl Pts',(5.67821209556232,23.0233190304191,-4.33081775314232));
#454879=CARTESIAN_POINT('Ctrl Pts',(4.55396647939442,22.9518359597249,-4.92035346181854));
#454880=CARTESIAN_POINT('Ctrl Pts',(4.44022731365593,22.8803528890307,-6.18457385510163));
#454881=CARTESIAN_POINT('Ctrl Pts',(5.44103442081458,22.8088698183366,-6.96547480693525));
#454882=CARTESIAN_POINT('Ctrl Pts',(6.63978858397884,22.7373867476423,-6.54710119607151));
#454883=CARTESIAN_POINT('Ctrl Pts',(6.93756666268009,22.6659036769482,-5.31375101838665));
#454884=CARTESIAN_POINT('Ctrl Pts',(6.062815025304,22.594420606254,-4.39345456041576));
#454885=CARTESIAN_POINT('Ctrl Pts',(4.81438317658877,22.5229375355598,-4.63327178349906));
#454886=CARTESIAN_POINT('Ctrl Pts',(4.49968717359432,22.475282155097,-5.41441506110672));
#454887=CARTESIAN_POINT('Ctrl Pts',(4.54238608881333,22.4514544648656,-5.78519550592941));
#454888=CARTESIAN_POINT('Ctrl Pts',(4.75759373111246,26.1456366054031,-5.13891927882859));
#454889=CARTESIAN_POINT('Ctrl Pts',(4.58527827879321,26.1218089151717,-5.43810071821374));
#454890=CARTESIAN_POINT('Ctrl Pts',(4.5658640060888,26.0741535347089,-6.21688915400102));
#454891=CARTESIAN_POINT('Ctrl Pts',(5.53797444142439,26.0026704640147,-6.87864168992013));
#454892=CARTESIAN_POINT('Ctrl Pts',(6.61847524998255,25.9311873933205,-6.41815729896024));
#454893=CARTESIAN_POINT('Ctrl Pts',(6.81819229031504,25.8597043226264,-5.26158350250274));
#454894=CARTESIAN_POINT('Ctrl Pts',(5.95378694567247,25.7882212519322,-4.46643823922044));
#454895=CARTESIAN_POINT('Ctrl Pts',(4.81739664217988,25.716738181238,-4.7622984340844));
#454896=CARTESIAN_POINT('Ctrl Pts',(4.45007439859105,25.6452551105439,-5.87755291922296));
#454897=CARTESIAN_POINT('Ctrl Pts',(5.18840274984286,25.5737720398496,-6.79070035947327));
#454898=CARTESIAN_POINT('Ctrl Pts',(6.35591148837984,25.5022889691555,-6.66498514592993));
#454899=CARTESIAN_POINT('Ctrl Pts',(6.88295739545433,25.4308058984613,-5.61565848936591));
#454900=CARTESIAN_POINT('Ctrl Pts',(6.28666204489055,25.3593228277671,-4.60406196791575));
#454901=CARTESIAN_POINT('Ctrl Pts',(5.11334619850668,25.2878397570729,-4.55702527594187));
#454902=CARTESIAN_POINT('Ctrl Pts',(4.43798405643501,25.2163566863788,-5.51763314847689));
#454903=CARTESIAN_POINT('Ctrl Pts',(4.87933393703958,25.1448736156846,-6.60579479560106));
#454904=CARTESIAN_POINT('Ctrl Pts',(6.03303673742344,25.0733905449905,-6.82454899803953));
#454905=CARTESIAN_POINT('Ctrl Pts',(6.84208605608162,25.0019074742962,-5.97347744575397));
#454906=CARTESIAN_POINT('Ctrl Pts',(6.56524194061871,24.9304244036021,-4.83231952202541));
#454907=CARTESIAN_POINT('Ctrl Pts',(5.45614521253248,24.8589413329078,-4.44658873189996));
#454908=CARTESIAN_POINT('Ctrl Pts',(4.53093499038958,24.7874582622137,-5.16968614336583));
#454909=CARTESIAN_POINT('Ctrl Pts',(4.63727615158268,24.7159751915195,-6.33911995340987));
#454910=CARTESIAN_POINT('Ctrl Pts',(5.67774038144015,24.6444921208254,-6.88347096747714));
#454911=CARTESIAN_POINT('Ctrl Pts',(6.69906868632339,24.5730090501312,-6.30401230613993));
#454912=CARTESIAN_POINT('Ctrl Pts',(6.76553413784902,24.501525979437,-5.1316360027112));
#454913=CARTESIAN_POINT('Ctrl Pts',(5.8162420056622,24.4300429087428,-4.4404570855349));
#454914=CARTESIAN_POINT('Ctrl Pts',(4.72092066657002,24.3585598380486,-4.86372415598114));
#454915=CARTESIAN_POINT('Ctrl Pts',(4.48308844595715,24.2870767673545,-6.01364575549065));
#454916=CARTESIAN_POINT('Ctrl Pts',(5.32064394905434,24.2155936966602,-6.83667955068161));
#454917=CARTESIAN_POINT('Ctrl Pts',(6.46623035855224,24.1441106259661,-6.57877331548262));
#454918=CARTESIAN_POINT('Ctrl Pts',(6.87027718549015,24.0726275552719,-5.4762171877825));
#454919=CARTESIAN_POINT('Ctrl Pts',(6.16260228864267,24.0011444845778,-4.5391579116818));
#454920=CARTESIAN_POINT('Ctrl Pts',(4.99156766820889,23.9296614138835,-4.62611628030964));
#454921=CARTESIAN_POINT('Ctrl Pts',(4.43005910275823,23.8581783431894,-5.65742225312448));
#454922=CARTESIAN_POINT('Ctrl Pts',(4.99252303072782,23.7866952724952,-6.68820746419386));
#454923=CARTESIAN_POINT('Ctrl Pts',(6.16363770038041,23.715212201801,-6.77408077335862));
#454924=CARTESIAN_POINT('Ctrl Pts',(6.87044407409259,23.6437291311068,-5.83636609328009));
#454925=CARTESIAN_POINT('Ctrl Pts',(6.46537570391973,23.5722460604127,-4.73418498174874));
#454926=CARTESIAN_POINT('Ctrl Pts',(5.31955101057097,23.5007629897185,-4.47734003862102));
#454927=CARTESIAN_POINT('Ctrl Pts',(4.48275809327536,23.4292799190243,-5.30115015081045));
#454928=CARTESIAN_POINT('Ctrl Pts',(4.72165647802515,23.3577968483301,-6.4508497069919));
#454929=CARTESIAN_POINT('Ctrl Pts',(5.81736804855842,23.286313777636,-6.8731039905307));
#454930=CARTESIAN_POINT('Ctrl Pts',(6.76602226241636,23.2148307069418,-6.18104124059857));
#454931=CARTESIAN_POINT('Ctrl Pts',(6.69846478576951,23.1433476362476,-5.00873590166638));
#454932=CARTESIAN_POINT('Ctrl Pts',(5.67661126055156,23.0718645655534,-4.43020643614536));
#454933=CARTESIAN_POINT('Ctrl Pts',(4.63662978245479,23.0003814948593,-4.97555543184771));
#454934=CARTESIAN_POINT('Ctrl Pts',(4.5314155623581,22.9288984241651,-6.1450203373264));
#454935=CARTESIAN_POINT('Ctrl Pts',(5.45721045950911,22.8574153534709,-6.86739142284001));
#454936=CARTESIAN_POINT('Ctrl Pts',(6.56611594115257,22.7859322827767,-6.48037563201499));
#454937=CARTESIAN_POINT('Ctrl Pts',(6.84157504188551,22.7144492120825,-5.33946716650399));
#454938=CARTESIAN_POINT('Ctrl Pts',(6.0323875407531,22.6429661413884,-4.48814850723257));
#454939=CARTESIAN_POINT('Ctrl Pts',(4.87752780133468,22.5714830706942,-4.70999101793355));
#454940=CARTESIAN_POINT('Ctrl Pts',(4.58641880376449,22.5238276902314,-5.4325862664886));
#454941=CARTESIAN_POINT('Ctrl Pts',(4.62591736201901,22.5,-5.7755760807344));
#454942=CARTESIAN_POINT('Ctrl Pts',(4.92443355077908,25.6019615242271,-6.39006796800885));
#454943=CARTESIAN_POINT('Ctrl Pts',(5.02053320993752,25.5925650294346,-6.48712194011206));
#454944=CARTESIAN_POINT('Ctrl Pts',(5.13467106978717,25.5831685346421,-6.56580235206401));
#454945=CARTESIAN_POINT('Ctrl Pts',(5.25993281439039,25.5737720398497,-6.617556583841));
#454946=CARTESIAN_POINT('Ctrl Pts',(5.57757232935518,25.5499443496183,-6.74879528829216));
#454947=CARTESIAN_POINT('Ctrl Pts',(5.96674190886751,25.5261166593869,-6.70689021711105));
#454948=CARTESIAN_POINT('Ctrl Pts',(6.24916768313609,25.5022889691555,-6.51104990542648));
#454949=CARTESIAN_POINT('Ctrl Pts',(6.53159345740467,25.4784612789241,-6.31520959374192));
#454950=CARTESIAN_POINT('Ctrl Pts',(6.7072754264295,25.4546335886927,-5.96543404155392));
#454951=CARTESIAN_POINT('Ctrl Pts',(6.69573385251462,25.4308058984613,-5.62194684521822));
#454952=CARTESIAN_POINT('Ctrl Pts',(6.68419227859974,25.4069782082299,-5.27845964888252));
#454953=CARTESIAN_POINT('Ctrl Pts',(6.48542716174514,25.3831505179985,-4.94126080839914));
#454954=CARTESIAN_POINT('Ctrl Pts',(6.19049196225387,25.3593228277671,-4.76482193949513));
#454955=CARTESIAN_POINT('Ctrl Pts',(5.89555676276259,25.3354951375357,-4.58838307059113));
#454956=CARTESIAN_POINT('Ctrl Pts',(5.50445148063464,25.3116674473043,-4.5727041732665));
#454957=CARTESIAN_POINT('Ctrl Pts',(5.19633848255872,25.2878397570729,-4.72496603669335));
#454958=CARTESIAN_POINT('Ctrl Pts',(4.8882254844828,25.2640120668416,-4.87722790012021));
#454959=CARTESIAN_POINT('Ctrl Pts',(4.6631047704589,25.2401843766102,-5.19743052429855));
#454960=CARTESIAN_POINT('Ctrl Pts',(4.62410272688105,25.2163566863788,-5.53889211090841));
#454961=CARTESIAN_POINT('Ctrl Pts',(4.58896793348097,25.1948916323282,-5.84649605160076));
#454962=CARTESIAN_POINT('Ctrl Pts',(4.70487246063661,25.1734265782776,-6.17135209942283));
#454963=CARTESIAN_POINT('Ctrl Pts',(4.92254817630007,25.1519615242271,-6.39198798715976));
#454964=CARTESIAN_POINT('Origin',(5.65685387860011,26.,-5.65685387860012));
#459211=UNCERTAINTY_MEASURE_WITH_UNIT(LENGTH_MEASURE(0.01),#459243,
'DISTANCE_ACCURACY_VALUE',
'Maximum model space distance between geometric entities at asserted c
onnectivities');
#459216=UNCERTAINTY_MEASURE_WITH_UNIT(LENGTH_MEASURE(0.01),#459243,
'DISTANCE_ACCURACY_VALUE',
'Maximum model space distance between geometric entities at asserted c
onnectivities');
#459237=(
GEOMETRIC_REPRESENTATION_CONTEXT(3)
GLOBAL_UNCERTAINTY_ASSIGNED_CONTEXT((#459211))
GLOBAL_UNIT_ASSIGNED_CONTEXT((#459243,#459245,#459246))
REPRESENTATION_CONTEXT('','3D')
);
#459242=(
GEOMETRIC_REPRESENTATION_CONTEXT(3)
GLOBAL_UNCERTAINTY_ASSIGNED_CONTEXT((#459216))
GLOBAL_UNIT_ASSIGNED_CONTEXT((#459243,#459245,#459246))
REPRESENTATION_CONTEXT('','3D')
);
#459243=(
LENGTH_UNIT()
NAMED_UNIT(*)
SI_UNIT(.MILLI.,.METRE.)
);
#459245=(
NAMED_UNIT(*)
PLANE_ANGLE_UNIT()
SI_UNIT($,.RADIAN.)
);
#459246=(
NAMED_UNIT(*)
SI_UNIT($,.STERADIAN.)
SOLID_ANGLE_UNIT()
);
#459267=SHAPE_DEFINITION_REPRESENTATION(#459294,#459348);
#459294=PRODUCT_DEFINITION_SHAPE('',$,#459374);
#459348=SHAPE_REPRESENTATION('',(#105175),#459237);
#459353=PRODUCT_DEFINITION_CONTEXT('part definition',#459430,'design');
#459374=PRODUCT_DEFINITION('Hotend Heatsink','Hotend Heatsink',#459399,
#459353);
#459399=PRODUCT_DEFINITION_FORMATION('',$,#459452);
#459430=APPLICATION_CONTEXT(
'Core Data for Automotive Mechanical Design Process');
#459431=PRODUCT_CONTEXT('part definition',#459430,'mechanical');
#459452=PRODUCT('Hotend Heatsink','Hotend Heatsink',$,(#459431));
#459513=COLOUR_RGB('Sky Blue',0.24,0.69,0.87);
#459514=FILL_AREA_STYLE_COLOUR('',#459513);
#459515=FILL_AREA_STYLE('',(#459514));
#459516=SURFACE_STYLE_FILL_AREA(#459515);
#459517=SURFACE_SIDE_STYLE('',(#459516));
#459518=SURFACE_STYLE_USAGE(.BOTH.,#459517);
#459519=PRESENTATION_STYLE_ASSIGNMENT((#459518));
ENDSEC;
END-ISO-10303-21;
